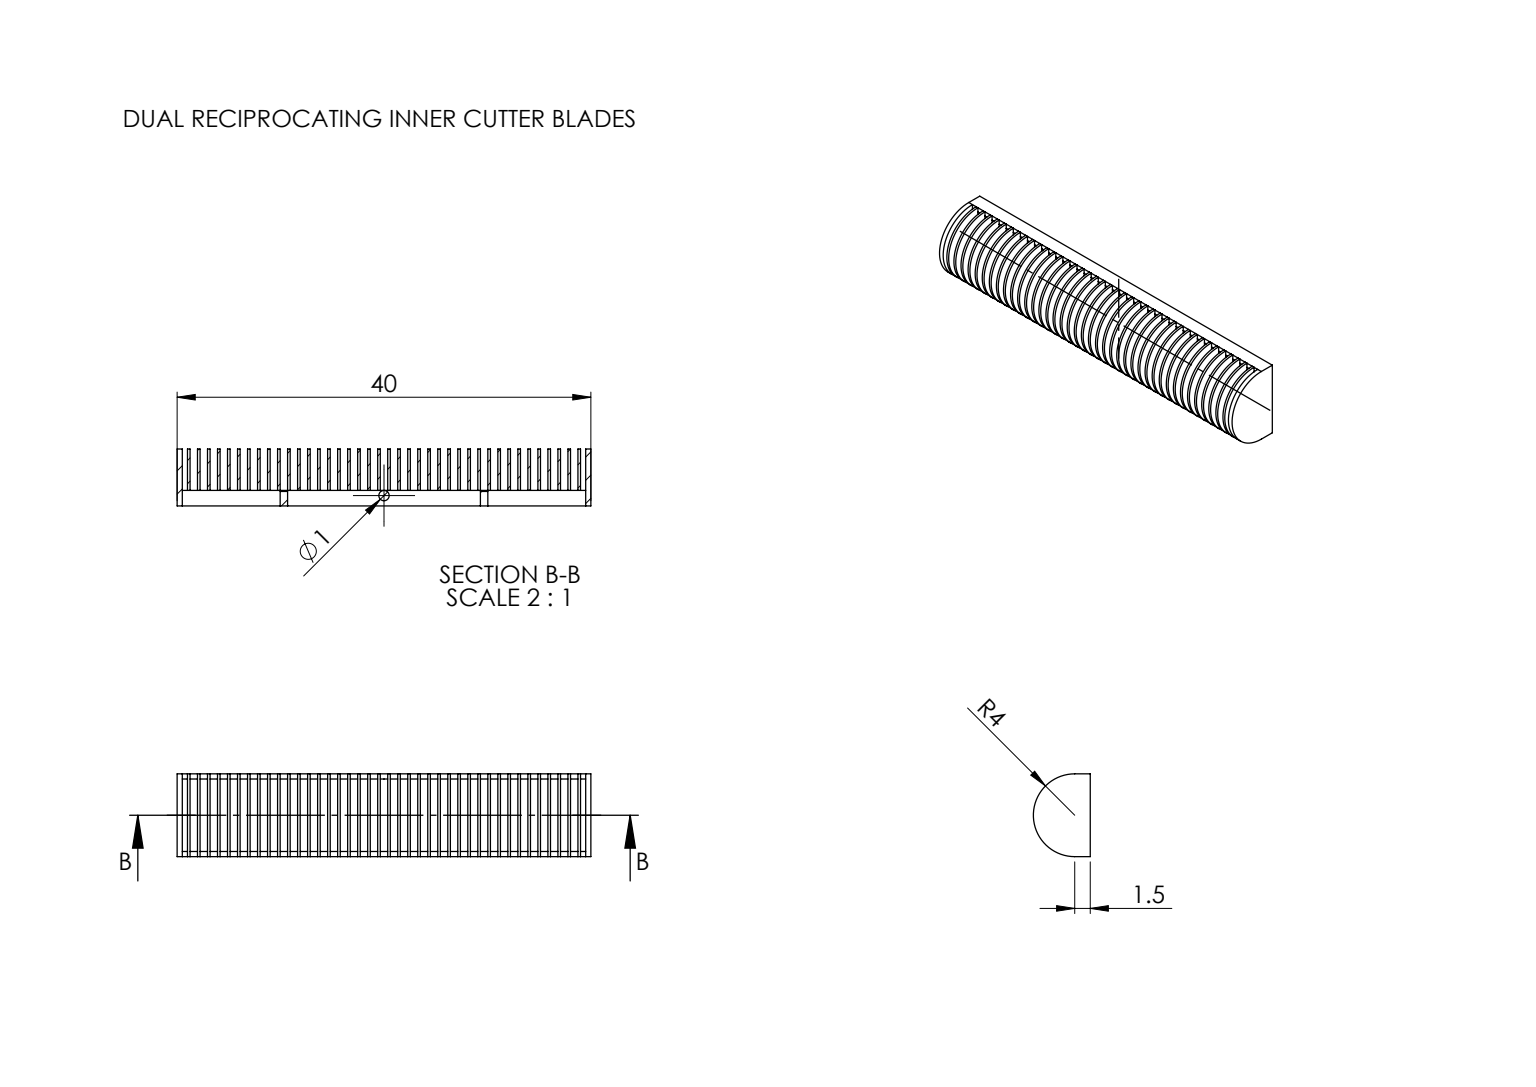
ISO-10303-21;
HEADER;
FILE_DESCRIPTION (('STEP AP214'),
    '1' );
FILE_NAME ('Dual Reciprocating Inner Cutter Blades.step',
    '2026-10-05T05:16:24',
    ( '' ),
    ( '' ),
    'SwSTEP 2.0',
    'SolidWorks 2026',
    '' );
FILE_SCHEMA (( 'AUTOMOTIVE_DESIGN' ));
ENDSEC;

DATA;
#43=ORIENTED_EDGE ( 'NONE', *, *, #10350, .F. ) ;
#63=CARTESIAN_POINT ( 'NONE',  ( -10.28846153846153832, -7.500000000000000000, 29.75000000000000355 ) ) ;
#66=ORIENTED_EDGE ( 'NONE', *, *, #42296, .F. ) ;
#80=EDGE_CURVE ( 'NONE', #19996, #25471, #12251, .T. ) ;
#85=CARTESIAN_POINT ( 'NONE',  ( -6.416666666666667851, -7.500000000000000000, 33.75000000000000000 ) ) ;
#89=ORIENTED_EDGE ( 'NONE', *, *, #31781, .F. ) ;
#103=EDGE_CURVE ( 'NONE', #84442, #3259, #72212, .T. ) ;
#104=VECTOR ( 'NONE', #2101, 1000.000000000000000 ) ;
#130=DIRECTION ( 'NONE',  ( -0.000000000000000000, 1.000000000000000000, -0.000000000000000000 ) ) ;
#140=CIRCLE ( 'NONE', #14540, 4.000000000000000000 ) ;
#156=CARTESIAN_POINT ( 'NONE',  ( 0.000000000000000000, -4.000000000000000000, 29.65000000000000213 ) ) ;
#169=ORIENTED_EDGE ( 'NONE', *, *, #57936, .F. ) ;
#181=ADVANCED_FACE ( 'NONE', ( #62640 ), #1839, .F. ) ;
#187=DIRECTION ( 'NONE',  ( -1.000000000000000000, -0.000000000000000000, -0.000000000000000000 ) ) ;
#201=EDGE_CURVE ( 'NONE', #75095, #37056, #56777, .T. ) ;
#227=DIRECTION ( 'NONE',  ( 1.000000000000000000, 0.000000000000000000, 0.000000000000000000 ) ) ;
#231=ORIENTED_EDGE ( 'NONE', *, *, #20585, .T. ) ;
#235=VERTEX_POINT ( 'NONE', #52679 ) ;
#282=EDGE_CURVE ( 'NONE', #18719, #16151, #10625, .T. ) ;
#284=CARTESIAN_POINT ( 'NONE',  ( -19.50000000000000000, -3.499999999999999556, 29.75000000000000355 ) ) ;
#286=CARTESIAN_POINT ( 'NONE',  ( 20.00000000000000000, -4.000000000000000000, 29.75000000000000355 ) ) ;
#293=DIRECTION ( 'NONE',  ( 0.000000000000000000, 0.000000000000000000, -1.000000000000000000 ) ) ;
#298=VECTOR ( 'NONE', #58906, 1000.000000000000000 ) ;
#299=ORIENTED_EDGE ( 'NONE', *, *, #31219, .F. ) ;
#325=VECTOR ( 'NONE', #40257, 1000.000000000000000 ) ;
#332=VECTOR ( 'NONE', #25563, 1000.000000000000000 ) ;
#345=VERTEX_POINT ( 'NONE', #74747 ) ;
#351=DIRECTION ( 'NONE',  ( -1.000000000000000000, -0.000000000000000000, -0.000000000000000000 ) ) ;
#357=FACE_OUTER_BOUND ( 'NONE', #7317, .T. ) ;
#362=CARTESIAN_POINT ( 'NONE',  ( 5.198717948717946236, -4.000000000000000000, 29.75000000000000355 ) ) ;
#377=ADVANCED_FACE ( 'NONE', ( #29653 ), #76057, .T. ) ;
#393=EDGE_CURVE ( 'NONE', #23382, #20924, #8053, .T. ) ;
#417=DIRECTION ( 'NONE',  ( 1.000000000000000000, 0.000000000000000000, 0.000000000000000000 ) ) ;
#418=CARTESIAN_POINT ( 'NONE',  ( -16.81410256410256565, -11.50000000000000000, 29.75000000000000355 ) ) ;
#426=COLOUR_RGB ( '', 0.72549020, 0.75294118, 0.79215686) ;
#427=VERTEX_POINT ( 'NONE', #8497 ) ;
#455=LINE ( 'NONE', #48625, #11505 ) ;
#469=CARTESIAN_POINT ( 'NONE',  ( 8.102564102564102200, -11.00000000000000000, 29.75000000000000355 ) ) ;
#496=VERTEX_POINT ( 'NONE', #69311 ) ;
#498=FACE_OUTER_BOUND ( 'NONE', #59189, .T. ) ;
#499=EDGE_LOOP ( 'NONE', ( #8065, #69891, #54153, #58268 ) ) ;
#505=ADVANCED_FACE ( 'NONE', ( #65191 ), #59330, .F. ) ;
#525=AXIS2_PLACEMENT_3D ( 'NONE', #7311, #6858, #76199 ) ;
#528=CARTESIAN_POINT ( 'NONE',  ( -3.262820512820514107, -7.500000000000000000, 29.75000000000000355 ) ) ;
#532=ORIENTED_EDGE ( 'NONE', *, *, #45439, .F. ) ;
#537=LINE ( 'NONE', #63557, #72302 ) ;
#544=CIRCLE ( 'NONE', #45150, 4.000000000000000000 ) ;
#548=DIRECTION ( 'NONE',  ( -0.000000000000000000, 1.000000000000000000, -0.000000000000000000 ) ) ;
#550=VECTOR ( 'NONE', #21356, 1000.000000000000000 ) ;
#573=CARTESIAN_POINT ( 'NONE',  ( 20.00000000000000000, -4.000000000000000000, 29.75000000000000355 ) ) ;
#598=DIRECTION ( 'NONE',  ( 0.000000000000000000, -0.000000000000000000, 1.000000000000000000 ) ) ;
#619=ORIENTED_EDGE ( 'NONE', *, *, #51470, .F. ) ;
#634=DIRECTION ( 'NONE',  ( 1.000000000000000000, 0.000000000000000000, 0.000000000000000000 ) ) ;
#641=CARTESIAN_POINT ( 'NONE',  ( 20.00000000000000000, -4.000000000000000000, 29.75000000000000355 ) ) ;
#681=ORIENTED_EDGE ( 'NONE', *, *, #24672, .T. ) ;
#686=DIRECTION ( 'NONE',  ( -0.000000000000000000, 1.000000000000000000, -0.000000000000000000 ) ) ;
#691=PLANE ( 'NONE',  #60122 ) ;
#695=VECTOR ( 'NONE', #44680, 1000.000000000000000 ) ;
#706=CARTESIAN_POINT ( 'NONE',  ( 3.512820512820510555, -3.499999999999999556, 29.75000000000000355 ) ) ;
#723=DIRECTION ( 'NONE',  ( 1.000000000000000000, 0.000000000000000000, 0.000000000000000000 ) ) ;
#756=LINE ( 'NONE', #28222, #84616 ) ;
#774=ORIENTED_EDGE ( 'NONE', *, *, #775, .F. ) ;
#775=EDGE_CURVE ( 'NONE', #46484, #84195, #71288, .T. ) ;
#780=ORIENTED_EDGE ( 'NONE', *, *, #80659, .F. ) ;
#792=CARTESIAN_POINT ( 'NONE',  ( -18.75000000000000000, -4.000000000000000000, 29.75000000000000355 ) ) ;
#811=DIRECTION ( 'NONE',  ( 1.000000000000000000, 0.000000000000000000, 0.000000000000000000 ) ) ;
#823=EDGE_CURVE ( 'NONE', #22055, #5633, #71733, .T. ) ;
#832=CARTESIAN_POINT ( 'NONE',  ( 16.81410256410256565, -3.499999999999999556, 29.75000000000000355 ) ) ;
#838=CARTESIAN_POINT ( 'NONE',  ( -17.78205128205128105, -3.499999999999999556, 29.75000000000000355 ) ) ;
#851=CARTESIAN_POINT ( 'NONE',  ( 20.00000000000000000, -3.499999999999999556, 29.75000000000000355 ) ) ;
#856=VERTEX_POINT ( 'NONE', #42182 ) ;
#857=LINE ( 'NONE', #49041, #17570 ) ;
#859=LINE ( 'NONE', #33327, #83953 ) ;
#860=LINE ( 'NONE', #69327, #48492 ) ;
#866=EDGE_CURVE ( 'NONE', #87922, #72293, #29882, .T. ) ;
#882=VECTOR ( 'NONE', #7598, 1000.000000000000000 ) ;
#885=ORIENTED_EDGE ( 'NONE', *, *, #13025, .T. ) ;
#909=CARTESIAN_POINT ( 'NONE',  ( -5.198717948717948012, -7.500000000000000000, 33.75000000000000000 ) ) ;
#923=ADVANCED_BREP_SHAPE_REPRESENTATION ( '', ( #28293, #83448 ), #70522 ) ;
#938=DIRECTION ( 'NONE',  ( 0.000000000000000000, 0.000000000000000000, -1.000000000000000000 ) ) ;
#940=CYLINDRICAL_SURFACE ( 'NONE', #5295, 4.000000000000000000 ) ;
#949=VERTEX_POINT ( 'NONE', #24881 ) ;
#955=VERTEX_POINT ( 'NONE', #59557 ) ;
#959=AXIS2_PLACEMENT_3D ( 'NONE', #1082, #49271, #73543 ) ;
#965=VECTOR ( 'NONE', #65719, 1000.000000000000000 ) ;
#972=DIRECTION ( 'NONE',  ( -0.000000000000000000, 1.000000000000000000, -0.000000000000000000 ) ) ;
#981=CARTESIAN_POINT ( 'NONE',  ( -10.03846153846153832, -4.000000000000000000, 29.25000000000000000 ) ) ;
#985=ORIENTED_EDGE ( 'NONE', *, *, #59724, .T. ) ;
#987=EDGE_LOOP ( 'NONE', ( #37352, #22515, #57564, #42926 ) ) ;
#992=VECTOR ( 'NONE', #4402, 1000.000000000000000 ) ;
#993=FACE_OUTER_BOUND ( 'NONE', #69056, .T. ) ;
#1006=CARTESIAN_POINT ( 'NONE',  ( -4.480769230769229061, -4.000000000000000000, 29.75000000000000355 ) ) ;
#1012=VERTEX_POINT ( 'NONE', #48701 ) ;
#1029=ORIENTED_EDGE ( 'NONE', *, *, #8831, .T. ) ;
#1031=ADVANCED_FACE ( 'NONE', ( #5959 ), #53690, .T. ) ;
#1036=DIRECTION ( 'NONE',  ( 0.000000000000000000, 0.000000000000000000, -1.000000000000000000 ) ) ;
#1051=VECTOR ( 'NONE', #75352, 1000.000000000000000 ) ;
#1057=EDGE_LOOP ( 'NONE', ( #1568, #37917, #18646, #65919 ) ) ;
#1082=CARTESIAN_POINT ( 'NONE',  ( -16.81410256410256565, -7.500000000000000000, 29.75000000000000355 ) ) ;
#1092=ORIENTED_EDGE ( 'NONE', *, *, #823, .F. ) ;
#1103=EDGE_CURVE ( 'NONE', #81224, #48029, #68558, .T. ) ;
#1133=DIRECTION ( 'NONE',  ( 0.000000000000000000, 0.000000000000000000, 1.000000000000000000 ) ) ;
#1148=VECTOR ( 'NONE', #38524, 1000.000000000000000 ) ;
#1206=ORIENTED_EDGE ( 'NONE', *, *, #30331, .F. ) ;
#1231=DIRECTION ( 'NONE',  ( 0.000000000000000000, 0.000000000000000000, -1.000000000000000000 ) ) ;
#1250=CARTESIAN_POINT ( 'NONE',  ( 20.00000000000000000, -4.000000000000000000, 29.75000000000000355 ) ) ;
#1268=CARTESIAN_POINT ( 'NONE',  ( 6.416666666666664298, -11.50000000000000000, 29.75000000000000355 ) ) ;
#1284=ORIENTED_EDGE ( 'NONE', *, *, #40773, .F. ) ;
#1327=AXIS2_PLACEMENT_3D ( 'NONE', #67691, #28352, #40223 ) ;
#1331=AXIS2_PLACEMENT_3D ( 'NONE', #28757, #51198, #49466 ) ;
#1333=VERTEX_POINT ( 'NONE', #30644 ) ;
#1374=FACE_OUTER_BOUND ( 'NONE', #33214, .T. ) ;
#1386=PLANE ( 'NONE',  #17654 ) ;
#1393=AXIS2_PLACEMENT_3D ( 'NONE', #18730, #59256, #59702 ) ;
#1395=DIRECTION ( 'NONE',  ( 1.000000000000000000, 0.000000000000000000, 0.000000000000000000 ) ) ;
#1397=DIRECTION ( 'NONE',  ( -1.000000000000000000, -0.000000000000000000, 0.000000000000000000 ) ) ;
#1401=VECTOR ( 'NONE', #24481, 1000.000000000000000 ) ;
#1405=AXIS2_PLACEMENT_3D ( 'NONE', #11950, #31322, #53361 ) ;
#1406=ORIENTED_EDGE ( 'NONE', *, *, #78616, .F. ) ;
#1415=CARTESIAN_POINT ( 'NONE',  ( -0.6089743589743593644, -3.499999999999999556, 29.75000000000000355 ) ) ;
#1428=ORIENTED_EDGE ( 'NONE', *, *, #57736, .F. ) ;
#1434=EDGE_CURVE ( 'NONE', #50542, #83291, #88729, .T. ) ;
#1450=AXIS2_PLACEMENT_3D ( 'NONE', #52880, #24518, #79482 ) ;
#1456=ORIENTED_EDGE ( 'NONE', *, *, #88867, .T. ) ;
#1473=ORIENTED_EDGE ( 'NONE', *, *, #63442, .F. ) ;
#1490=CARTESIAN_POINT ( 'NONE',  ( -18.03205128205128105, -3.499999999999999556, 29.75000000000000355 ) ) ;
#1493=VERTEX_POINT ( 'NONE', #21123 ) ;
#1495=DIRECTION ( 'NONE',  ( -1.000000000000000000, -0.000000000000000000, -0.000000000000000000 ) ) ;
#1501=ADVANCED_FACE ( 'NONE', ( #63440 ), #77841, .F. ) ;
#1503=VECTOR ( 'NONE', #30513, 1000.000000000000000 ) ;
#1506=FACE_OUTER_BOUND ( 'NONE', #62728, .T. ) ;
#1517=EDGE_CURVE ( 'NONE', #55049, #67618, #860, .T. ) ;
#1526=ORIENTED_EDGE ( 'NONE', *, *, #34553, .F. ) ;
#1553=EDGE_CURVE ( 'NONE', #78266, #17849, #49497, .T. ) ;
#1559=ORIENTED_EDGE ( 'NONE', *, *, #71272, .T. ) ;
#1565=DIRECTION ( 'NONE',  ( 0.000000000000000000, 0.000000000000000000, -1.000000000000000000 ) ) ;
#1568=ORIENTED_EDGE ( 'NONE', *, *, #54155, .F. ) ;
#1572=EDGE_CURVE ( 'NONE', #20924, #27696, #5306, .T. ) ;
#1576=VECTOR ( 'NONE', #71122, 1000.000000000000000 ) ;
#1582=DIRECTION ( 'NONE',  ( -1.000000000000000000, -0.000000000000000000, -0.000000000000000000 ) ) ;
#1583=DIRECTION ( 'NONE',  ( 0.000000000000000000, 0.000000000000000000, -1.000000000000000000 ) ) ;
#1584=DIRECTION ( 'NONE',  ( -0.000000000000000000, 0.000000000000000000, 1.000000000000000000 ) ) ;
#1587=VECTOR ( 'NONE', #24500, 1000.000000000000000 ) ;
#1614=EDGE_CURVE ( 'NONE', #32479, #19139, #52139, .T. ) ;
#1627=VECTOR ( 'NONE', #61858, 1000.000000000000000 ) ;
#1652=VERTEX_POINT ( 'NONE', #78732 ) ;
#1654=ORIENTED_EDGE ( 'NONE', *, *, #27147, .T. ) ;
#1664=ORIENTED_EDGE ( 'NONE', *, *, #70919, .F. ) ;
#1669=DIRECTION ( 'NONE',  ( 1.000000000000000000, 0.000000000000000000, 0.000000000000000000 ) ) ;
#1679=EDGE_CURVE ( 'NONE', #34673, #24943, #58899, .T. ) ;
#1682=CARTESIAN_POINT ( 'NONE',  ( -2.294871794871794712, -11.00000000000000000, 29.75000000000000355 ) ) ;
#1708=ORIENTED_EDGE ( 'NONE', *, *, #14428, .T. ) ;
#1731=CARTESIAN_POINT ( 'NONE',  ( 14.16025641025641235, -3.499999999999999556, 29.75000000000000355 ) ) ;
#1733=DIRECTION ( 'NONE',  ( 0.000000000000000000, 0.000000000000000000, -1.000000000000000000 ) ) ;
#1734=FACE_OUTER_BOUND ( 'NONE', #71110, .T. ) ;
#1747=ORIENTED_EDGE ( 'NONE', *, *, #24136, .F. ) ;
#1752=PLANE ( 'NONE',  #35748 ) ;
#1759=CARTESIAN_POINT ( 'NONE',  ( 18.75000000000000000, -4.000000000000000000, 29.75000000000000355 ) ) ;
#1774=PLANE ( 'NONE',  #72639 ) ;
#1775=ORIENTED_EDGE ( 'NONE', *, *, #3712, .T. ) ;
#1813=DIRECTION ( 'NONE',  ( -0.000000000000000000, 1.000000000000000000, -0.000000000000000000 ) ) ;
#1829=EDGE_CURVE ( 'NONE', #64127, #48416, #12500, .T. ) ;
#1832=DIRECTION ( 'NONE',  ( -1.000000000000000000, -0.000000000000000000, -0.000000000000000000 ) ) ;
#1839=PLANE ( 'NONE',  #51896 ) ;
#1856=LINE ( 'NONE', #63987, #27063 ) ;
#1861=DIRECTION ( 'NONE',  ( -0.000000000000000000, 1.000000000000000000, -0.000000000000000000 ) ) ;
#1863=VECTOR ( 'NONE', #23258, 1000.000000000000000 ) ;
#1865=CARTESIAN_POINT ( 'NONE',  ( -13.91025641025641058, -11.50000000000000000, 29.75000000000000355 ) ) ;
#1877=ADVANCED_FACE ( 'NONE', ( #25410 ), #51976, .F. ) ;
#1878=VERTEX_POINT ( 'NONE', #66841 ) ;
#1892=DIRECTION ( 'NONE',  ( -1.000000000000000000, 0.000000000000000000, -0.000000000000000000 ) ) ;
#1898=CARTESIAN_POINT ( 'NONE',  ( -3.262820512820514107, -7.500000000000000000, 33.75000000000000000 ) ) ;
#1908=ADVANCED_FACE ( 'NONE', ( #60074 ), #86239, .F. ) ;
#1926=VECTOR ( 'NONE', #72975, 1000.000000000000000 ) ;
#1944=DIRECTION ( 'NONE',  ( -1.000000000000000000, 0.000000000000000000, -0.000000000000000000 ) ) ;
#1957=CARTESIAN_POINT ( 'NONE',  ( 7.384615384615385025, -3.499999999999999556, 29.75000000000000355 ) ) ;
#1964=CIRCLE ( 'NONE', #52285, 4.000000000000000000 ) ;
#1970=EDGE_CURVE ( 'NONE', #30104, #87793, #20865, .T. ) ;
#1972=EDGE_LOOP ( 'NONE', ( #51803, #60788, #41402, #7362 ) ) ;
#1980=EDGE_CURVE ( 'NONE', #55785, #38648, #82590, .T. ) ;
#1992=ORIENTED_EDGE ( 'NONE', *, *, #87731, .T. ) ;
#2027=CARTESIAN_POINT ( 'NONE',  ( -5.198717948717948012, -7.500000000000000000, 33.75000000000000000 ) ) ;
#2070=CARTESIAN_POINT ( 'NONE',  ( -19.50000000000000000, -3.499999999999999556, 29.75000000000000355 ) ) ;
#2085=VERTEX_POINT ( 'NONE', #74740 ) ;
#2092=CARTESIAN_POINT ( 'NONE',  ( -19.00000000000000000, -7.500000000000000000, 29.75000000000000355 ) ) ;
#2095=ORIENTED_EDGE ( 'NONE', *, *, #39042, .F. ) ;
#2101=DIRECTION ( 'NONE',  ( -1.000000000000000000, -0.000000000000000000, 0.000000000000000000 ) ) ;
#2116=CARTESIAN_POINT ( 'NONE',  ( 0.3589743589743582541, -7.500000000000000000, 29.75000000000000355 ) ) ;
#2121=CARTESIAN_POINT ( 'NONE',  ( 20.00000000000000000, -4.000000000000000000, 29.75000000000000355 ) ) ;
#2125=ORIENTED_EDGE ( 'NONE', *, *, #16712, .F. ) ;
#2144=FACE_OUTER_BOUND ( 'NONE', #19220, .T. ) ;
#2160=ORIENTED_EDGE ( 'NONE', *, *, #26803, .T. ) ;
#2174=VECTOR ( 'NONE', #49018, 1000.000000000000000 ) ;
#2177=ORIENTED_EDGE ( 'NONE', *, *, #59364, .T. ) ;
#2183=ORIENTED_EDGE ( 'NONE', *, *, #14015, .F. ) ;
#2191=ADVANCED_FACE ( 'NONE', ( #48569 ), #76050, .F. ) ;
#2194=ORIENTED_EDGE ( 'NONE', *, *, #21005, .T. ) ;
#2199=AXIS2_PLACEMENT_3D ( 'NONE', #14959, #44167, #77095 ) ;
#2212=CARTESIAN_POINT ( 'NONE',  ( -18.75000000000000000, -11.50000000000000000, 29.75000000000000355 ) ) ;
#2225=LINE ( 'NONE', #55849, #67827 ) ;
#2235=CARTESIAN_POINT ( 'NONE',  ( 20.00000000000000000, -4.000000000000000000, 29.75000000000000355 ) ) ;
#2237=EDGE_LOOP ( 'NONE', ( #84036, #26205, #82453, #32891, #73664 ) ) ;
#2248=CARTESIAN_POINT ( 'NONE',  ( 1.326923076923075762, -11.00000000000000000, 29.75000000000000355 ) ) ;
#2256=AXIS2_PLACEMENT_3D ( 'NONE', #9773, #56636, #71466 ) ;
#2258=FACE_OUTER_BOUND ( 'NONE', #13603, .T. ) ;
#2269=CIRCLE ( 'NONE', #6595, 4.000000000000000000 ) ;
#2279=ORIENTED_EDGE ( 'NONE', *, *, #42735, .T. ) ;
#2287=EDGE_CURVE ( 'NONE', #23070, #235, #14045, .T. ) ;
#2291=VECTOR ( 'NONE', #33549, 1000.000000000000000 ) ;
#2293=LINE ( 'NONE', #22141, #25357 ) ;
#2307=ORIENTED_EDGE ( 'NONE', *, *, #76762, .T. ) ;
#2311=DIRECTION ( 'NONE',  ( -0.000000000000000000, 1.000000000000000000, -0.000000000000000000 ) ) ;
#2319=ADVANCED_FACE ( 'NONE', ( #77380 ), #23751, .F. ) ;
#2322=ORIENTED_EDGE ( 'NONE', *, *, #44361, .F. ) ;
#2351=EDGE_LOOP ( 'NONE', ( #79932, #72056, #42009, #57754 ) ) ;
#2360=EDGE_CURVE ( 'NONE', #29827, #86419, #51204, .T. ) ;
#2362=CYLINDRICAL_SURFACE ( 'NONE', #36184, 4.000000000000000000 ) ;
#2382=CIRCLE ( 'NONE', #15324, 4.000000000000000000 ) ;
#2392=VERTEX_POINT ( 'NONE', #78711 ) ;
#2421=VECTOR ( 'NONE', #3040, 1000.000000000000000 ) ;
#2425=EDGE_CURVE ( 'NONE', #48052, #5633, #24651, .T. ) ;
#2432=ORIENTED_EDGE ( 'NONE', *, *, #24288, .T. ) ;
#2434=ORIENTED_EDGE ( 'NONE', *, *, #22837, .T. ) ;
#2437=VECTOR ( 'NONE', #87966, 1000.000000000000000 ) ;
#2441=ORIENTED_EDGE ( 'NONE', *, *, #7391, .T. ) ;
#2448=EDGE_CURVE ( 'NONE', #6548, #11602, #73751, .T. ) ;
#2467=DIRECTION ( 'NONE',  ( 1.000000000000000000, 0.000000000000000000, 0.000000000000000000 ) ) ;
#2502=EDGE_CURVE ( 'NONE', #24740, #74652, #52560, .T. ) ;
#2512=CARTESIAN_POINT ( 'NONE',  ( -13.91025641025641058, -3.499999999999999556, 29.75000000000000355 ) ) ;
#2513=AXIS2_PLACEMENT_3D ( 'NONE', #838, #35064, #62095 ) ;
#2519=ORIENTED_EDGE ( 'NONE', *, *, #20527, .F. ) ;
#2528=DIRECTION ( 'NONE',  ( 0.000000000000000000, 0.000000000000000000, 1.000000000000000000 ) ) ;
#2530=ORIENTED_EDGE ( 'NONE', *, *, #33972, .F. ) ;
#2538=CARTESIAN_POINT ( 'NONE',  ( -19.50000000000000000, -11.50000000000000000, 29.75000000000000355 ) ) ;
#2571=LINE ( 'NONE', #30063, #7312 ) ;
#2576=ADVANCED_FACE ( 'NONE', ( #36202 ), #69525, .F. ) ;
#2579=CARTESIAN_POINT ( 'NONE',  ( 12.94230769230769340, -3.499999999999999556, 29.75000000000000355 ) ) ;
#2608=EDGE_CURVE ( 'NONE', #80662, #81634, #61100, .T. ) ;
#2616=CIRCLE ( 'NONE', #27123, 4.000000000000000000 ) ;
#2620=ADVANCED_FACE ( 'NONE', ( #9587 ), #58213, .F. ) ;
#2623=FACE_OUTER_BOUND ( 'NONE', #72608, .T. ) ;
#2631=EDGE_CURVE ( 'NONE', #35283, #64127, #30743, .T. ) ;
#2662=AXIS2_PLACEMENT_3D ( 'NONE', #67394, #47108, #27293 ) ;
#2667=ORIENTED_EDGE ( 'NONE', *, *, #61590, .F. ) ;
#2668=DIRECTION ( 'NONE',  ( 0.000000000000000000, 1.000000000000000000, 0.000000000000000000 ) ) ;
#2672=LINE ( 'NONE', #2235, #40622 ) ;
#2678=ORIENTED_EDGE ( 'NONE', *, *, #36115, .T. ) ;
#2680=EDGE_CURVE ( 'NONE', #74021, #13621, #37497, .T. ) ;
#2716=EDGE_CURVE ( 'NONE', #53841, #77088, #5511, .T. ) ;
#2724=ORIENTED_EDGE ( 'NONE', *, *, #51536, .T. ) ;
#2725=VECTOR ( 'NONE', #47467, 1000.000000000000000 ) ;
#2742=ORIENTED_EDGE ( 'NONE', *, *, #79560, .T. ) ;
#2763=DIRECTION ( 'NONE',  ( -1.000000000000000000, -0.000000000000000000, -0.000000000000000000 ) ) ;
#2781=VECTOR ( 'NONE', #43857, 1000.000000000000000 ) ;
#2792=VECTOR ( 'NONE', #5260, 1000.000000000000000 ) ;
#2796=AXIS2_PLACEMENT_3D ( 'NONE', #85379, #21900, #44364 ) ;
#2827=VECTOR ( 'NONE', #8252, 1000.000000000000000 ) ;
#2828=ORIENTED_EDGE ( 'NONE', *, *, #53808, .F. ) ;
#2843=VERTEX_POINT ( 'NONE', #20356 ) ;
#2852=VECTOR ( 'NONE', #1832, 1000.000000000000000 ) ;
#2853=CIRCLE ( 'NONE', #11558, 4.000000000000000000 ) ;
#2855=ORIENTED_EDGE ( 'NONE', *, *, #6324, .T. ) ;
#2867=EDGE_CURVE ( 'NONE', #38648, #58158, #59998, .T. ) ;
#2869=CARTESIAN_POINT ( 'NONE',  ( 17.78205128205128105, -3.499999999999999556, 29.75000000000000355 ) ) ;
#2890=EDGE_CURVE ( 'NONE', #10355, #2843, #41066, .T. ) ;
#2904=EDGE_CURVE ( 'NONE', #35531, #86970, #68527, .T. ) ;
#2908=DIRECTION ( 'NONE',  ( 0.000000000000000000, 0.000000000000000000, -1.000000000000000000 ) ) ;
#2913=VECTOR ( 'NONE', #79043, 1000.000000000000000 ) ;
#2915=ADVANCED_FACE ( 'NONE', ( #46489 ), #73967, .F. ) ;
#2928=AXIS2_PLACEMENT_3D ( 'NONE', #34029, #20950, #48421 ) ;
#2966=VECTOR ( 'NONE', #38248, 1000.000000000000000 ) ;
#2972=AXIS2_PLACEMENT_3D ( 'NONE', #41805, #26956, #54413 ) ;
#2979=VECTOR ( 'NONE', #40702, 1000.000000000000000 ) ;
#3004=CARTESIAN_POINT ( 'NONE',  ( 5.448717948717947124, -7.500000000000000000, 29.75000000000000355 ) ) ;
#3029=CARTESIAN_POINT ( 'NONE',  ( 18.03205128205128105, -11.00000000000000000, 29.75000000000000355 ) ) ;
#3040=DIRECTION ( 'NONE',  ( -1.000000000000000000, -0.000000000000000000, -0.000000000000000000 ) ) ;
#3044=VECTOR ( 'NONE', #84328, 1000.000000000000000 ) ;
#3048=DIRECTION ( 'NONE',  ( 1.000000000000000000, 0.000000000000000000, 0.000000000000000000 ) ) ;
#3060=CARTESIAN_POINT ( 'NONE',  ( -19.50000000000000000, -3.499999999999999556, 29.75000000000000355 ) ) ;
#3074=ORIENTED_EDGE ( 'NONE', *, *, #10327, .F. ) ;
#3077=AXIS2_PLACEMENT_3D ( 'NONE', #88927, #42055, #49246 ) ;
#3084=EDGE_CURVE ( 'NONE', #22055, #74851, #83095, .T. ) ;
#3089=CARTESIAN_POINT ( 'NONE',  ( -10.03846153846153832, -3.499999999999999556, 29.75000000000000355 ) ) ;
#3091=ORIENTED_EDGE ( 'NONE', *, *, #14653, .T. ) ;
#3093=CARTESIAN_POINT ( 'NONE',  ( -8.102564102564102200, -7.500000000000000000, 29.75000000000000355 ) ) ;
#3095=CARTESIAN_POINT ( 'NONE',  ( 16.09615384615384670, -3.499999999999999556, 29.75000000000000355 ) ) ;
#3099=VECTOR ( 'NONE', #55182, 1000.000000000000000 ) ;
#3102=LINE ( 'NONE', #10760, #1576 ) ;
#3118=CARTESIAN_POINT ( 'NONE',  ( -11.97435897435897267, -7.500000000000000000, 29.75000000000000355 ) ) ;
#3122=DIRECTION ( 'NONE',  ( 0.000000000000000000, 0.000000000000000000, -1.000000000000000000 ) ) ;
#3128=ORIENTED_EDGE ( 'NONE', *, *, #73177, .F. ) ;
#3154=EDGE_CURVE ( 'NONE', #43102, #76951, #87849, .T. ) ;
#3185=CIRCLE ( 'NONE', #19071, 4.000000000000000000 ) ;
#3188=LINE ( 'NONE', #65770, #78107 ) ;
#3195=ADVANCED_FACE ( 'NONE', ( #14824 ), #68425, .F. ) ;
#3208=VECTOR ( 'NONE', #88293, 1000.000000000000000 ) ;
#3212=CARTESIAN_POINT ( 'NONE',  ( -11.25641025641025550, -3.499999999999999556, 29.75000000000000355 ) ) ;
#3215=CARTESIAN_POINT ( 'NONE',  ( -19.50000000000000000, -3.499999999999999556, 29.75000000000000355 ) ) ;
#3235=ADVANCED_FACE ( 'NONE', ( #56246 ), #62541, .F. ) ;
#3251=ORIENTED_EDGE ( 'NONE', *, *, #79029, .T. ) ;
#3259=VERTEX_POINT ( 'NONE', #7619 ) ;
#3262=VERTEX_POINT ( 'NONE', #418 ) ;
#3275=DIRECTION ( 'NONE',  ( 0.000000000000000000, 0.000000000000000000, -1.000000000000000000 ) ) ;
#3292=VERTEX_POINT ( 'NONE', #27887 ) ;
#3294=ORIENTED_EDGE ( 'NONE', *, *, #55497, .F. ) ;
#3296=CIRCLE ( 'NONE', #66576, 4.000000000000000000 ) ;
#3302=EDGE_CURVE ( 'NONE', #5633, #496, #34222, .T. ) ;
#3303=FACE_OUTER_BOUND ( 'NONE', #83869, .T. ) ;
#3310=EDGE_LOOP ( 'NONE', ( #83643, #82972, #52409, #33244, #73566 ) ) ;
#3332=EDGE_CURVE ( 'NONE', #37853, #58001, #85933, .T. ) ;
#3340=DIRECTION ( 'NONE',  ( 0.000000000000000000, 0.000000000000000000, 1.000000000000000000 ) ) ;
#3356=CARTESIAN_POINT ( 'NONE',  ( 9.070512820512819374, -3.499999999999999556, 29.75000000000000355 ) ) ;
#3398=EDGE_CURVE ( 'NONE', #3876, #58816, #16576, .T. ) ;
#3414=VECTOR ( 'NONE', #68678, 1000.000000000000000 ) ;
#3438=ORIENTED_EDGE ( 'NONE', *, *, #30030, .T. ) ;
#3448=EDGE_CURVE ( 'NONE', #76927, #73366, #25114, .T. ) ;
#3488=AXIS2_PLACEMENT_3D ( 'NONE', #63887, #16156, #15722 ) ;
#3489=VECTOR ( 'NONE', #65292, 1000.000000000000000 ) ;
#3492=ORIENTED_EDGE ( 'NONE', *, *, #69496, .F. ) ;
#3497=CARTESIAN_POINT ( 'NONE',  ( -3.262820512820514107, -7.500000000000000000, 29.75000000000000355 ) ) ;
#3519=ORIENTED_EDGE ( 'NONE', *, *, #19505, .T. ) ;
#3529=VERTEX_POINT ( 'NONE', #52133 ) ;
#3563=DIRECTION ( 'NONE',  ( 0.000000000000000000, 0.000000000000000000, -1.000000000000000000 ) ) ;
#3593=DIRECTION ( 'NONE',  ( 0.000000000000000000, 0.000000000000000000, 1.000000000000000000 ) ) ;
#3624=VECTOR ( 'NONE', #69672, 1000.000000000000000 ) ;
#3628=CARTESIAN_POINT ( 'NONE',  ( 11.97435897435897623, -11.50000000000000000, 29.75000000000000355 ) ) ;
#3629=CARTESIAN_POINT ( 'NONE',  ( 20.00000000000000000, -4.000000000000000000, 29.75000000000000355 ) ) ;
#3633=VERTEX_POINT ( 'NONE', #7952 ) ;
#3634=CARTESIAN_POINT ( 'NONE',  ( -19.50000000000000000, -7.500000000000000000, 33.75000000000000000 ) ) ;
#3638=ORIENTED_EDGE ( 'NONE', *, *, #21291, .T. ) ;
#3647=EDGE_LOOP ( 'NONE', ( #62792, #87525, #25905, #75128, #60301 ) ) ;
#3664=CARTESIAN_POINT ( 'NONE',  ( -1.326923076923076872, -3.499999999999999556, 29.75000000000000355 ) ) ;
#3692=DIRECTION ( 'NONE',  ( 0.000000000000000000, 0.000000000000000000, -1.000000000000000000 ) ) ;
#3698=ORIENTED_EDGE ( 'NONE', *, *, #27739, .F. ) ;
#3701=CARTESIAN_POINT ( 'NONE',  ( 8.102564102564102200, -7.500000000000000000, 29.75000000000000355 ) ) ;
#3712=EDGE_CURVE ( 'NONE', #48041, #62888, #16477, .T. ) ;
#3724=ORIENTED_EDGE ( 'NONE', *, *, #22949, .T. ) ;
#3750=LINE ( 'NONE', #73105, #68099 ) ;
#3756=VERTEX_POINT ( 'NONE', #79520 ) ;
#3770=EDGE_CURVE ( 'NONE', #2392, #2085, #58787, .T. ) ;
#3773=DIRECTION ( 'NONE',  ( -0.000000000000000000, 1.000000000000000000, -0.000000000000000000 ) ) ;
#3778=DIRECTION ( 'NONE',  ( 1.000000000000000000, 0.000000000000000000, 0.000000000000000000 ) ) ;
#3789=CARTESIAN_POINT ( 'NONE',  ( 0.000000000000000000, -11.00000000000000000, 29.75000000000000355 ) ) ;
#3798=DIRECTION ( 'NONE',  ( 0.000000000000000000, 0.000000000000000000, -1.000000000000000000 ) ) ;
#3805=VECTOR ( 'NONE', #55218, 1000.000000000000000 ) ;
#3819=VECTOR ( 'NONE', #9595, 1000.000000000000000 ) ;
#3826=CARTESIAN_POINT ( 'NONE',  ( -3.512820512820513663, -3.499999999999999556, 29.75000000000000355 ) ) ;
#3834=EDGE_CURVE ( 'NONE', #29630, #74179, #48822, .T. ) ;
#3839=LINE ( 'NONE', #12384, #43124 ) ;
#3853=LINE ( 'NONE', #67347, #86829 ) ;
#3856=VERTEX_POINT ( 'NONE', #13713 ) ;
#3871=EDGE_LOOP ( 'NONE', ( #60480, #5811, #3957, #27026 ) ) ;
#3876=VERTEX_POINT ( 'NONE', #42087 ) ;
#3885=CARTESIAN_POINT ( 'NONE',  ( -13.19230769230769162, -11.50000000000000000, 29.75000000000000355 ) ) ;
#3886=PLANE ( 'NONE',  #83698 ) ;
#3887=ORIENTED_EDGE ( 'NONE', *, *, #79981, .F. ) ;
#3894=DIRECTION ( 'NONE',  ( 1.000000000000000000, 0.000000000000000000, 0.000000000000000000 ) ) ;
#3898=DIRECTION ( 'NONE',  ( -1.000000000000000000, -0.000000000000000000, -0.000000000000000000 ) ) ;
#3925=ORIENTED_EDGE ( 'NONE', *, *, #49061, .T. ) ;
#3939=VECTOR ( 'NONE', #25329, 1000.000000000000000 ) ;
#3944=DIRECTION ( 'NONE',  ( -1.000000000000000000, -0.000000000000000000, -0.000000000000000000 ) ) ;
#3945=EDGE_CURVE ( 'NONE', #34461, #49704, #58502, .T. ) ;
#3953=FACE_OUTER_BOUND ( 'NONE', #65208, .T. ) ;
#3956=FACE_OUTER_BOUND ( 'NONE', #54120, .T. ) ;
#3957=ORIENTED_EDGE ( 'NONE', *, *, #5157, .T. ) ;
#3972=DIRECTION ( 'NONE',  ( 0.000000000000000000, 0.000000000000000000, -1.000000000000000000 ) ) ;
#3988=CARTESIAN_POINT ( 'NONE',  ( 2.294871794871793380, -7.500000000000000000, 29.75000000000000355 ) ) ;
#3992=ORIENTED_EDGE ( 'NONE', *, *, #52615, .T. ) ;
#3993=ORIENTED_EDGE ( 'NONE', *, *, #44371, .F. ) ;
#3998=CARTESIAN_POINT ( 'NONE',  ( -5.198717948717948012, -7.500000000000000000, 29.75000000000000355 ) ) ;
#4011=EDGE_CURVE ( 'NONE', #64127, #17254, #64104, .T. ) ;
#4022=CIRCLE ( 'NONE', #22682, 4.000000000000000000 ) ;
#4034=FACE_OUTER_BOUND ( 'NONE', #28136, .T. ) ;
#4036=DIRECTION ( 'NONE',  ( -1.000000000000000000, -0.000000000000000000, -0.000000000000000000 ) ) ;
#4042=ORIENTED_EDGE ( 'NONE', *, *, #13960, .T. ) ;
#4049=EDGE_LOOP ( 'NONE', ( #71534, #10954, #36982, #59686 ) ) ;
#4074=ORIENTED_EDGE ( 'NONE', *, *, #75691, .T. ) ;
#4084=VECTOR ( 'NONE', #85447, 1000.000000000000000 ) ;
#4101=ORIENTED_EDGE ( 'NONE', *, *, #50813, .F. ) ;
#4103=EDGE_CURVE ( 'NONE', #9873, #48052, #5861, .T. ) ;
#4107=LINE ( 'NONE', #51381, #45120 ) ;
#4132=ORIENTED_EDGE ( 'NONE', *, *, #13927, .T. ) ;
#4157=DIRECTION ( 'NONE',  ( -0.000000000000000000, 1.000000000000000000, -0.000000000000000000 ) ) ;
#4165=VECTOR ( 'NONE', #4349, 1000.000000000000000 ) ;
#4183=LINE ( 'NONE', #79854, #35127 ) ;
#4184=CARTESIAN_POINT ( 'NONE',  ( -11.00641025641025550, -11.00000000000000000, 29.75000000000000355 ) ) ;
#4196=CARTESIAN_POINT ( 'NONE',  ( -2.294871794871794712, -7.500000000000000000, 29.75000000000000355 ) ) ;
#4213=LINE ( 'NONE', #71778, #7812 ) ;
#4216=ORIENTED_EDGE ( 'NONE', *, *, #61033, .F. ) ;
#4230=ORIENTED_EDGE ( 'NONE', *, *, #52347, .T. ) ;
#4240=EDGE_LOOP ( 'NONE', ( #29342, #74023, #19363, #82436 ) ) ;
#4260=VECTOR ( 'NONE', #42806, 1000.000000000000000 ) ;
#4285=CARTESIAN_POINT ( 'NONE',  ( 0.000000000000000000, -11.00000000000000000, 29.75000000000000355 ) ) ;
#4291=LINE ( 'NONE', #65088, #73741 ) ;
#4294=ADVANCED_FACE ( 'NONE', ( #3953 ), #71088, .F. ) ;
#4307=PLANE ( 'NONE',  #4987 ) ;
#4331=AXIS2_PLACEMENT_3D ( 'NONE', #67044, #88667, #26947 ) ;
#4346=VERTEX_POINT ( 'NONE', #32334 ) ;
#4349=DIRECTION ( 'NONE',  ( -1.000000000000000000, -0.000000000000000000, -0.000000000000000000 ) ) ;
#4357=DIRECTION ( 'NONE',  ( -1.000000000000000000, -0.000000000000000000, 0.000000000000000000 ) ) ;
#4363=CARTESIAN_POINT ( 'NONE',  ( 0.000000000000000000, -11.00000000000000000, 29.75000000000000355 ) ) ;
#4382=CARTESIAN_POINT ( 'NONE',  ( 0.3589743589743582541, -3.499999999999999556, 29.75000000000000355 ) ) ;
#4402=DIRECTION ( 'NONE',  ( -1.000000000000000000, -0.000000000000000000, 0.000000000000000000 ) ) ;
#4432=DIRECTION ( 'NONE',  ( 1.000000000000000000, 0.000000000000000000, 0.000000000000000000 ) ) ;
#4456=PLANE ( 'NONE',  #9739 ) ;
#4458=EDGE_CURVE ( 'NONE', #63745, #58726, #7071, .T. ) ;
#4476=CARTESIAN_POINT ( 'NONE',  ( 19.50000000000000000, -3.499999999999999556, 28.25000000000000000 ) ) ;
#4488=DIRECTION ( 'NONE',  ( 1.000000000000000000, 0.000000000000000000, 0.000000000000000000 ) ) ;
#4495=ORIENTED_EDGE ( 'NONE', *, *, #45969, .T. ) ;
#4517=AXIS2_PLACEMENT_3D ( 'NONE', #59989, #80272, #32967 ) ;
#4526=EDGE_CURVE ( 'NONE', #64401, #65515, #8403, .T. ) ;
#4528=ORIENTED_EDGE ( 'NONE', *, *, #82243, .F. ) ;
#4533=VECTOR ( 'NONE', #81786, 1000.000000000000000 ) ;
#4540=VECTOR ( 'NONE', #9373, 1000.000000000000000 ) ;
#4541=ORIENTED_EDGE ( 'NONE', *, *, #79517, .T. ) ;
#4543=VERTEX_POINT ( 'NONE', #82299 ) ;
#4551=EDGE_CURVE ( 'NONE', #87881, #31043, #62441, .T. ) ;
#4561=ORIENTED_EDGE ( 'NONE', *, *, #201, .F. ) ;
#4566=FACE_OUTER_BOUND ( 'NONE', #29098, .T. ) ;
#4568=ORIENTED_EDGE ( 'NONE', *, *, #76269, .T. ) ;
#4576=VERTEX_POINT ( 'NONE', #84953 ) ;
#4603=FACE_OUTER_BOUND ( 'NONE', #4716, .T. ) ;
#4607=VECTOR ( 'NONE', #22252, 1000.000000000000000 ) ;
#4641=AXIS2_PLACEMENT_3D ( 'NONE', #83628, #62870, #29558 ) ;
#4647=DIRECTION ( 'NONE',  ( 1.000000000000000000, 0.000000000000000000, 0.000000000000000000 ) ) ;
#4652=ORIENTED_EDGE ( 'NONE', *, *, #30004, .F. ) ;
#4663=AXIS2_PLACEMENT_3D ( 'NONE', #31170, #84818, #58196 ) ;
#4665=DIRECTION ( 'NONE',  ( 1.000000000000000000, 0.000000000000000000, 0.000000000000000000 ) ) ;
#4674=ORIENTED_EDGE ( 'NONE', *, *, #55465, .T. ) ;
#4690=VERTEX_POINT ( 'NONE', #66897 ) ;
#4693=ADVANCED_FACE ( 'NONE', ( #18268 ), #12836, .F. ) ;
#4707=DIRECTION ( 'NONE',  ( 1.000000000000000000, 0.000000000000000000, 0.000000000000000000 ) ) ;
#4716=EDGE_LOOP ( 'NONE', ( #63443, #14466, #29500, #67780 ) ) ;
#4717=DIRECTION ( 'NONE',  ( -1.000000000000000000, 0.000000000000000000, -0.000000000000000000 ) ) ;
#4735=EDGE_CURVE ( 'NONE', #88166, #19996, #32622, .T. ) ;
#4740=AXIS2_PLACEMENT_3D ( 'NONE', #57764, #43803, #31628 ) ;
#4749=CARTESIAN_POINT ( 'NONE',  ( -0.3589743589743593088, -7.500000000000000000, 33.75000000000000000 ) ) ;
#4763=ADVANCED_FACE ( 'NONE', ( #15060 ), #42533, .F. ) ;
#4764=ORIENTED_EDGE ( 'NONE', *, *, #40650, .T. ) ;
#4789=( GEOMETRIC_REPRESENTATION_CONTEXT ( 3 ) GLOBAL_UNCERTAINTY_ASSIGNED_CONTEXT ( ( #48799 ) ) GLOBAL_UNIT_ASSIGNED_CONTEXT ( ( #88673, #50737, #78670 ) ) REPRESENTATION_CONTEXT ( 'NONE', 'WORKASPACE' ) );
#4790=ADVANCED_FACE ( 'NONE', ( #6966 ), #69112, .F. ) ;
#4838=FACE_OUTER_BOUND ( 'NONE', #34839, .T. ) ;
#4853=EDGE_CURVE ( 'NONE', #5644, #53642, #69989, .T. ) ;
#4866=ORIENTED_EDGE ( 'NONE', *, *, #51633, .F. ) ;
#4873=EDGE_LOOP ( 'NONE', ( #21431, #65058, #63052, #41099 ) ) ;
#4889=ORIENTED_EDGE ( 'NONE', *, *, #36115, .F. ) ;
#4891=CARTESIAN_POINT ( 'NONE',  ( 14.16025641025641235, -11.50000000000000000, 29.75000000000000355 ) ) ;
#4924=CARTESIAN_POINT ( 'NONE',  ( -19.50000000000000000, -7.500000000000000000, 29.75000000000000355 ) ) ;
#4932=CARTESIAN_POINT ( 'NONE',  ( -19.50000000000000000, -3.499999999999999556, 29.75000000000000355 ) ) ;
#4936=DIRECTION ( 'NONE',  ( -0.000000000000000000, 1.000000000000000000, -0.000000000000000000 ) ) ;
#4958=CYLINDRICAL_SURFACE ( 'NONE', #44058, 4.000000000000000000 ) ;
#4959=EDGE_CURVE ( 'NONE', #88786, #21236, #50603, .T. ) ;
#4960=VERTEX_POINT ( 'NONE', #85290 ) ;
#4977=LINE ( 'NONE', #45947, #71069 ) ;
#4984=VERTEX_POINT ( 'NONE', #73998 ) ;
#4987=AXIS2_PLACEMENT_3D ( 'NONE', #31788, #79533, #38092 ) ;
#5005=DIRECTION ( 'NONE',  ( -1.000000000000000000, -0.000000000000000000, -0.000000000000000000 ) ) ;
#5015=LINE ( 'NONE', #75251, #25653 ) ;
#5016=CARTESIAN_POINT ( 'NONE',  ( 4.480769230769229061, -7.500000000000000000, 33.75000000000000000 ) ) ;
#5018=LINE ( 'NONE', #32481, #8385 ) ;
#5023=ORIENTED_EDGE ( 'NONE', *, *, #80249, .T. ) ;
#5025=CARTESIAN_POINT ( 'NONE',  ( 0.000000000000000000, -11.00000000000000000, 29.75000000000000355 ) ) ;
#5036=CARTESIAN_POINT ( 'NONE',  ( -11.97435897435897267, -3.499999999999999556, 29.75000000000000355 ) ) ;
#5055=ADVANCED_FACE ( 'NONE', ( #46072 ), #86638, .T. ) ;
#5058=DIRECTION ( 'NONE',  ( -1.000000000000000000, -0.000000000000000000, -0.000000000000000000 ) ) ;
#5068=VERTEX_POINT ( 'NONE', #11857 ) ;
#5075=CARTESIAN_POINT ( 'NONE',  ( 19.00000000000000000, -7.500000000000000000, 33.75000000000000000 ) ) ;
#5076=AXIS2_PLACEMENT_3D ( 'NONE', #22433, #43585, #29209 ) ;
#5082=LINE ( 'NONE', #73098, #30014 ) ;
#5087=DIRECTION ( 'NONE',  ( 0.000000000000000000, 0.000000000000000000, -1.000000000000000000 ) ) ;
#5091=ADVANCED_FACE ( 'NONE', ( #2258 ), #37827, .F. ) ;
#5124=ORIENTED_EDGE ( 'NONE', *, *, #84379, .F. ) ;
#5128=ORIENTED_EDGE ( 'NONE', *, *, #26771, .T. ) ;
#5134=LINE ( 'NONE', #33500, #19821 ) ;
#5139=VECTOR ( 'NONE', #74516, 1000.000000000000000 ) ;
#5152=CARTESIAN_POINT ( 'NONE',  ( 0.6089743589743582541, -3.499999999999999556, 29.75000000000000355 ) ) ;
#5154=VERTEX_POINT ( 'NONE', #15800 ) ;
#5155=DIRECTION ( 'NONE',  ( 0.000000000000000000, 0.000000000000000000, -1.000000000000000000 ) ) ;
#5157=EDGE_CURVE ( 'NONE', #24285, #64772, #13965, .T. ) ;
#5184=ADVANCED_FACE ( 'NONE', ( #85139 ), #50448, .F. ) ;
#5185=CIRCLE ( 'NONE', #64636, 4.000000000000000000 ) ;
#5203=DIRECTION ( 'NONE',  ( -0.000000000000000000, 1.000000000000000000, -0.000000000000000000 ) ) ;
#5226=DIRECTION ( 'NONE',  ( -0.000000000000000000, 1.000000000000000000, -0.000000000000000000 ) ) ;
#5228=DIRECTION ( 'NONE',  ( 1.000000000000000000, 0.000000000000000000, 0.000000000000000000 ) ) ;
#5245=DIRECTION ( 'NONE',  ( -1.000000000000000000, 0.000000000000000000, -0.000000000000000000 ) ) ;
#5254=DIRECTION ( 'NONE',  ( -0.000000000000000000, 0.000000000000000000, 1.000000000000000000 ) ) ;
#5260=DIRECTION ( 'NONE',  ( -1.000000000000000000, -0.000000000000000000, -0.000000000000000000 ) ) ;
#5261=FACE_OUTER_BOUND ( 'NONE', #1972, .T. ) ;
#5271=DIRECTION ( 'NONE',  ( 0.000000000000000000, 0.000000000000000000, 1.000000000000000000 ) ) ;
#5294=CARTESIAN_POINT ( 'NONE',  ( 1.326923076923076206, -11.50000000000000000, 29.75000000000000355 ) ) ;
#5295=AXIS2_PLACEMENT_3D ( 'NONE', #28407, #24190, #22101 ) ;
#5298=VERTEX_POINT ( 'NONE', #20714 ) ;
#5302=ORIENTED_EDGE ( 'NONE', *, *, #41534, .T. ) ;
#5306=CIRCLE ( 'NONE', #35530, 4.000000000000000000 ) ;
#5330=FACE_OUTER_BOUND ( 'NONE', #68814, .T. ) ;
#5348=ORIENTED_EDGE ( 'NONE', *, *, #54458, .T. ) ;
#5353=CARTESIAN_POINT ( 'NONE',  ( 20.00000000000000000, -4.000000000000000000, 29.75000000000000355 ) ) ;
#5355=AXIS2_PLACEMENT_3D ( 'NONE', #78495, #22233, #16796 ) ;
#5356=CARTESIAN_POINT ( 'NONE',  ( -2.544871794871794268, -3.499999999999999556, 29.75000000000000355 ) ) ;
#5362=CARTESIAN_POINT ( 'NONE',  ( -8.102564102564102200, -7.500000000000000000, 29.75000000000000355 ) ) ;
#5370=VECTOR ( 'NONE', #81390, 1000.000000000000000 ) ;
#5376=EDGE_CURVE ( 'NONE', #23382, #4960, #58809, .T. ) ;
#5384=EDGE_CURVE ( 'NONE', #38268, #62375, #61914, .T. ) ;
#5385=EDGE_CURVE ( 'NONE', #82638, #50277, #85920, .T. ) ;
#5419=CARTESIAN_POINT ( 'NONE',  ( 0.6089743589743582541, -11.00000000000000000, 29.75000000000000355 ) ) ;
#5423=EDGE_CURVE ( 'NONE', #13394, #88674, #27691, .T. ) ;
#5425=CIRCLE ( 'NONE', #47060, 4.000000000000000000 ) ;
#5461=VECTOR ( 'NONE', #79594, 1000.000000000000000 ) ;
#5468=DIRECTION ( 'NONE',  ( -1.000000000000000000, -0.000000000000000000, 0.000000000000000000 ) ) ;
#5474=DIRECTION ( 'NONE',  ( 0.000000000000000000, 0.000000000000000000, -1.000000000000000000 ) ) ;
#5476=ORIENTED_EDGE ( 'NONE', *, *, #60288, .F. ) ;
#5484=CARTESIAN_POINT ( 'NONE',  ( 6.416666666666664298, -3.499999999999999556, 29.75000000000000355 ) ) ;
#5490=EDGE_LOOP ( 'NONE', ( #68024, #52183, #40695, #29887, #49586 ) ) ;
#5491=CARTESIAN_POINT ( 'NONE',  ( 20.00000000000000000, -4.000000000000000000, 29.75000000000000355 ) ) ;
#5494=AXIS2_PLACEMENT_3D ( 'NONE', #62378, #63274, #16425 ) ;
#5501=VERTEX_POINT ( 'NONE', #42546 ) ;
#5504=DIRECTION ( 'NONE',  ( -1.000000000000000000, -0.000000000000000000, -0.000000000000000000 ) ) ;
#5511=LINE ( 'NONE', #52791, #60013 ) ;
#5521=DIRECTION ( 'NONE',  ( 0.000000000000000000, 0.000000000000000000, -1.000000000000000000 ) ) ;
#5522=FILL_AREA_STYLE ('',( #67224 ) ) ;
#5532=AXIS2_PLACEMENT_3D ( 'NONE', #3664, #37452, #37909 ) ;
#5554=PLANE ( 'NONE',  #79245 ) ;
#5559=ORIENTED_EDGE ( 'NONE', *, *, #55685, .F. ) ;
#5565=VERTEX_POINT ( 'NONE', #69565 ) ;
#5578=ORIENTED_EDGE ( 'NONE', *, *, #84632, .F. ) ;
#5582=ORIENTED_EDGE ( 'NONE', *, *, #86968, .T. ) ;
#5588=DIRECTION ( 'NONE',  ( -0.000000000000000000, 1.000000000000000000, -0.000000000000000000 ) ) ;
#5602=ORIENTED_EDGE ( 'NONE', *, *, #20892, .T. ) ;
#5619=VECTOR ( 'NONE', #37011, 1000.000000000000000 ) ;
#5630=ORIENTED_EDGE ( 'NONE', *, *, #51166, .F. ) ;
#5631=LINE ( 'NONE', #25460, #9828 ) ;
#5633=VERTEX_POINT ( 'NONE', #65469 ) ;
#5644=VERTEX_POINT ( 'NONE', #44740 ) ;
#5649=LINE ( 'NONE', #12849, #3414 ) ;
#5656=ORIENTED_EDGE ( 'NONE', *, *, #11400, .T. ) ;
#5667=DIRECTION ( 'NONE',  ( 1.000000000000000000, 0.000000000000000000, 0.000000000000000000 ) ) ;
#5668=CARTESIAN_POINT ( 'NONE',  ( -19.50000000000000000, -3.499999999999999556, 29.75000000000000355 ) ) ;
#5682=EDGE_CURVE ( 'NONE', #13118, #48938, #51040, .T. ) ;
#5685=DIRECTION ( 'NONE',  ( -1.000000000000000000, -0.000000000000000000, -0.000000000000000000 ) ) ;
#5687=CARTESIAN_POINT ( 'NONE',  ( -7.134615384615385025, -7.500000000000000000, 33.75000000000000000 ) ) ;
#5694=ORIENTED_EDGE ( 'NONE', *, *, #18098, .T. ) ;
#5696=VECTOR ( 'NONE', #83649, 1000.000000000000000 ) ;
#5702=DIRECTION ( 'NONE',  ( -1.000000000000000000, 0.000000000000000000, -0.000000000000000000 ) ) ;
#5714=VECTOR ( 'NONE', #63324, 1000.000000000000000 ) ;
#5719=DIRECTION ( 'NONE',  ( 1.000000000000000000, 0.000000000000000000, 0.000000000000000000 ) ) ;
#5729=FACE_OUTER_BOUND ( 'NONE', #80632, .T. ) ;
#5739=ORIENTED_EDGE ( 'NONE', *, *, #57543, .F. ) ;
#5743=ADVANCED_FACE ( 'NONE', ( #53280 ), #68572, .F. ) ;
#5747=FACE_OUTER_BOUND ( 'NONE', #42025, .T. ) ;
#5749=DIRECTION ( 'NONE',  ( -1.000000000000000000, -0.000000000000000000, -0.000000000000000000 ) ) ;
#5753=VECTOR ( 'NONE', #41479, 1000.000000000000000 ) ;
#5761=VECTOR ( 'NONE', #25421, 1000.000000000000000 ) ;
#5764=CARTESIAN_POINT ( 'NONE',  ( 13.19230769230769340, -4.000000000000000000, 29.75000000000000355 ) ) ;
#5774=DIRECTION ( 'NONE',  ( -1.000000000000000000, -0.000000000000000000, 0.000000000000000000 ) ) ;
#5791=ORIENTED_EDGE ( 'NONE', *, *, #1572, .T. ) ;
#5804=DIRECTION ( 'NONE',  ( -1.000000000000000000, -0.000000000000000000, -0.000000000000000000 ) ) ;
#5809=VERTEX_POINT ( 'NONE', #76667 ) ;
#5811=ORIENTED_EDGE ( 'NONE', *, *, #30990, .T. ) ;
#5816=DIRECTION ( 'NONE',  ( -1.000000000000000000, -0.000000000000000000, 0.000000000000000000 ) ) ;
#5826=CARTESIAN_POINT ( 'NONE',  ( 12.94230769230769340, -4.000000000000000000, 29.75000000000000355 ) ) ;
#5834=AXIS2_PLACEMENT_3D ( 'NONE', #56873, #84368, #72487 ) ;
#5861=LINE ( 'NONE', #25683, #8194 ) ;
#5864=LINE ( 'NONE', #38758, #24848 ) ;
#5870=EDGE_CURVE ( 'NONE', #40595, #7366, #10870, .T. ) ;
#5892=VECTOR ( 'NONE', #53076, 1000.000000000000000 ) ;
#5893=DIRECTION ( 'NONE',  ( 1.000000000000000000, 0.000000000000000000, 0.000000000000000000 ) ) ;
#5894=CARTESIAN_POINT ( 'NONE',  ( 0.000000000000000000, -11.00000000000000000, 29.75000000000000355 ) ) ;
#5895=CYLINDRICAL_SURFACE ( 'NONE', #36611, 4.000000000000000000 ) ;
#5900=VECTOR ( 'NONE', #55086, 1000.000000000000000 ) ;
#5910=FACE_OUTER_BOUND ( 'NONE', #87078, .T. ) ;
#5920=LINE ( 'NONE', #88358, #39585 ) ;
#5941=EDGE_CURVE ( 'NONE', #50855, #66461, #31123, .T. ) ;
#5958=AXIS2_PLACEMENT_3D ( 'NONE', #65402, #51413, #65837 ) ;
#5959=FACE_OUTER_BOUND ( 'NONE', #2351, .T. ) ;
#5961=VERTEX_POINT ( 'NONE', #72560 ) ;
#5964=ORIENTED_EDGE ( 'NONE', *, *, #13142, .T. ) ;
#5979=ORIENTED_EDGE ( 'NONE', *, *, #25373, .F. ) ;
#5989=ORIENTED_EDGE ( 'NONE', *, *, #22457, .T. ) ;
#5990=VERTEX_POINT ( 'NONE', #18959 ) ;
#5998=VECTOR ( 'NONE', #76844, 1000.000000000000000 ) ;
#6024=VECTOR ( 'NONE', #83112, 1000.000000000000000 ) ;
#6027=LINE ( 'NONE', #61835, #57855 ) ;
#6036=AXIS2_PLACEMENT_3D ( 'NONE', #16575, #79619, #58435 ) ;
#6039=EDGE_LOOP ( 'NONE', ( #23897, #26384, #32819, #20124, #6320 ) ) ;
#6058=CARTESIAN_POINT ( 'NONE',  ( -7.384615384615385025, -3.499999999999999556, 29.75000000000000355 ) ) ;
#6062=LINE ( 'NONE', #88065, #81908 ) ;
#6064=ADVANCED_FACE ( 'NONE', ( #45974 ), #47307, .T. ) ;
#6067=LINE ( 'NONE', #68207, #37670 ) ;
#6101=CARTESIAN_POINT ( 'NONE',  ( -17.06410256410256565, -7.500000000000000000, 33.75000000000000000 ) ) ;
#6112=PLANE ( 'NONE',  #43188 ) ;
#6115=VERTEX_POINT ( 'NONE', #8550 ) ;
#6121=CARTESIAN_POINT ( 'NONE',  ( 6.416666666666664298, -7.500000000000000000, 33.75000000000000000 ) ) ;
#6134=CARTESIAN_POINT ( 'NONE',  ( -10.03846153846153832, -1.926643599941765039, 29.65000000000000213 ) ) ;
#6135=LINE ( 'NONE', #66044, #12959 ) ;
#6147=ORIENTED_EDGE ( 'NONE', *, *, #52746, .T. ) ;
#6148=CARTESIAN_POINT ( 'NONE',  ( 11.97435897435897267, -3.499999999999999556, 29.75000000000000355 ) ) ;
#6169=ADVANCED_FACE ( 'NONE', ( #43213 ), #36026, .T. ) ;
#6197=CARTESIAN_POINT ( 'NONE',  ( -19.50000000000000000, -4.000000000000000000, 28.25000000000000000 ) ) ;
#6215=DIRECTION ( 'NONE',  ( 1.000000000000000000, 0.000000000000000000, 0.000000000000000000 ) ) ;
#6216=CARTESIAN_POINT ( 'NONE',  ( 0.000000000000000000, -11.00000000000000000, 29.75000000000000355 ) ) ;
#6226=ORIENTED_EDGE ( 'NONE', *, *, #64141, .F. ) ;
#6237=CARTESIAN_POINT ( 'NONE',  ( 7.384615384615385025, -11.50000000000000000, 29.75000000000000355 ) ) ;
#6242=ORIENTED_EDGE ( 'NONE', *, *, #72877, .F. ) ;
#6244=VECTOR ( 'NONE', #37854, 1000.000000000000000 ) ;
#6261=ORIENTED_EDGE ( 'NONE', *, *, #30593, .T. ) ;
#6269=CARTESIAN_POINT ( 'NONE',  ( 16.81410256410256565, -4.000000000000000000, 29.75000000000000355 ) ) ;
#6283=AXIS2_PLACEMENT_3D ( 'NONE', #19019, #46491, #86154 ) ;
#6284=VECTOR ( 'NONE', #36456, 1000.000000000000000 ) ;
#6319=ORIENTED_EDGE ( 'NONE', *, *, #18918, .F. ) ;
#6320=ORIENTED_EDGE ( 'NONE', *, *, #17694, .F. ) ;
#6322=VERTEX_POINT ( 'NONE', #33697 ) ;
#6324=EDGE_CURVE ( 'NONE', #79249, #2843, #60269, .T. ) ;
#6345=DIRECTION ( 'NONE',  ( -1.000000000000000000, -0.000000000000000000, -0.000000000000000000 ) ) ;
#6349=CARTESIAN_POINT ( 'NONE',  ( -9.070512820512819374, -7.500000000000000000, 29.75000000000000355 ) ) ;
#6359=CARTESIAN_POINT ( 'NONE',  ( -12.22435897435897267, -11.50000000000000000, 29.75000000000000355 ) ) ;
#6369=ORIENTED_EDGE ( 'NONE', *, *, #27784, .F. ) ;
#6376=CARTESIAN_POINT ( 'NONE',  ( 20.00000000000000000, -4.000000000000000000, 29.75000000000000355 ) ) ;
#6379=VECTOR ( 'NONE', #1813, 1000.000000000000000 ) ;
#6384=CARTESIAN_POINT ( 'NONE',  ( 17.06410256410256565, -7.500000000000000000, 29.75000000000000355 ) ) ;
#6390=DIRECTION ( 'NONE',  ( 0.000000000000000000, 0.000000000000000000, 1.000000000000000000 ) ) ;
#6396=ORIENTED_EDGE ( 'NONE', *, *, #28478, .F. ) ;
#6402=DIRECTION ( 'NONE',  ( -0.000000000000000000, 1.000000000000000000, -0.000000000000000000 ) ) ;
#6412=DIRECTION ( 'NONE',  ( 0.000000000000000000, 0.000000000000000000, -1.000000000000000000 ) ) ;
#6420=EDGE_CURVE ( 'NONE', #80799, #72564, #49855, .T. ) ;
#6425=DIRECTION ( 'NONE',  ( -1.000000000000000000, -0.000000000000000000, -0.000000000000000000 ) ) ;
#6433=ADVANCED_FACE ( 'NONE', ( #43109 ), #82334, .T. ) ;
#6464=CARTESIAN_POINT ( 'NONE',  ( -6.166666666666667851, -11.50000000000000000, 29.75000000000000355 ) ) ;
#6467=DIRECTION ( 'NONE',  ( 1.000000000000000000, 0.000000000000000000, 0.000000000000000000 ) ) ;
#6481=CARTESIAN_POINT ( 'NONE',  ( 0.3589743589743582541, -3.499999999999999556, 29.75000000000000355 ) ) ;
#6486=PLANE ( 'NONE',  #23167 ) ;
#6487=CARTESIAN_POINT ( 'NONE',  ( -5.198717948717948012, -7.500000000000000000, 29.75000000000000355 ) ) ;
#6496=VERTEX_POINT ( 'NONE', #792 ) ;
#6497=CARTESIAN_POINT ( 'NONE',  ( 14.16025641025641235, -7.500000000000000000, 29.75000000000000355 ) ) ;
#6501=DIRECTION ( 'NONE',  ( 0.000000000000000000, 0.000000000000000000, -1.000000000000000000 ) ) ;
#6529=EDGE_CURVE ( 'NONE', #52479, #73448, #71629, .T. ) ;
#6531=DIRECTION ( 'NONE',  ( 0.000000000000000000, 0.000000000000000000, -1.000000000000000000 ) ) ;
#6540=ORIENTED_EDGE ( 'NONE', *, *, #53299, .F. ) ;
#6546=DIRECTION ( 'NONE',  ( -0.000000000000000000, 1.000000000000000000, -0.000000000000000000 ) ) ;
#6547=CARTESIAN_POINT ( 'NONE',  ( 1.576923076923075762, -11.00000000000000000, 29.75000000000000355 ) ) ;
#6548=VERTEX_POINT ( 'NONE', #10212 ) ;
#6562=CARTESIAN_POINT ( 'NONE',  ( 14.87820512820512953, -3.499999999999999556, 29.75000000000000355 ) ) ;
#6565=EDGE_CURVE ( 'NONE', #37401, #85779, #78661, .T. ) ;
#6566=FACE_OUTER_BOUND ( 'NONE', #15968, .T. ) ;
#6580=EDGE_CURVE ( 'NONE', #54838, #3756, #72342, .T. ) ;
#6595=AXIS2_PLACEMENT_3D ( 'NONE', #54505, #33360, #41893 ) ;
#6602=LINE ( 'NONE', #12909, #78993 ) ;
#6611=CARTESIAN_POINT ( 'NONE',  ( 14.16025641025641235, -3.499999999999999556, 29.75000000000000355 ) ) ;
#6628=VERTEX_POINT ( 'NONE', #52070 ) ;
#6637=VECTOR ( 'NONE', #33943, 1000.000000000000000 ) ;
#6645=CARTESIAN_POINT ( 'NONE',  ( 10.03846153846153832, -1.926643599941765039, 29.65000000000000213 ) ) ;
#6647=ORIENTED_EDGE ( 'NONE', *, *, #51633, .T. ) ;
#6668=ORIENTED_EDGE ( 'NONE', *, *, #86809, .F. ) ;
#6700=DIRECTION ( 'NONE',  ( -1.000000000000000000, -0.000000000000000000, -0.000000000000000000 ) ) ;
#6707=ORIENTED_EDGE ( 'NONE', *, *, #44492, .T. ) ;
#6732=EDGE_LOOP ( 'NONE', ( #22007, #12714, #55571, #82893, #84727, #32780, #29589, #11892, #20486, #69305, #45069, #41570, #8770, #19516, #76424, #88197, #86066, #77163, #13618, #60068, #66458, #56708, #17357, #40141, #77014, #86223, #6974, #14962, #58072, #65817, #48595, #69662, #76166, #49047, #7948, #45831, #8960, #29724, #48770, #78647, #11151, #80574, #43607, #4541, #80061, #17587, #65323, #24272, #34896, #23065, #26972, #74702, #84230, #24839, #30342, #61277, #20497, #29129, #47612, #44170, #50715, #77781, #14043, #14906, #39795, #47545, #49913, #87314, #87688, #88531, #22922, #85957, #1526, #18470, #10522, #19414, #23812, #10562, #89167, #28977, #73570, #4132, #86573, #37817, #8363, #6647 ) ) ;
#6764=CARTESIAN_POINT ( 'NONE',  ( 12.22435897435897267, -7.500000000000000000, 29.75000000000000355 ) ) ;
#6771=AXIS2_PLACEMENT_3D ( 'NONE', #16870, #44319, #3798 ) ;
#6773=EDGE_CURVE ( 'NONE', #48865, #4543, #11996, .T. ) ;
#6774=EDGE_LOOP ( 'NONE', ( #17258, #68046, #58584, #42297, #2432 ) ) ;
#6783=DIRECTION ( 'NONE',  ( -0.000000000000000000, 1.000000000000000000, -0.000000000000000000 ) ) ;
#6784=CARTESIAN_POINT ( 'NONE',  ( 14.16025641025641235, -11.50000000000000000, 29.75000000000000355 ) ) ;
#6787=DIRECTION ( 'NONE',  ( 1.000000000000000000, 0.000000000000000000, 0.000000000000000000 ) ) ;
#6789=ORIENTED_EDGE ( 'NONE', *, *, #30004, .T. ) ;
#6792=VECTOR ( 'NONE', #55177, 1000.000000000000000 ) ;
#6794=ORIENTED_EDGE ( 'NONE', *, *, #62694, .T. ) ;
#6812=CARTESIAN_POINT ( 'NONE',  ( -11.00641025641025550, -3.499999999999999556, 29.75000000000000355 ) ) ;
#6815=PLANE ( 'NONE',  #64702 ) ;
#6817=EDGE_CURVE ( 'NONE', #60898, #30751, #77567, .T. ) ;
#6836=ORIENTED_EDGE ( 'NONE', *, *, #71965, .F. ) ;
#6849=ORIENTED_EDGE ( 'NONE', *, *, #59724, .F. ) ;
#6858=DIRECTION ( 'NONE',  ( 1.000000000000000000, 0.000000000000000000, 0.000000000000000000 ) ) ;
#6860=EDGE_CURVE ( 'NONE', #61382, #66664, #9543, .T. ) ;
#6877=ORIENTED_EDGE ( 'NONE', *, *, #35665, .T. ) ;
#6902=LINE ( 'NONE', #66836, #8310 ) ;
#6908=DIRECTION ( 'NONE',  ( 0.000000000000000000, 0.000000000000000000, -1.000000000000000000 ) ) ;
#6911=CARTESIAN_POINT ( 'NONE',  ( 16.81410256410256565, -3.499999999999999556, 29.75000000000000355 ) ) ;
#6912=DIRECTION ( 'NONE',  ( -1.000000000000000000, -0.000000000000000000, -0.000000000000000000 ) ) ;
#6914=CARTESIAN_POINT ( 'NONE',  ( 18.75000000000000000, -7.500000000000000000, 33.75000000000000000 ) ) ;
#6916=CARTESIAN_POINT ( 'NONE',  ( 10.03846153846153832, -1.926643599941765039, 29.65000000000000213 ) ) ;
#6918=ADVANCED_FACE ( 'NONE', ( #30270 ), #57738, .T. ) ;
#6924=EDGE_CURVE ( 'NONE', #20735, #50090, #31595, .T. ) ;
#6925=AXIS2_PLACEMENT_3D ( 'NONE', #59193, #4707, #79478 ) ;
#6937=CARTESIAN_POINT ( 'NONE',  ( 16.09615384615384670, -7.500000000000000000, 33.75000000000000000 ) ) ;
#6939=ADVANCED_FACE ( 'NONE', ( #86561 ), #59062, .F. ) ;
#6944=EDGE_CURVE ( 'NONE', #4960, #30751, #85658, .T. ) ;
#6957=CARTESIAN_POINT ( 'NONE',  ( -10.03846153846153832, -7.500000000000000000, 29.75000000000000355 ) ) ;
#6958=CARTESIAN_POINT ( 'NONE',  ( 20.00000000000000000, -4.000000000000000000, 29.75000000000000355 ) ) ;
#6963=VECTOR ( 'NONE', #16964, 1000.000000000000000 ) ;
#6966=FACE_OUTER_BOUND ( 'NONE', #25400, .T. ) ;
#6969=DIRECTION ( 'NONE',  ( -1.000000000000000000, -0.000000000000000000, -0.000000000000000000 ) ) ;
#6970=VERTEX_POINT ( 'NONE', #11778 ) ;
#6974=ORIENTED_EDGE ( 'NONE', *, *, #88867, .F. ) ;
#6983=ORIENTED_EDGE ( 'NONE', *, *, #23229, .T. ) ;
#6985=EDGE_LOOP ( 'NONE', ( #87739, #6986, #36817, #66625 ) ) ;
#6986=ORIENTED_EDGE ( 'NONE', *, *, #52585, .F. ) ;
#6990=EDGE_CURVE ( 'NONE', #1652, #27448, #5018, .T. ) ;
#6998=CARTESIAN_POINT ( 'NONE',  ( 10.03846153846153832, -3.499999999999999556, 29.75000000000000355 ) ) ;
#7010=LINE ( 'NONE', #12441, #31149 ) ;
#7020=CIRCLE ( 'NONE', #47273, 4.000000000000000000 ) ;
#7026=ORIENTED_EDGE ( 'NONE', *, *, #15358, .F. ) ;
#7035=FACE_OUTER_BOUND ( 'NONE', #25856, .T. ) ;
#7036=DIRECTION ( 'NONE',  ( 1.000000000000000000, 0.000000000000000000, 0.000000000000000000 ) ) ;
#7037=CARTESIAN_POINT ( 'NONE',  ( 19.00000000000000000, -7.500000000000000000, 29.75000000000000355 ) ) ;
#7054=EDGE_LOOP ( 'NONE', ( #33026, #20969, #20577, #49044 ) ) ;
#7067=ORIENTED_EDGE ( 'NONE', *, *, #36613, .F. ) ;
#7071=LINE ( 'NONE', #89070, #77224 ) ;
#7072=PLANE ( 'NONE',  #81771 ) ;
#7074=DIRECTION ( 'NONE',  ( -0.000000000000000000, 1.000000000000000000, -0.000000000000000000 ) ) ;
#7093=DIRECTION ( 'NONE',  ( -0.000000000000000000, 1.000000000000000000, -0.000000000000000000 ) ) ;
#7105=EDGE_CURVE ( 'NONE', #35739, #24943, #82901, .T. ) ;
#7112=VECTOR ( 'NONE', #45288, 1000.000000000000000 ) ;
#7117=CARTESIAN_POINT ( 'NONE',  ( -15.84615384615384670, -3.499999999999999556, 29.75000000000000355 ) ) ;
#7122=VECTOR ( 'NONE', #46272, 1000.000000000000000 ) ;
#7126=ORIENTED_EDGE ( 'NONE', *, *, #1679, .T. ) ;
#7139=VERTEX_POINT ( 'NONE', #16202 ) ;
#7147=DIRECTION ( 'NONE',  ( 0.000000000000000000, -0.000000000000000000, 1.000000000000000000 ) ) ;
#7154=LINE ( 'NONE', #80613, #57776 ) ;
#7168=ORIENTED_EDGE ( 'NONE', *, *, #86757, .T. ) ;
#7177=AXIS2_PLACEMENT_3D ( 'NONE', #70355, #36135, #63587 ) ;
#7190=FACE_OUTER_BOUND ( 'NONE', #50073, .T. ) ;
#7193=VECTOR ( 'NONE', #16509, 1000.000000000000000 ) ;
#7207=ORIENTED_EDGE ( 'NONE', *, *, #80705, .T. ) ;
#7214=ORIENTED_EDGE ( 'NONE', *, *, #52463, .T. ) ;
#7217=VECTOR ( 'NONE', #57206, 1000.000000000000000 ) ;
#7226=FACE_OUTER_BOUND ( 'NONE', #77540, .T. ) ;
#7231=DIRECTION ( 'NONE',  ( -0.000000000000000000, 1.000000000000000000, -0.000000000000000000 ) ) ;
#7235=LINE ( 'NONE', #14885, #30321 ) ;
#7244=CIRCLE ( 'NONE', #57574, 4.000000000000000000 ) ;
#7253=VECTOR ( 'NONE', #38968, 1000.000000000000000 ) ;
#7263=DIRECTION ( 'NONE',  ( 0.000000000000000000, 0.000000000000000000, -1.000000000000000000 ) ) ;
#7269=ORIENTED_EDGE ( 'NONE', *, *, #54079, .F. ) ;
#7285=AXIS2_PLACEMENT_3D ( 'NONE', #284, #32733, #25978 ) ;
#7287=LINE ( 'NONE', #13158, #2437 ) ;
#7311=CARTESIAN_POINT ( 'NONE',  ( -7.134615384615385025, -7.500000000000000000, 29.75000000000000355 ) ) ;
#7312=VECTOR ( 'NONE', #71477, 1000.000000000000000 ) ;
#7317=EDGE_LOOP ( 'NONE', ( #51929, #19614, #55066, #88928 ) ) ;
#7318=EDGE_CURVE ( 'NONE', #64772, #24285, #29985, .T. ) ;
#7336=LINE ( 'NONE', #82108, #69095 ) ;
#7345=CARTESIAN_POINT ( 'NONE',  ( -15.84615384615384670, -3.499999999999999556, 29.75000000000000355 ) ) ;
#7348=VECTOR ( 'NONE', #75930, 1000.000000000000000 ) ;
#7351=ORIENTED_EDGE ( 'NONE', *, *, #10327, .T. ) ;
#7353=CARTESIAN_POINT ( 'NONE',  ( 20.00000000000000000, -4.000000000000000000, 29.75000000000000355 ) ) ;
#7358=CARTESIAN_POINT ( 'NONE',  ( 13.91025641025641235, -7.500000000000000000, 29.75000000000000355 ) ) ;
#7362=ORIENTED_EDGE ( 'NONE', *, *, #45497, .T. ) ;
#7366=VERTEX_POINT ( 'NONE', #72023 ) ;
#7367=CARTESIAN_POINT ( 'NONE',  ( -6.166666666666667851, -3.499999999999999556, 29.75000000000000355 ) ) ;
#7379=ORIENTED_EDGE ( 'NONE', *, *, #13473, .F. ) ;
#7381=ORIENTED_EDGE ( 'NONE', *, *, #62694, .F. ) ;
#7388=LINE ( 'NONE', #13692, #55380 ) ;
#7390=AXIS2_PLACEMENT_3D ( 'NONE', #57083, #16540, #50754 ) ;
#7391=EDGE_CURVE ( 'NONE', #83716, #50957, #37799, .T. ) ;
#7400=EDGE_CURVE ( 'NONE', #67446, #54682, #11330, .T. ) ;
#7405=LINE ( 'NONE', #40751, #88621 ) ;
#7408=CARTESIAN_POINT ( 'NONE',  ( -8.102564102564102200, -3.499999999999999556, 29.75000000000000355 ) ) ;
#7446=VERTEX_POINT ( 'NONE', #60736 ) ;
#7465=DIRECTION ( 'NONE',  ( 1.000000000000000000, 0.000000000000000000, 0.000000000000000000 ) ) ;
#7479=EDGE_CURVE ( 'NONE', #62888, #53841, #84714, .T. ) ;
#7481=ORIENTED_EDGE ( 'NONE', *, *, #3154, .T. ) ;
#7487=ORIENTED_EDGE ( 'NONE', *, *, #5385, .F. ) ;
#7526=CARTESIAN_POINT ( 'NONE',  ( -17.06410256410256565, -4.000000000000000000, 29.75000000000000355 ) ) ;
#7527=AXIS2_PLACEMENT_3D ( 'NONE', #33271, #18421, #46333 ) ;
#7532=ORIENTED_EDGE ( 'NONE', *, *, #56827, .T. ) ;
#7534=CIRCLE ( 'NONE', #53563, 4.000000000000000000 ) ;
#7543=DIRECTION ( 'NONE',  ( -1.000000000000000000, -0.000000000000000000, -0.000000000000000000 ) ) ;
#7551=EDGE_CURVE ( 'NONE', #86305, #34265, #49873, .T. ) ;
#7558=CARTESIAN_POINT ( 'NONE',  ( -19.50000000000000000, -3.499999999999999556, 29.75000000000000355 ) ) ;
#7584=EDGE_CURVE ( 'NONE', #21400, #53945, #48537, .T. ) ;
#7586=CARTESIAN_POINT ( 'NONE',  ( 8.102564102564102200, -7.500000000000000000, 29.75000000000000355 ) ) ;
#7589=FACE_OUTER_BOUND ( 'NONE', #54038, .T. ) ;
#7598=DIRECTION ( 'NONE',  ( -1.000000000000000000, -0.000000000000000000, 0.000000000000000000 ) ) ;
#7619=CARTESIAN_POINT ( 'NONE',  ( 14.87820512820512953, -7.500000000000000000, 33.75000000000000000 ) ) ;
#7644=VERTEX_POINT ( 'NONE', #9347 ) ;
#7652=CIRCLE ( 'NONE', #63699, 4.000000000000000000 ) ;
#7666=DIRECTION ( 'NONE',  ( 0.000000000000000000, 0.000000000000000000, 1.000000000000000000 ) ) ;
#7668=DIRECTION ( 'NONE',  ( -1.000000000000000000, -0.000000000000000000, -0.000000000000000000 ) ) ;
#7677=EDGE_CURVE ( 'NONE', #63997, #5154, #37238, .T. ) ;
#7687=CARTESIAN_POINT ( 'NONE',  ( -13.91025641025641058, -3.499999999999999556, 29.75000000000000355 ) ) ;
#7690=ORIENTED_EDGE ( 'NONE', *, *, #64805, .F. ) ;
#7709=ORIENTED_EDGE ( 'NONE', *, *, #17869, .F. ) ;
#7715=EDGE_CURVE ( 'NONE', #81881, #26475, #7020, .T. ) ;
#7753=PLANE ( 'NONE',  #58862 ) ;
#7774=PLANE ( 'NONE',  #14439 ) ;
#7784=DIRECTION ( 'NONE',  ( 0.000000000000000000, 0.000000000000000000, -1.000000000000000000 ) ) ;
#7794=CARTESIAN_POINT ( 'NONE',  ( 0.000000000000000000, -11.00000000000000000, 29.75000000000000355 ) ) ;
#7812=VECTOR ( 'NONE', #44744, 1000.000000000000000 ) ;
#7850=DIRECTION ( 'NONE',  ( 0.000000000000000000, 0.000000000000000000, -1.000000000000000000 ) ) ;
#7873=FACE_OUTER_BOUND ( 'NONE', #28467, .T. ) ;
#7880=VERTEX_POINT ( 'NONE', #20526 ) ;
#7883=CARTESIAN_POINT ( 'NONE',  ( 0.000000000000000000, -11.00000000000000000, 29.75000000000000355 ) ) ;
#7894=DIRECTION ( 'NONE',  ( -1.000000000000000000, -0.000000000000000000, -0.000000000000000000 ) ) ;
#7904=DIRECTION ( 'NONE',  ( -0.000000000000000000, 0.000000000000000000, 1.000000000000000000 ) ) ;
#7921=ORIENTED_EDGE ( 'NONE', *, *, #14548, .T. ) ;
#7932=LINE ( 'NONE', #14689, #79909 ) ;
#7939=DIRECTION ( 'NONE',  ( -1.000000000000000000, -0.000000000000000000, -0.000000000000000000 ) ) ;
#7948=ORIENTED_EDGE ( 'NONE', *, *, #77177, .F. ) ;
#7952=CARTESIAN_POINT ( 'NONE',  ( -12.94230769230769162, -7.500000000000000000, 33.75000000000000000 ) ) ;
#7969=ADVANCED_FACE ( 'NONE', ( #70042 ), #48431, .T. ) ;
#7972=DIRECTION ( 'NONE',  ( -1.000000000000000000, -0.000000000000000000, 0.000000000000000000 ) ) ;
#7973=VERTEX_POINT ( 'NONE', #15551 ) ;
#7995=VERTEX_POINT ( 'NONE', #43901 ) ;
#8005=EDGE_LOOP ( 'NONE', ( #10524, #88073, #64116, #46392 ) ) ;
#8019=CARTESIAN_POINT ( 'NONE',  ( 5.198717948717946236, -7.500000000000000000, 29.75000000000000355 ) ) ;
#8027=PLANE ( 'NONE',  #52136 ) ;
#8036=VECTOR ( 'NONE', #60996, 1000.000000000000000 ) ;
#8053=LINE ( 'NONE', #1731, #26952 ) ;
#8065=ORIENTED_EDGE ( 'NONE', *, *, #33339, .F. ) ;
#8067=DIRECTION ( 'NONE',  ( 1.000000000000000000, 0.000000000000000000, 0.000000000000000000 ) ) ;
#8068=DIRECTION ( 'NONE',  ( -0.000000000000000000, 1.000000000000000000, -0.000000000000000000 ) ) ;
#8078=AXIS2_PLACEMENT_3D ( 'NONE', #21958, #42676, #88668 ) ;
#8096=ORIENTED_EDGE ( 'NONE', *, *, #45232, .F. ) ;
#8124=EDGE_LOOP ( 'NONE', ( #72308, #87766, #31778, #65672 ) ) ;
#8139=CARTESIAN_POINT ( 'NONE',  ( -8.352564102564102200, -7.500000000000000000, 29.75000000000000355 ) ) ;
#8144=EDGE_LOOP ( 'NONE', ( #16860, #78803, #52814, #32722 ) ) ;
#8153=FACE_OUTER_BOUND ( 'NONE', #15511, .T. ) ;
#8183=CARTESIAN_POINT ( 'NONE',  ( -19.50000000000000000, -11.50000000000000000, 29.75000000000000355 ) ) ;
#8193=DIRECTION ( 'NONE',  ( 0.000000000000000000, 0.000000000000000000, 1.000000000000000000 ) ) ;
#8194=VECTOR ( 'NONE', #53595, 1000.000000000000000 ) ;
#8199=CARTESIAN_POINT ( 'NONE',  ( -13.91025641025641058, -3.499999999999999556, 29.75000000000000355 ) ) ;
#8221=DIRECTION ( 'NONE',  ( -1.000000000000000000, -0.000000000000000000, -0.000000000000000000 ) ) ;
#8230=DIRECTION ( 'NONE',  ( -0.000000000000000000, 1.000000000000000000, -0.000000000000000000 ) ) ;
#8252=DIRECTION ( 'NONE',  ( -0.000000000000000000, 1.000000000000000000, -0.000000000000000000 ) ) ;
#8257=LINE ( 'NONE', #82594, #66991 ) ;
#8285=PLANE ( 'NONE',  #5355 ) ;
#8287=VERTEX_POINT ( 'NONE', #62295 ) ;
#8298=VECTOR ( 'NONE', #83941, 1000.000000000000000 ) ;
#8299=ORIENTED_EDGE ( 'NONE', *, *, #49583, .F. ) ;
#8302=DIRECTION ( 'NONE',  ( 0.000000000000000000, 0.000000000000000000, -1.000000000000000000 ) ) ;
#8310=VECTOR ( 'NONE', #53759, 1000.000000000000000 ) ;
#8312=ORIENTED_EDGE ( 'NONE', *, *, #59850, .F. ) ;
#8326=ORIENTED_EDGE ( 'NONE', *, *, #26310, .F. ) ;
#8336=ORIENTED_EDGE ( 'NONE', *, *, #103, .T. ) ;
#8346=DIRECTION ( 'NONE',  ( -1.000000000000000000, -0.000000000000000000, -0.000000000000000000 ) ) ;
#8352=DIRECTION ( 'NONE',  ( -1.000000000000000000, -0.000000000000000000, -0.000000000000000000 ) ) ;
#8357=AXIS2_PLACEMENT_3D ( 'NONE', #11380, #5521, #60895 ) ;
#8363=ORIENTED_EDGE ( 'NONE', *, *, #63023, .F. ) ;
#8367=ORIENTED_EDGE ( 'NONE', *, *, #5384, .F. ) ;
#8385=VECTOR ( 'NONE', #6783, 1000.000000000000000 ) ;
#8390=CARTESIAN_POINT ( 'NONE',  ( 20.00000000000000000, -4.000000000000000000, 29.75000000000000355 ) ) ;
#8393=PLANE ( 'NONE',  #37709 ) ;
#8403=LINE ( 'NONE', #61563, #88766 ) ;
#8411=EDGE_LOOP ( 'NONE', ( #70986, #57155, #45065, #52294, #13962 ) ) ;
#8421=LINE ( 'NONE', #37651, #65263 ) ;
#8434=ORIENTED_EDGE ( 'NONE', *, *, #37084, .F. ) ;
#8457=FACE_OUTER_BOUND ( 'NONE', #24417, .T. ) ;
#8465=LINE ( 'NONE', #40919, #66054 ) ;
#8467=LINE ( 'NONE', #1250, #25708 ) ;
#8486=LINE ( 'NONE', #23310, #31024 ) ;
#8492=CARTESIAN_POINT ( 'NONE',  ( -4.230769230769230838, -11.00000000000000000, 29.75000000000000355 ) ) ;
#8495=EDGE_CURVE ( 'NONE', #15822, #82638, #9546, .T. ) ;
#8497=CARTESIAN_POINT ( 'NONE',  ( -12.22435897435897267, -7.500000000000000000, 33.75000000000000000 ) ) ;
#8502=DIRECTION ( 'NONE',  ( 1.000000000000000000, 0.000000000000000000, 0.000000000000000000 ) ) ;
#8520=EDGE_CURVE ( 'NONE', #55273, #7366, #71687, .T. ) ;
#8541=VERTEX_POINT ( 'NONE', #23938 ) ;
#8543=DIRECTION ( 'NONE',  ( -1.000000000000000000, -0.000000000000000000, -0.000000000000000000 ) ) ;
#8550=CARTESIAN_POINT ( 'NONE',  ( -0.3589743589743593088, -11.00000000000000000, 29.75000000000000355 ) ) ;
#8554=CARTESIAN_POINT ( 'NONE',  ( 14.16025641025641235, -3.499999999999999556, 29.75000000000000355 ) ) ;
#8560=ORIENTED_EDGE ( 'NONE', *, *, #50296, .F. ) ;
#8573=EDGE_CURVE ( 'NONE', #7973, #76696, #18607, .T. ) ;
#8580=CARTESIAN_POINT ( 'NONE',  ( -19.50000000000000000, -3.499999999999999556, 29.75000000000000355 ) ) ;
#8613=CIRCLE ( 'NONE', #74774, 4.000000000000000000 ) ;
#8616=CARTESIAN_POINT ( 'NONE',  ( 0.000000000000000000, -4.000000000000000000, 29.65000000000000213 ) ) ;
#8620=DIRECTION ( 'NONE',  ( -0.000000000000000000, 1.000000000000000000, -0.000000000000000000 ) ) ;
#8633=ADVANCED_FACE ( 'NONE', ( #65813 ), #58615, .T. ) ;
#8635=EDGE_CURVE ( 'NONE', #71093, #62448, #11395, .T. ) ;
#8649=ORIENTED_EDGE ( 'NONE', *, *, #36816, .F. ) ;
#8651=ORIENTED_EDGE ( 'NONE', *, *, #53689, .T. ) ;
#8666=ORIENTED_EDGE ( 'NONE', *, *, #24551, .F. ) ;
#8691=DIRECTION ( 'NONE',  ( 0.000000000000000000, 0.000000000000000000, 1.000000000000000000 ) ) ;
#8706=LINE ( 'NONE', #49242, #73730 ) ;
#8715=ORIENTED_EDGE ( 'NONE', *, *, #40494, .F. ) ;
#8729=ADVANCED_FACE ( 'NONE', ( #5910 ), #61273, .F. ) ;
#8730=VECTOR ( 'NONE', #11999, 1000.000000000000000 ) ;
#8733=VECTOR ( 'NONE', #29711, 1000.000000000000000 ) ;
#8741=CARTESIAN_POINT ( 'NONE',  ( -15.84615384615384670, -7.500000000000000000, 29.75000000000000355 ) ) ;
#8747=EDGE_LOOP ( 'NONE', ( #36110, #40984, #75532, #17105 ) ) ;
#8751=CARTESIAN_POINT ( 'NONE',  ( -14.87820512820512953, -11.50000000000000000, 29.75000000000000355 ) ) ;
#8768=ORIENTED_EDGE ( 'NONE', *, *, #80913, .F. ) ;
#8770=ORIENTED_EDGE ( 'NONE', *, *, #18098, .F. ) ;
#8779=ORIENTED_EDGE ( 'NONE', *, *, #29078, .T. ) ;
#8785=VECTOR ( 'NONE', #73028, 1000.000000000000000 ) ;
#8787=ORIENTED_EDGE ( 'NONE', *, *, #56126, .F. ) ;
#8811=CARTESIAN_POINT ( 'NONE',  ( 2.294871794871793380, -7.500000000000000000, 29.75000000000000355 ) ) ;
#8813=EDGE_CURVE ( 'NONE', #22240, #42959, #9448, .T. ) ;
#8831=EDGE_CURVE ( 'NONE', #53391, #4984, #50850, .T. ) ;
#8835=LINE ( 'NONE', #15588, #61986 ) ;
#8851=VECTOR ( 'NONE', #12312, 1000.000000000000000 ) ;
#8858=ORIENTED_EDGE ( 'NONE', *, *, #27806, .T. ) ;
#8865=DIRECTION ( 'NONE',  ( -1.000000000000000000, -0.000000000000000000, -0.000000000000000000 ) ) ;
#8876=LINE ( 'NONE', #57047, #1863 ) ;
#8894=ORIENTED_EDGE ( 'NONE', *, *, #59168, .T. ) ;
#8935=DIRECTION ( 'NONE',  ( 0.000000000000000000, 0.000000000000000000, -1.000000000000000000 ) ) ;
#8946=EDGE_LOOP ( 'NONE', ( #34097, #5578, #55629, #61111 ) ) ;
#8951=CARTESIAN_POINT ( 'NONE',  ( 5.448717948717947124, -7.500000000000000000, 33.75000000000000000 ) ) ;
#8957=VECTOR ( 'NONE', #27006, 1000.000000000000000 ) ;
#8960=ORIENTED_EDGE ( 'NONE', *, *, #26750, .F. ) ;
#8970=ORIENTED_EDGE ( 'NONE', *, *, #77003, .T. ) ;
#9007=AXIS2_PLACEMENT_3D ( 'NONE', #8811, #84474, #10134 ) ;
#9008=DIRECTION ( 'NONE',  ( 0.000000000000000000, 0.000000000000000000, -1.000000000000000000 ) ) ;
#9015=DIRECTION ( 'NONE',  ( 1.000000000000000000, 0.000000000000000000, 0.000000000000000000 ) ) ;
#9027=LINE ( 'NONE', #36497, #72514 ) ;
#9032=ORIENTED_EDGE ( 'NONE', *, *, #45241, .F. ) ;
#9033=CARTESIAN_POINT ( 'NONE',  ( -2.294871794871794712, -3.499999999999999556, 29.75000000000000355 ) ) ;
#9037=CARTESIAN_POINT ( 'NONE',  ( 20.00000000000000000, -3.499999999999999556, 29.75000000000000355 ) ) ;
#9048=CIRCLE ( 'NONE', #4663, 4.000000000000000000 ) ;
#9049=ADVANCED_FACE ( 'NONE', ( #26074 ), #20207, .F. ) ;
#9050=AXIS2_PLACEMENT_3D ( 'NONE', #75325, #14501, #62676 ) ;
#9054=CARTESIAN_POINT ( 'NONE',  ( 0.000000000000000000, -11.00000000000000000, 29.75000000000000355 ) ) ;
#9059=ORIENTED_EDGE ( 'NONE', *, *, #6924, .T. ) ;
#9062=EDGE_CURVE ( 'NONE', #61963, #18170, #67952, .T. ) ;
#9074=FACE_OUTER_BOUND ( 'NONE', #45275, .T. ) ;
#9080=ORIENTED_EDGE ( 'NONE', *, *, #88924, .T. ) ;
#9084=FACE_OUTER_BOUND ( 'NONE', #84669, .T. ) ;
#9086=CARTESIAN_POINT ( 'NONE',  ( 0.000000000000000000, -3.499999999999999556, 29.25000000000000000 ) ) ;
#9089=PLANE ( 'NONE',  #43867 ) ;
#9096=LINE ( 'NONE', #69457, #50235 ) ;
#9142=AXIS2_PLACEMENT_3D ( 'NONE', #7358, #43353, #1036 ) ;
#9144=DIRECTION ( 'NONE',  ( 1.000000000000000000, 0.000000000000000000, 0.000000000000000000 ) ) ;
#9151=DIRECTION ( 'NONE',  ( -1.000000000000000000, -0.000000000000000000, -0.000000000000000000 ) ) ;
#9164=FACE_OUTER_BOUND ( 'NONE', #78650, .T. ) ;
#9171=CARTESIAN_POINT ( 'NONE',  ( 0.000000000000000000, -11.00000000000000000, 29.75000000000000355 ) ) ;
#9173=VECTOR ( 'NONE', #78196, 1000.000000000000000 ) ;
#9174=ADVANCED_FACE ( 'NONE', ( #28279 ), #58742, .F. ) ;
#9177=CIRCLE ( 'NONE', #20670, 4.000000000000000000 ) ;
#9202=VECTOR ( 'NONE', #21280, 1000.000000000000000 ) ;
#9244=CARTESIAN_POINT ( 'NONE',  ( 19.50000000000000000, -4.000000000000000000, 28.25000000000000000 ) ) ;
#9250=CARTESIAN_POINT ( 'NONE',  ( -7.384615384615385025, -7.500000000000000000, 29.75000000000000355 ) ) ;
#9253=PLANE ( 'NONE',  #47808 ) ;
#9262=DIRECTION ( 'NONE',  ( -0.000000000000000000, 1.000000000000000000, -0.000000000000000000 ) ) ;
#9286=DIRECTION ( 'NONE',  ( -1.000000000000000000, -0.000000000000000000, -0.000000000000000000 ) ) ;
#9291=VECTOR ( 'NONE', #89110, 1000.000000000000000 ) ;
#9292=ORIENTED_EDGE ( 'NONE', *, *, #46342, .T. ) ;
#9295=AXIS2_PLACEMENT_3D ( 'NONE', #48942, #39993, #61567 ) ;
#9303=FACE_OUTER_BOUND ( 'NONE', #22132, .T. ) ;
#9325=EDGE_CURVE ( 'NONE', #61773, #20358, #69497, .T. ) ;
#9332=CARTESIAN_POINT ( 'NONE',  ( 5.448717948717947124, -7.500000000000000000, 33.75000000000000000 ) ) ;
#9333=CARTESIAN_POINT ( 'NONE',  ( -16.09615384615384670, -11.50000000000000000, 29.75000000000000355 ) ) ;
#9347=CARTESIAN_POINT ( 'NONE',  ( -2.544871794871794268, -7.500000000000000000, 33.75000000000000000 ) ) ;
#9349=VECTOR ( 'NONE', #27491, 1000.000000000000000 ) ;
#9355=CARTESIAN_POINT ( 'NONE',  ( 20.00000000000000000, -4.000000000000000000, 29.75000000000000355 ) ) ;
#9373=DIRECTION ( 'NONE',  ( -0.000000000000000000, 1.000000000000000000, -0.000000000000000000 ) ) ;
#9384=EDGE_LOOP ( 'NONE', ( #169, #86856, #59499, #76673 ) ) ;
#9395=EDGE_LOOP ( 'NONE', ( #75224, #42056, #47172, #55235, #42415 ) ) ;
#9400=PLANE ( 'NONE',  #74565 ) ;
#9404=ORIENTED_EDGE ( 'NONE', *, *, #21500, .T. ) ;
#9407=ORIENTED_EDGE ( 'NONE', *, *, #42263, .T. ) ;
#9413=EDGE_LOOP ( 'NONE', ( #37798, #35222, #86346, #41951, #17194 ) ) ;
#9422=PLANE ( 'NONE',  #46519 ) ;
#9429=CARTESIAN_POINT ( 'NONE',  ( -13.91025641025641058, -3.499999999999999556, 29.75000000000000355 ) ) ;
#9430=AXIS2_PLACEMENT_3D ( 'NONE', #14458, #36070, #68952 ) ;
#9431=DIRECTION ( 'NONE',  ( 1.000000000000000000, 0.000000000000000000, 0.000000000000000000 ) ) ;
#9433=VERTEX_POINT ( 'NONE', #10006 ) ;
#9435=ORIENTED_EDGE ( 'NONE', *, *, #24038, .F. ) ;
#9448=LINE ( 'NONE', #42363, #40214 ) ;
#9456=EDGE_LOOP ( 'NONE', ( #8894, #28406, #50049, #88518, #36283 ) ) ;
#9459=CARTESIAN_POINT ( 'NONE',  ( 5.198717948717946236, -3.499999999999999556, 29.75000000000000355 ) ) ;
#9463=EDGE_LOOP ( 'NONE', ( #83758, #87340, #11262, #51150 ) ) ;
#9483=VECTOR ( 'NONE', #20190, 1000.000000000000000 ) ;
#9487=CARTESIAN_POINT ( 'NONE',  ( -5.198717948717946236, -4.000000000000000000, 29.75000000000000355 ) ) ;
#9490=DIRECTION ( 'NONE',  ( 1.000000000000000000, 0.000000000000000000, 0.000000000000000000 ) ) ;
#9513=EDGE_CURVE ( 'NONE', #73448, #24740, #68997, .T. ) ;
#9519=VECTOR ( 'NONE', #81699, 1000.000000000000000 ) ;
#9527=DIRECTION ( 'NONE',  ( 0.000000000000000000, 0.000000000000000000, 1.000000000000000000 ) ) ;
#9529=FACE_OUTER_BOUND ( 'NONE', #29127, .T. ) ;
#9543=LINE ( 'NONE', #63602, #18485 ) ;
#9546=LINE ( 'NONE', #63156, #38725 ) ;
#9550=CARTESIAN_POINT ( 'NONE',  ( 4.480769230769229061, -3.499999999999999556, 29.75000000000000355 ) ) ;
#9560=CARTESIAN_POINT ( 'NONE',  ( -11.97435897435897267, -7.500000000000000000, 33.75000000000000000 ) ) ;
#9573=VECTOR ( 'NONE', #51746, 1000.000000000000000 ) ;
#9587=FACE_OUTER_BOUND ( 'NONE', #10376, .T. ) ;
#9595=DIRECTION ( 'NONE',  ( -1.000000000000000000, -0.000000000000000000, -0.000000000000000000 ) ) ;
#9615=ORIENTED_EDGE ( 'NONE', *, *, #83641, .T. ) ;
#9623=VERTEX_POINT ( 'NONE', #26194 ) ;
#9632=CARTESIAN_POINT ( 'NONE',  ( 3.262820512820510999, -7.500000000000000000, 29.75000000000000355 ) ) ;
#9640=EDGE_LOOP ( 'NONE', ( #52202, #50522, #72406, #78322 ) ) ;
#9641=CARTESIAN_POINT ( 'NONE',  ( 0.000000000000000000, -11.00000000000000000, 29.75000000000000355 ) ) ;
#9643=DIRECTION ( 'NONE',  ( -0.000000000000000000, 1.000000000000000000, -0.000000000000000000 ) ) ;
#9647=ADVANCED_FACE ( 'NONE', ( #87471 ), #80255, .F. ) ;
#9663=ORIENTED_EDGE ( 'NONE', *, *, #41092, .T. ) ;
#9665=LINE ( 'NONE', #23618, #33684 ) ;
#9666=EDGE_LOOP ( 'NONE', ( #89, #41043, #9723, #58789, #79308 ) ) ;
#9684=ORIENTED_EDGE ( 'NONE', *, *, #25027, .F. ) ;
#9694=CARTESIAN_POINT ( 'NONE',  ( 6.416666666666664298, -3.499999999999999556, 29.75000000000000355 ) ) ;
#9708=FACE_OUTER_BOUND ( 'NONE', #67246, .T. ) ;
#9719=CARTESIAN_POINT ( 'NONE',  ( 20.00000000000000000, -4.000000000000000000, 29.75000000000000355 ) ) ;
#9723=ORIENTED_EDGE ( 'NONE', *, *, #42881, .F. ) ;
#9727=AXIS2_PLACEMENT_3D ( 'NONE', #84384, #43385, #42507 ) ;
#9730=ADVANCED_FACE ( 'NONE', ( #75271 ), #40604, .F. ) ;
#9737=DIRECTION ( 'NONE',  ( -1.000000000000000000, 0.000000000000000000, -0.000000000000000000 ) ) ;
#9738=CYLINDRICAL_SURFACE ( 'NONE', #50848, 4.000000000000000000 ) ;
#9739=AXIS2_PLACEMENT_3D ( 'NONE', #80124, #18426, #45886 ) ;
#9764=CARTESIAN_POINT ( 'NONE',  ( -15.12820512820512953, -11.50000000000000000, 29.75000000000000355 ) ) ;
#9773=CARTESIAN_POINT ( 'NONE',  ( -19.00000000000000000, -7.500000000000000000, 29.75000000000000355 ) ) ;
#9790=VECTOR ( 'NONE', #9286, 1000.000000000000000 ) ;
#9795=LINE ( 'NONE', #35168, #32613 ) ;
#9810=EDGE_CURVE ( 'NONE', #27448, #14834, #37363, .T. ) ;
#9819=EDGE_CURVE ( 'NONE', #68727, #71459, #36925, .T. ) ;
#9821=DIRECTION ( 'NONE',  ( 1.000000000000000000, 0.000000000000000000, 0.000000000000000000 ) ) ;
#9826=DIRECTION ( 'NONE',  ( -1.000000000000000000, 0.000000000000000000, -0.000000000000000000 ) ) ;
#9828=VECTOR ( 'NONE', #53370, 1000.000000000000000 ) ;
#9854=ORIENTED_EDGE ( 'NONE', *, *, #36587, .F. ) ;
#9862=CARTESIAN_POINT ( 'NONE',  ( 2.294871794871793380, -7.500000000000000000, 33.75000000000000000 ) ) ;
#9873=VERTEX_POINT ( 'NONE', #71592 ) ;
#9876=AXIS2_PLACEMENT_3D ( 'NONE', #51296, #84699, #85131 ) ;
#9891=VERTEX_POINT ( 'NONE', #85128 ) ;
#9902=EDGE_LOOP ( 'NONE', ( #44486, #12934, #46200, #87148, #46539 ) ) ;
#9912=DIRECTION ( 'NONE',  ( 0.000000000000000000, 0.000000000000000000, -1.000000000000000000 ) ) ;
#9916=CARTESIAN_POINT ( 'NONE',  ( -9.070512820512819374, -4.000000000000000000, 29.75000000000000355 ) ) ;
#9945=VECTOR ( 'NONE', #66875, 1000.000000000000000 ) ;
#9954=DIRECTION ( 'NONE',  ( -1.000000000000000000, -0.000000000000000000, -0.000000000000000000 ) ) ;
#9959=ORIENTED_EDGE ( 'NONE', *, *, #10586, .T. ) ;
#9960=ORIENTED_EDGE ( 'NONE', *, *, #64405, .F. ) ;
#9967=CYLINDRICAL_SURFACE ( 'NONE', #41115, 4.000000000000000000 ) ;
#9969=ORIENTED_EDGE ( 'NONE', *, *, #88741, .F. ) ;
#9975=CARTESIAN_POINT ( 'NONE',  ( 10.03846153846153832, -1.926643599941765039, 29.65000000000000213 ) ) ;
#9986=DIRECTION ( 'NONE',  ( 0.000000000000000000, 0.000000000000000000, 1.000000000000000000 ) ) ;
#9993=AXIS2_PLACEMENT_3D ( 'NONE', #19318, #53983, #19758 ) ;
#10005=VECTOR ( 'NONE', #3773, 1000.000000000000000 ) ;
#10006=CARTESIAN_POINT ( 'NONE',  ( 3.262820512820510999, -11.00000000000000000, 29.75000000000000355 ) ) ;
#10008=AXIS2_PLACEMENT_3D ( 'NONE', #13367, #12927, #82727 ) ;
#10041=CARTESIAN_POINT ( 'NONE',  ( -19.50000000000000000, -3.499999999999999556, 29.75000000000000355 ) ) ;
#10045=CARTESIAN_POINT ( 'NONE',  ( -12.94230769230769340, -4.000000000000000000, 29.75000000000000355 ) ) ;
#10052=EDGE_CURVE ( 'NONE', #78478, #17849, #59425, .T. ) ;
#10061=AXIS2_PLACEMENT_3D ( 'NONE', #79322, #52281, #38332 ) ;
#10064=DIRECTION ( 'NONE',  ( 0.000000000000000000, 0.000000000000000000, 1.000000000000000000 ) ) ;
#10092=DIRECTION ( 'NONE',  ( 0.000000000000000000, 0.000000000000000000, -1.000000000000000000 ) ) ;
#10094=ORIENTED_EDGE ( 'NONE', *, *, #27779, .F. ) ;
#10095=VECTOR ( 'NONE', #54775, 1000.000000000000000 ) ;
#10114=ORIENTED_EDGE ( 'NONE', *, *, #17333, .T. ) ;
#10123=VECTOR ( 'NONE', #7668, 1000.000000000000000 ) ;
#10131=ORIENTED_EDGE ( 'NONE', *, *, #71669, .T. ) ;
#10134=DIRECTION ( 'NONE',  ( 0.000000000000000000, 0.000000000000000000, -1.000000000000000000 ) ) ;
#10135=ADVANCED_FACE ( 'NONE', ( #60756 ), #68843, .F. ) ;
#10147=FACE_OUTER_BOUND ( 'NONE', #88297, .T. ) ;
#10154=CARTESIAN_POINT ( 'NONE',  ( -6.416666666666667851, -3.499999999999999556, 29.75000000000000355 ) ) ;
#10160=DIRECTION ( 'NONE',  ( -1.000000000000000000, 0.000000000000000000, -0.000000000000000000 ) ) ;
#10184=VECTOR ( 'NONE', #42027, 1000.000000000000000 ) ;
#10211=DIRECTION ( 'NONE',  ( 1.000000000000000000, 0.000000000000000000, 0.000000000000000000 ) ) ;
#10212=CARTESIAN_POINT ( 'NONE',  ( 19.00000000000000000, -11.50000000000000000, 29.75000000000000355 ) ) ;
#10215=CARTESIAN_POINT ( 'NONE',  ( -14.87820512820512953, -7.500000000000000000, 33.75000000000000000 ) ) ;
#10217=CARTESIAN_POINT ( 'NONE',  ( 11.25641025641025550, -11.50000000000000000, 29.75000000000000355 ) ) ;
#10252=CARTESIAN_POINT ( 'NONE',  ( -19.50000000000000000, -3.499999999999999556, 29.75000000000000355 ) ) ;
#10268=LINE ( 'NONE', #8616, #50245 ) ;
#10274=VECTOR ( 'NONE', #87686, 1000.000000000000000 ) ;
#10280=EDGE_LOOP ( 'NONE', ( #88879, #83982, #85742, #32925, #69482 ) ) ;
#10293=ORIENTED_EDGE ( 'NONE', *, *, #33937, .F. ) ;
#10303=ORIENTED_EDGE ( 'NONE', *, *, #76518, .T. ) ;
#10308=LINE ( 'NONE', #87325, #10585 ) ;
#10311=EDGE_CURVE ( 'NONE', #22055, #54542, #36393, .T. ) ;
#10312=DIRECTION ( 'NONE',  ( -1.000000000000000000, -0.000000000000000000, 0.000000000000000000 ) ) ;
#10319=LINE ( 'NONE', #51722, #15983 ) ;
#10327=EDGE_CURVE ( 'NONE', #66664, #30312, #50765, .T. ) ;
#10341=EDGE_LOOP ( 'NONE', ( #73695, #18486, #19239, #8336 ) ) ;
#10345=CARTESIAN_POINT ( 'NONE',  ( -19.50000000000000000, -11.50000000000000000, 29.75000000000000355 ) ) ;
#10350=EDGE_CURVE ( 'NONE', #21924, #27341, #52109, .T. ) ;
#10355=VERTEX_POINT ( 'NONE', #32298 ) ;
#10356=DIRECTION ( 'NONE',  ( 0.000000000000000000, 0.000000000000000000, -1.000000000000000000 ) ) ;
#10376=EDGE_LOOP ( 'NONE', ( #23159, #28106, #44586, #21061 ) ) ;
#10388=DIRECTION ( 'NONE',  ( 0.000000000000000000, 0.000000000000000000, -1.000000000000000000 ) ) ;
#10399=VECTOR ( 'NONE', #22780, 1000.000000000000000 ) ;
#10406=ORIENTED_EDGE ( 'NONE', *, *, #52347, .F. ) ;
#10412=CARTESIAN_POINT ( 'NONE',  ( -19.50000000000000000, -11.50000000000000000, 29.75000000000000355 ) ) ;
#10424=ORIENTED_EDGE ( 'NONE', *, *, #51993, .F. ) ;
#10475=ORIENTED_EDGE ( 'NONE', *, *, #8831, .F. ) ;
#10477=DIRECTION ( 'NONE',  ( 0.000000000000000000, 0.000000000000000000, -1.000000000000000000 ) ) ;
#10491=ORIENTED_EDGE ( 'NONE', *, *, #59941, .T. ) ;
#10495=DIRECTION ( 'NONE',  ( -1.000000000000000000, -0.000000000000000000, -0.000000000000000000 ) ) ;
#10501=PLANE ( 'NONE',  #58464 ) ;
#10513=MECHANICAL_DESIGN_GEOMETRIC_PRESENTATION_REPRESENTATION('',(#49347),#4789);
#10522=ORIENTED_EDGE ( 'NONE', *, *, #37549, .F. ) ;
#10524=ORIENTED_EDGE ( 'NONE', *, *, #54773, .F. ) ;
#10526=CARTESIAN_POINT ( 'NONE',  ( 7.384615384615385025, -3.499999999999999556, 29.75000000000000355 ) ) ;
#10553=DIRECTION ( 'NONE',  ( 1.000000000000000000, 0.000000000000000000, 0.000000000000000000 ) ) ;
#10557=DIRECTION ( 'NONE',  ( -0.000000000000000000, 1.000000000000000000, -0.000000000000000000 ) ) ;
#10558=DIRECTION ( 'NONE',  ( -1.000000000000000000, -0.000000000000000000, -0.000000000000000000 ) ) ;
#10562=ORIENTED_EDGE ( 'NONE', *, *, #775, .T. ) ;
#10572=DIRECTION ( 'NONE',  ( 0.000000000000000000, 0.000000000000000000, 1.000000000000000000 ) ) ;
#10573=DIRECTION ( 'NONE',  ( 0.000000000000000000, 0.000000000000000000, -1.000000000000000000 ) ) ;
#10581=EDGE_CURVE ( 'NONE', #88786, #31128, #27312, .T. ) ;
#10582=VECTOR ( 'NONE', #79390, 1000.000000000000000 ) ;
#10585=VECTOR ( 'NONE', #25600, 1000.000000000000000 ) ;
#10586=EDGE_CURVE ( 'NONE', #83291, #32479, #67413, .T. ) ;
#10607=DIRECTION ( 'NONE',  ( -1.000000000000000000, -0.000000000000000000, -0.000000000000000000 ) ) ;
#10612=ADVANCED_FACE ( 'NONE', ( #7035 ), #34512, .F. ) ;
#10623=EDGE_LOOP ( 'NONE', ( #18195, #86501, #4042, #44837 ) ) ;
#10625=CIRCLE ( 'NONE', #82529, 4.000000000000000000 ) ;
#10631=DIRECTION ( 'NONE',  ( -1.000000000000000000, -0.000000000000000000, 0.000000000000000000 ) ) ;
#10635=EDGE_CURVE ( 'NONE', #6496, #36253, #23210, .T. ) ;
#10656=DIRECTION ( 'NONE',  ( 0.000000000000000000, 0.000000000000000000, -1.000000000000000000 ) ) ;
#10664=ORIENTED_EDGE ( 'NONE', *, *, #22912, .F. ) ;
#10668=CARTESIAN_POINT ( 'NONE',  ( 0.000000000000000000, -11.00000000000000000, 29.75000000000000355 ) ) ;
#10675=LINE ( 'NONE', #50312, #41052 ) ;
#10688=CARTESIAN_POINT ( 'NONE',  ( 4.230769230769229061, -11.50000000000000000, 29.75000000000000355 ) ) ;
#10697=VECTOR ( 'NONE', #49299, 1000.000000000000000 ) ;
#10704=VECTOR ( 'NONE', #60762, 1000.000000000000000 ) ;
#10706=DIRECTION ( 'NONE',  ( -0.000000000000000000, 0.000000000000000000, 1.000000000000000000 ) ) ;
#10707=ORIENTED_EDGE ( 'NONE', *, *, #53737, .T. ) ;
#10721=CARTESIAN_POINT ( 'NONE',  ( 20.00000000000000000, -4.000000000000000000, 29.75000000000000355 ) ) ;
#10733=CARTESIAN_POINT ( 'NONE',  ( -17.06410256410256565, -11.00000000000000000, 29.75000000000000355 ) ) ;
#10743=ADVANCED_FACE ( 'NONE', ( #10147 ), #86721, .F. ) ;
#10756=DIRECTION ( 'NONE',  ( 0.000000000000000000, 0.000000000000000000, -1.000000000000000000 ) ) ;
#10760=CARTESIAN_POINT ( 'NONE',  ( 20.00000000000000000, -4.000000000000000000, 29.75000000000000355 ) ) ;
#10762=CARTESIAN_POINT ( 'NONE',  ( -1.326923076923076872, -7.500000000000000000, 29.75000000000000355 ) ) ;
#10776=CARTESIAN_POINT ( 'NONE',  ( 0.000000000000000000, -11.00000000000000000, 29.25000000000000000 ) ) ;
#10797=AXIS2_PLACEMENT_3D ( 'NONE', #70842, #9144, #36604 ) ;
#10802=DIRECTION ( 'NONE',  ( 1.000000000000000000, 0.000000000000000000, 0.000000000000000000 ) ) ;
#10811=CARTESIAN_POINT ( 'NONE',  ( 8.352564102564102200, -7.500000000000000000, 29.75000000000000355 ) ) ;
#10834=CARTESIAN_POINT ( 'NONE',  ( 20.00000000000000000, -4.000000000000000000, 29.75000000000000355 ) ) ;
#10840=AXIS2_PLACEMENT_3D ( 'NONE', #46090, #18175, #39785 ) ;
#10844=EDGE_CURVE ( 'NONE', #21562, #58964, #27542, .T. ) ;
#10858=AXIS2_PLACEMENT_3D ( 'NONE', #34848, #20460, #67761 ) ;
#10870=LINE ( 'NONE', #3212, #71555 ) ;
#10873=CARTESIAN_POINT ( 'NONE',  ( 10.28846153846153832, -11.50000000000000000, 29.75000000000000355 ) ) ;
#10876=ORIENTED_EDGE ( 'NONE', *, *, #68229, .T. ) ;
#10899=LINE ( 'NONE', #57750, #65410 ) ;
#10951=EDGE_CURVE ( 'NONE', #57687, #72142, #86948, .T. ) ;
#10954=ORIENTED_EDGE ( 'NONE', *, *, #43118, .F. ) ;
#10958=DIRECTION ( 'NONE',  ( 0.000000000000000000, 0.000000000000000000, 1.000000000000000000 ) ) ;
#10959=VECTOR ( 'NONE', #60018, 1000.000000000000000 ) ;
#10988=CARTESIAN_POINT ( 'NONE',  ( 0.3589743589743582541, -3.499999999999999556, 29.75000000000000355 ) ) ;
#11004=DIRECTION ( 'NONE',  ( 0.000000000000000000, 0.000000000000000000, -1.000000000000000000 ) ) ;
#11039=DIRECTION ( 'NONE',  ( -1.000000000000000000, -0.000000000000000000, -0.000000000000000000 ) ) ;
#11047=EDGE_LOOP ( 'NONE', ( #69568, #64526, #28938, #58143 ) ) ;
#11056=VECTOR ( 'NONE', #28002, 1000.000000000000000 ) ;
#11065=DIRECTION ( 'NONE',  ( 1.000000000000000000, 0.000000000000000000, 0.000000000000000000 ) ) ;
#11074=ORIENTED_EDGE ( 'NONE', *, *, #5941, .T. ) ;
#11076=LINE ( 'NONE', #73224, #25823 ) ;
#11078=DIRECTION ( 'NONE',  ( -1.000000000000000000, -0.000000000000000000, -0.000000000000000000 ) ) ;
#11091=ORIENTED_EDGE ( 'NONE', *, *, #11555, .T. ) ;
#11100=CARTESIAN_POINT ( 'NONE',  ( 0.6089743589743582541, -7.500000000000000000, 33.75000000000000000 ) ) ;
#11109=LINE ( 'NONE', #46229, #71650 ) ;
#11117=PLANE ( 'NONE',  #82335 ) ;
#11137=LINE ( 'NONE', #37716, #18946 ) ;
#11139=ORIENTED_EDGE ( 'NONE', *, *, #5384, .T. ) ;
#11146=CARTESIAN_POINT ( 'NONE',  ( 4.480769230769229061, -3.499999999999999556, 29.75000000000000355 ) ) ;
#11151=ORIENTED_EDGE ( 'NONE', *, *, #22457, .F. ) ;
#11154=VECTOR ( 'NONE', #19018, 1000.000000000000000 ) ;
#11155=ADVANCED_FACE ( 'NONE', ( #54452, #62100, #75186, #28311 ), #89157, .F. ) ;
#11172=DIRECTION ( 'NONE',  ( -1.000000000000000000, -0.000000000000000000, -0.000000000000000000 ) ) ;
#11175=ORIENTED_EDGE ( 'NONE', *, *, #28655, .T. ) ;
#11178=ORIENTED_EDGE ( 'NONE', *, *, #84873, .T. ) ;
#11205=DIRECTION ( 'NONE',  ( 0.000000000000000000, 0.000000000000000000, -1.000000000000000000 ) ) ;
#11208=AXIS2_PLACEMENT_3D ( 'NONE', #17586, #71620, #45036 ) ;
#11223=DIRECTION ( 'NONE',  ( -1.000000000000000000, 0.000000000000000000, -0.000000000000000000 ) ) ;
#11232=ORIENTED_EDGE ( 'NONE', *, *, #71061, .T. ) ;
#11236=LINE ( 'NONE', #80142, #48836 ) ;
#11262=ORIENTED_EDGE ( 'NONE', *, *, #60230, .T. ) ;
#11292=AXIS2_PLACEMENT_3D ( 'NONE', #46361, #68405, #86936 ) ;
#11303=EDGE_CURVE ( 'NONE', #26164, #73448, #32314, .T. ) ;
#11308=CARTESIAN_POINT ( 'NONE',  ( -4.480769230769230838, -7.500000000000000000, 33.75000000000000000 ) ) ;
#11321=CARTESIAN_POINT ( 'NONE',  ( -19.50000000000000000, -3.499999999999999556, 29.75000000000000355 ) ) ;
#11330=CIRCLE ( 'NONE', #45847, 4.000000000000000000 ) ;
#11334=EDGE_LOOP ( 'NONE', ( #35981, #75989, #32268, #85677, #58131 ) ) ;
#11346=VERTEX_POINT ( 'NONE', #25551 ) ;
#11360=AXIS2_PLACEMENT_3D ( 'NONE', #32553, #4647, #85733 ) ;
#11380=CARTESIAN_POINT ( 'NONE',  ( -19.50000000000000000, -3.499999999999999556, 29.75000000000000355 ) ) ;
#11395=CIRCLE ( 'NONE', #30105, 4.000000000000000000 ) ;
#11400=EDGE_CURVE ( 'NONE', #79802, #12929, #67714, .T. ) ;
#11405=EDGE_CURVE ( 'NONE', #20924, #30751, #33642, .T. ) ;
#11417=VECTOR ( 'NONE', #35791, 1000.000000000000000 ) ;
#11421=DIRECTION ( 'NONE',  ( -1.000000000000000000, 0.000000000000000000, -0.000000000000000000 ) ) ;
#11424=AXIS2_PLACEMENT_3D ( 'NONE', #52103, #59310, #5702 ) ;
#11436=DIRECTION ( 'NONE',  ( 1.000000000000000000, 0.000000000000000000, 0.000000000000000000 ) ) ;
#11465=CARTESIAN_POINT ( 'NONE',  ( 18.03205128205128105, -3.499999999999999556, 29.75000000000000355 ) ) ;
#11471=ORIENTED_EDGE ( 'NONE', *, *, #21667, .T. ) ;
#11489=EDGE_CURVE ( 'NONE', #48658, #5961, #140, .T. ) ;
#11492=VECTOR ( 'NONE', #49536, 1000.000000000000000 ) ;
#11498=VERTEX_POINT ( 'NONE', #83162 ) ;
#11500=PLANE ( 'NONE',  #50301 ) ;
#11505=VECTOR ( 'NONE', #21155, 1000.000000000000000 ) ;
#11506=DIRECTION ( 'NONE',  ( -0.000000000000000000, 1.000000000000000000, -0.000000000000000000 ) ) ;
#11513=DIRECTION ( 'NONE',  ( 1.000000000000000000, 0.000000000000000000, 0.000000000000000000 ) ) ;
#11522=DIRECTION ( 'NONE',  ( -0.000000000000000000, 1.000000000000000000, -0.000000000000000000 ) ) ;
#11525=CARTESIAN_POINT ( 'NONE',  ( 0.000000000000000000, -11.00000000000000000, 29.75000000000000355 ) ) ;
#11554=DIRECTION ( 'NONE',  ( 0.000000000000000000, 0.000000000000000000, -1.000000000000000000 ) ) ;
#11555=EDGE_CURVE ( 'NONE', #77416, #83736, #8835, .T. ) ;
#11558=AXIS2_PLACEMENT_3D ( 'NONE', #84979, #49418, #21942 ) ;
#11561=CARTESIAN_POINT ( 'NONE',  ( 8.352564102564102200, -7.500000000000000000, 33.75000000000000000 ) ) ;
#11578=DIRECTION ( 'NONE',  ( -0.000000000000000000, 1.000000000000000000, -0.000000000000000000 ) ) ;
#11579=FACE_OUTER_BOUND ( 'NONE', #57814, .T. ) ;
#11593=ORIENTED_EDGE ( 'NONE', *, *, #34870, .T. ) ;
#11602=VERTEX_POINT ( 'NONE', #63761 ) ;
#11614=VECTOR ( 'NONE', #12329, 1000.000000000000000 ) ;
#11647=CIRCLE ( 'NONE', #66291, 4.000000000000000000 ) ;
#11658=LINE ( 'NONE', #88226, #23038 ) ;
#11681=CARTESIAN_POINT ( 'NONE',  ( -3.512820512820514995, -4.000000000000000000, 29.75000000000000355 ) ) ;
#11694=AXIS2_PLACEMENT_3D ( 'NONE', #75800, #6467, #61836 ) ;
#11698=PLANE ( 'NONE',  #22298 ) ;
#11702=DIRECTION ( 'NONE',  ( -0.000000000000000000, 1.000000000000000000, -0.000000000000000000 ) ) ;
#11720=VERTEX_POINT ( 'NONE', #13211 ) ;
#11739=EDGE_CURVE ( 'NONE', #83736, #30367, #47877, .T. ) ;
#11744=EDGE_LOOP ( 'NONE', ( #37988, #51134, #20401, #31272, #45517 ) ) ;
#11750=ORIENTED_EDGE ( 'NONE', *, *, #84771, .F. ) ;
#11751=LINE ( 'NONE', #25259, #32480 ) ;
#11759=DIRECTION ( 'NONE',  ( 0.000000000000000000, 0.000000000000000000, -1.000000000000000000 ) ) ;
#11768=EDGE_CURVE ( 'NONE', #59129, #17957, #87943, .T. ) ;
#11778=CARTESIAN_POINT ( 'NONE',  ( -6.166666666666667851, -4.000000000000000000, 29.75000000000000355 ) ) ;
#11786=EDGE_LOOP ( 'NONE', ( #81747, #58600, #21146, #2279, #78024, #81684, #26917, #22752, #44699, #28036, #1092, #54484, #46566, #85352, #75983, #46149, #40359, #76800, #30647, #15158, #85073, #84949, #37862, #86317, #10406, #11139, #40252, #25292, #61926, #2434, #53309, #35326, #58106, #67871, #83489, #18129, #75727, #53301, #36157, #50719, #79728, #63123, #17530, #86073, #41626, #30701, #30650, #78169, #21478, #1992, #30205, #57152, #32586, #42760, #45603, #38976, #44053, #77305, #59553, #75258, #47396, #45939, #35971, #33373, #3993, #80361, #53610, #46528, #26508, #35802, #12841, #35703, #15423, #60400, #39197, #74072, #73796, #86199, #3492, #35711, #69423, #45285, #59915, #61486, #74999, #50583 ) ) ;
#11794=DIRECTION ( 'NONE',  ( -1.000000000000000000, -0.000000000000000000, -0.000000000000000000 ) ) ;
#11807=ADVANCED_FACE ( 'NONE', ( #40248 ), #67712, .F. ) ;
#11820=CARTESIAN_POINT ( 'NONE',  ( 0.000000000000000000, -11.00000000000000000, 29.75000000000000355 ) ) ;
#11821=LINE ( 'NONE', #17685, #38956 ) ;
#11822=VECTOR ( 'NONE', #48917, 1000.000000000000000 ) ;
#11835=DIRECTION ( 'NONE',  ( 1.000000000000000000, 0.000000000000000000, 0.000000000000000000 ) ) ;
#11837=DIRECTION ( 'NONE',  ( 0.000000000000000000, 0.000000000000000000, -1.000000000000000000 ) ) ;
#11843=DIRECTION ( 'NONE',  ( -1.000000000000000000, -0.000000000000000000, -0.000000000000000000 ) ) ;
#11845=AXIS2_PLACEMENT_3D ( 'NONE', #51062, #7894, #1133 ) ;
#11856=ADVANCED_FACE ( 'NONE', ( #25527 ), #39500, .T. ) ;
#11857=CARTESIAN_POINT ( 'NONE',  ( 3.512820512820510555, -3.499999999999999556, 29.75000000000000355 ) ) ;
#11880=VERTEX_POINT ( 'NONE', #12892 ) ;
#11892=ORIENTED_EDGE ( 'NONE', *, *, #20072, .T. ) ;
#11920=DIRECTION ( 'NONE',  ( 0.000000000000000000, 0.000000000000000000, -1.000000000000000000 ) ) ;
#11928=EDGE_CURVE ( 'NONE', #43735, #71459, #84035, .T. ) ;
#11944=LINE ( 'NONE', #66880, #79535 ) ;
#11950=CARTESIAN_POINT ( 'NONE',  ( -19.50000000000000000, -3.499999999999999556, 29.75000000000000355 ) ) ;
#11960=ORIENTED_EDGE ( 'NONE', *, *, #56342, .F. ) ;
#11976=DIRECTION ( 'NONE',  ( 1.000000000000000000, 0.000000000000000000, 0.000000000000000000 ) ) ;
#11985=ORIENTED_EDGE ( 'NONE', *, *, #11405, .T. ) ;
#11987=DIRECTION ( 'NONE',  ( 0.000000000000000000, 0.000000000000000000, -1.000000000000000000 ) ) ;
#11996=LINE ( 'NONE', #45766, #47195 ) ;
#11999=DIRECTION ( 'NONE',  ( 1.000000000000000000, 0.000000000000000000, 0.000000000000000000 ) ) ;
#12001=VECTOR ( 'NONE', #6546, 1000.000000000000000 ) ;
#12002=LINE ( 'NONE', #46661, #62075 ) ;
#12026=DIRECTION ( 'NONE',  ( 0.000000000000000000, 0.000000000000000000, -1.000000000000000000 ) ) ;
#12036=VECTOR ( 'NONE', #17871, 1000.000000000000000 ) ;
#12047=ADVANCED_FACE ( 'NONE', ( #33524 ), #72716, .F. ) ;
#12049=CARTESIAN_POINT ( 'NONE',  ( -19.50000000000000000, -3.499999999999999556, 29.75000000000000355 ) ) ;
#12054=FACE_OUTER_BOUND ( 'NONE', #72107, .T. ) ;
#12071=EDGE_LOOP ( 'NONE', ( #19629, #61689, #89120, #56208, #13405 ) ) ;
#12080=ORIENTED_EDGE ( 'NONE', *, *, #48877, .F. ) ;
#12089=ORIENTED_EDGE ( 'NONE', *, *, #79684, .T. ) ;
#12090=ADVANCED_FACE ( 'NONE', ( #38954 ), #32623, .F. ) ;
#12112=ORIENTED_EDGE ( 'NONE', *, *, #40665, .T. ) ;
#12117=FACE_OUTER_BOUND ( 'NONE', #57303, .T. ) ;
#12121=FACE_OUTER_BOUND ( 'NONE', #27381, .T. ) ;
#12157=CARTESIAN_POINT ( 'NONE',  ( -15.12820512820512953, -7.500000000000000000, 29.75000000000000355 ) ) ;
#12158=ORIENTED_EDGE ( 'NONE', *, *, #19215, .T. ) ;
#12160=FACE_OUTER_BOUND ( 'NONE', #64616, .T. ) ;
#12161=ORIENTED_EDGE ( 'NONE', *, *, #17333, .F. ) ;
#12162=VECTOR ( 'NONE', #53311, 1000.000000000000000 ) ;
#12168=ORIENTED_EDGE ( 'NONE', *, *, #3302, .T. ) ;
#12176=CARTESIAN_POINT ( 'NONE',  ( -19.50000000000000000, -3.499999999999999556, 29.75000000000000355 ) ) ;
#12183=ADVANCED_FACE ( 'NONE', ( #68627 ), #20878, .F. ) ;
#12188=VECTOR ( 'NONE', #46473, 1000.000000000000000 ) ;
#12190=LINE ( 'NONE', #85624, #29554 ) ;
#12195=ORIENTED_EDGE ( 'NONE', *, *, #72553, .T. ) ;
#12204=DIRECTION ( 'NONE',  ( -1.000000000000000000, -0.000000000000000000, -0.000000000000000000 ) ) ;
#12208=LINE ( 'NONE', #82889, #14571 ) ;
#12230=VERTEX_POINT ( 'NONE', #33953 ) ;
#12233=DIRECTION ( 'NONE',  ( -0.000000000000000000, 1.000000000000000000, -0.000000000000000000 ) ) ;
#12249=DIRECTION ( 'NONE',  ( -1.000000000000000000, 0.000000000000000000, -0.000000000000000000 ) ) ;
#12251=LINE ( 'NONE', #67204, #69275 ) ;
#12256=ADVANCED_FACE ( 'NONE', ( #1506 ), #48793, .T. ) ;
#12258=CARTESIAN_POINT ( 'NONE',  ( -19.50000000000000000, -3.499999999999999556, 29.75000000000000355 ) ) ;
#12265=CARTESIAN_POINT ( 'NONE',  ( -9.320512820512821150, -4.000000000000000000, 29.65000000000000213 ) ) ;
#12277=VECTOR ( 'NONE', #5774, 1000.000000000000000 ) ;
#12281=EDGE_CURVE ( 'NONE', #61882, #11602, #54656, .T. ) ;
#12284=FACE_OUTER_BOUND ( 'NONE', #27778, .T. ) ;
#12298=VECTOR ( 'NONE', #59644, 1000.000000000000000 ) ;
#12312=DIRECTION ( 'NONE',  ( -1.000000000000000000, 0.000000000000000000, -0.000000000000000000 ) ) ;
#12313=ORIENTED_EDGE ( 'NONE', *, *, #7677, .F. ) ;
#12320=CARTESIAN_POINT ( 'NONE',  ( 11.25641025641025550, -7.500000000000000000, 33.75000000000000000 ) ) ;
#12329=DIRECTION ( 'NONE',  ( -0.000000000000000000, 1.000000000000000000, -0.000000000000000000 ) ) ;
#12332=VECTOR ( 'NONE', #58522, 1000.000000000000000 ) ;
#12340=ORIENTED_EDGE ( 'NONE', *, *, #78372, .F. ) ;
#12348=CARTESIAN_POINT ( 'NONE',  ( 20.00000000000000000, -4.000000000000000000, 29.75000000000000355 ) ) ;
#12361=CARTESIAN_POINT ( 'NONE',  ( -19.50000000000000000, -3.499999999999999556, 29.75000000000000355 ) ) ;
#12369=LINE ( 'NONE', #6058, #27235 ) ;
#12380=CARTESIAN_POINT ( 'NONE',  ( 0.000000000000000000, -11.00000000000000000, 28.75000000000000000 ) ) ;
#12384=CARTESIAN_POINT ( 'NONE',  ( -2.294871794871794712, -3.499999999999999556, 29.75000000000000355 ) ) ;
#12389=CARTESIAN_POINT ( 'NONE',  ( 9.320512820512821150, -7.500000000000000000, 29.75000000000000355 ) ) ;
#12397=VECTOR ( 'NONE', #25543, 1000.000000000000000 ) ;
#12401=ORIENTED_EDGE ( 'NONE', *, *, #27038, .F. ) ;
#12405=EDGE_CURVE ( 'NONE', #80094, #22635, #30423, .T. ) ;
#12410=LINE ( 'NONE', #11525, #55174 ) ;
#12440=DIRECTION ( 'NONE',  ( -0.000000000000000000, 1.000000000000000000, -0.000000000000000000 ) ) ;
#12441=CARTESIAN_POINT ( 'NONE',  ( 9.320512820512821150, -3.499999999999999556, 29.75000000000000355 ) ) ;
#12447=DIRECTION ( 'NONE',  ( 0.000000000000000000, 0.000000000000000000, -1.000000000000000000 ) ) ;
#12463=VERTEX_POINT ( 'NONE', #66300 ) ;
#12469=ADVANCED_FACE ( 'NONE', ( #4603 ), #45136, .T. ) ;
#12488=DIRECTION ( 'NONE',  ( 0.000000000000000000, 0.000000000000000000, -1.000000000000000000 ) ) ;
#12499=CARTESIAN_POINT ( 'NONE',  ( -9.070512820512819374, -7.500000000000000000, 33.75000000000000000 ) ) ;
#12500=LINE ( 'NONE', #47607, #21112 ) ;
#12516=CARTESIAN_POINT ( 'NONE',  ( 11.00641025641025550, -3.499999999999999556, 29.75000000000000355 ) ) ;
#12520=LINE ( 'NONE', #6216, #81312 ) ;
#12531=CARTESIAN_POINT ( 'NONE',  ( 20.00000000000000000, -4.000000000000000000, 29.75000000000000355 ) ) ;
#12551=VERTEX_POINT ( 'NONE', #20777 ) ;
#12557=LINE ( 'NONE', #5356, #12650 ) ;
#12567=ORIENTED_EDGE ( 'NONE', *, *, #37856, .F. ) ;
#12570=CARTESIAN_POINT ( 'NONE',  ( -9.070512820512819374, -7.500000000000000000, 29.75000000000000355 ) ) ;
#12585=DIRECTION ( 'NONE',  ( -0.000000000000000000, 1.000000000000000000, -0.000000000000000000 ) ) ;
#12586=EDGE_CURVE ( 'NONE', #44505, #54542, #55449, .T. ) ;
#12595=VECTOR ( 'NONE', #25604, 1000.000000000000000 ) ;
#12620=CARTESIAN_POINT ( 'NONE',  ( -1.326923076923076872, -7.500000000000000000, 33.75000000000000000 ) ) ;
#12630=PLANE ( 'NONE',  #77521 ) ;
#12632=VECTOR ( 'NONE', #43172, 1000.000000000000000 ) ;
#12637=ORIENTED_EDGE ( 'NONE', *, *, #59833, .F. ) ;
#12646=LINE ( 'NONE', #21164, #24085 ) ;
#12648=DIRECTION ( 'NONE',  ( -0.000000000000000000, 0.000000000000000000, 1.000000000000000000 ) ) ;
#12650=VECTOR ( 'NONE', #38246, 1000.000000000000000 ) ;
#12651=DIRECTION ( 'NONE',  ( -0.000000000000000000, 1.000000000000000000, -0.000000000000000000 ) ) ;
#12670=ORIENTED_EDGE ( 'NONE', *, *, #28655, .F. ) ;
#12675=ORIENTED_EDGE ( 'NONE', *, *, #52809, .F. ) ;
#12676=DIRECTION ( 'NONE',  ( 0.000000000000000000, 0.000000000000000000, -1.000000000000000000 ) ) ;
#12684=ORIENTED_EDGE ( 'NONE', *, *, #60417, .F. ) ;
#12686=FACE_OUTER_BOUND ( 'NONE', #3871, .T. ) ;
#12699=VECTOR ( 'NONE', #58234, 1000.000000000000000 ) ;
#12704=CARTESIAN_POINT ( 'NONE',  ( -9.320512820512821150, -4.000000000000000000, 29.25000000000000000 ) ) ;
#12706=EDGE_LOOP ( 'NONE', ( #32954, #14510, #35927, #85228 ) ) ;
#12712=ORIENTED_EDGE ( 'NONE', *, *, #44209, .F. ) ;
#12714=ORIENTED_EDGE ( 'NONE', *, *, #12768, .F. ) ;
#12734=CYLINDRICAL_SURFACE ( 'NONE', #9050, 4.000000000000000000 ) ;
#12745=DIRECTION ( 'NONE',  ( -0.000000000000000000, 0.000000000000000000, 1.000000000000000000 ) ) ;
#12746=LINE ( 'NONE', #46094, #83955 ) ;
#12749=ORIENTED_EDGE ( 'NONE', *, *, #60356, .T. ) ;
#12755=LINE ( 'NONE', #54173, #46291 ) ;
#12758=DIRECTION ( 'NONE',  ( -1.000000000000000000, -0.000000000000000000, -0.000000000000000000 ) ) ;
#12768=EDGE_CURVE ( 'NONE', #80730, #82878, #25214, .T. ) ;
#12771=DIRECTION ( 'NONE',  ( 0.000000000000000000, -1.000000000000000000, 0.000000000000000000 ) ) ;
#12794=AXIS2_PLACEMENT_3D ( 'NONE', #3998, #65258, #64808 ) ;
#12809=DIRECTION ( 'NONE',  ( -0.000000000000000000, 1.000000000000000000, -0.000000000000000000 ) ) ;
#12819=ORIENTED_EDGE ( 'NONE', *, *, #81031, .T. ) ;
#12824=DIRECTION ( 'NONE',  ( 1.000000000000000000, 0.000000000000000000, 0.000000000000000000 ) ) ;
#12827=LINE ( 'NONE', #4749, #86665 ) ;
#12833=ORIENTED_EDGE ( 'NONE', *, *, #82525, .T. ) ;
#12835=CIRCLE ( 'NONE', #9993, 4.000000000000000000 ) ;
#12836=PLANE ( 'NONE',  #51485 ) ;
#12841=ORIENTED_EDGE ( 'NONE', *, *, #79709, .F. ) ;
#12849=CARTESIAN_POINT ( 'NONE',  ( 20.00000000000000000, -4.000000000000000000, 29.75000000000000355 ) ) ;
#12869=ADVANCED_FACE ( 'NONE', ( #83611 ), #15141, .T. ) ;
#12871=ORIENTED_EDGE ( 'NONE', *, *, #36613, .T. ) ;
#12892=CARTESIAN_POINT ( 'NONE',  ( 8.102564102564102200, -4.000000000000000000, 29.75000000000000355 ) ) ;
#12905=AXIS2_PLACEMENT_3D ( 'NONE', #25639, #53545, #20217 ) ;
#12909=CARTESIAN_POINT ( 'NONE',  ( 0.000000000000000000, -11.00000000000000000, 29.75000000000000355 ) ) ;
#12927=DIRECTION ( 'NONE',  ( 1.000000000000000000, 0.000000000000000000, 0.000000000000000000 ) ) ;
#12929=VERTEX_POINT ( 'NONE', #41726 ) ;
#12931=EDGE_CURVE ( 'NONE', #5154, #46042, #49365, .T. ) ;
#12934=ORIENTED_EDGE ( 'NONE', *, *, #44903, .T. ) ;
#12937=DIRECTION ( 'NONE',  ( -1.000000000000000000, -0.000000000000000000, 0.000000000000000000 ) ) ;
#12939=ORIENTED_EDGE ( 'NONE', *, *, #73718, .T. ) ;
#12949=ORIENTED_EDGE ( 'NONE', *, *, #4551, .F. ) ;
#12956=CARTESIAN_POINT ( 'NONE',  ( 15.12820512820512953, -3.499999999999999556, 29.75000000000000355 ) ) ;
#12959=VECTOR ( 'NONE', #4357, 1000.000000000000000 ) ;
#12967=AXIS2_PLACEMENT_3D ( 'NONE', #30029, #37665, #76891 ) ;
#12969=ORIENTED_EDGE ( 'NONE', *, *, #63442, .T. ) ;
#12979=CARTESIAN_POINT ( 'NONE',  ( -14.87820512820512953, -7.500000000000000000, 29.75000000000000355 ) ) ;
#12990=DIRECTION ( 'NONE',  ( -0.000000000000000000, 0.000000000000000000, 1.000000000000000000 ) ) ;
#13025=EDGE_CURVE ( 'NONE', #32479, #80662, #65078, .T. ) ;
#13044=PLANE ( 'NONE',  #66457 ) ;
#13060=LINE ( 'NONE', #88737, #54840 ) ;
#13066=CARTESIAN_POINT ( 'NONE',  ( -8.352564102564102200, -7.500000000000000000, 33.75000000000000000 ) ) ;
#13067=ORIENTED_EDGE ( 'NONE', *, *, #20037, .F. ) ;
#13094=DIRECTION ( 'NONE',  ( -1.000000000000000000, -0.000000000000000000, -0.000000000000000000 ) ) ;
#13100=DIRECTION ( 'NONE',  ( -0.000000000000000000, 1.000000000000000000, -0.000000000000000000 ) ) ;
#13118=VERTEX_POINT ( 'NONE', #39419 ) ;
#13132=VECTOR ( 'NONE', #82955, 1000.000000000000000 ) ;
#13142=EDGE_CURVE ( 'NONE', #19996, #17369, #6067, .T. ) ;
#13158=CARTESIAN_POINT ( 'NONE',  ( 20.00000000000000000, -4.000000000000000000, 29.75000000000000355 ) ) ;
#13160=VERTEX_POINT ( 'NONE', #27215 ) ;
#13167=VECTOR ( 'NONE', #12585, 1000.000000000000000 ) ;
#13174=VERTEX_POINT ( 'NONE', #75406 ) ;
#13180=CARTESIAN_POINT ( 'NONE',  ( -7.384615384615385025, -4.000000000000000000, 29.75000000000000355 ) ) ;
#13193=DIRECTION ( 'NONE',  ( 1.000000000000000000, 0.000000000000000000, 0.000000000000000000 ) ) ;
#13202=EDGE_LOOP ( 'NONE', ( #5124, #37956, #67610, #59324, #4652 ) ) ;
#13211=CARTESIAN_POINT ( 'NONE',  ( 20.00000000000000000, -3.499999999999999556, 28.25000000000000000 ) ) ;
#13221=ORIENTED_EDGE ( 'NONE', *, *, #10311, .F. ) ;
#13224=CARTESIAN_POINT ( 'NONE',  ( -19.50000000000000000, -3.499999999999999556, 29.75000000000000355 ) ) ;
#13234=ORIENTED_EDGE ( 'NONE', *, *, #2287, .F. ) ;
#13235=LINE ( 'NONE', #81698, #24142 ) ;
#13246=DIRECTION ( 'NONE',  ( 0.000000000000000000, 0.000000000000000000, -1.000000000000000000 ) ) ;
#13248=ORIENTED_EDGE ( 'NONE', *, *, #37353, .F. ) ;
#13258=LINE ( 'NONE', #81726, #8036 ) ;
#13259=VECTOR ( 'NONE', #78017, 1000.000000000000000 ) ;
#13262=DIRECTION ( 'NONE',  ( -1.000000000000000000, -0.000000000000000000, -0.000000000000000000 ) ) ;
#13272=DIRECTION ( 'NONE',  ( 0.000000000000000000, 0.000000000000000000, -1.000000000000000000 ) ) ;
#13274=EDGE_LOOP ( 'NONE', ( #71321, #36383, #30231, #80298 ) ) ;
#13278=AXIS2_PLACEMENT_3D ( 'NONE', #44543, #3122, #24280 ) ;
#13285=AXIS2_PLACEMENT_3D ( 'NONE', #73659, #75417, #13711 ) ;
#13287=ORIENTED_EDGE ( 'NONE', *, *, #25012, .T. ) ;
#13316=EDGE_CURVE ( 'NONE', #53642, #45062, #57803, .T. ) ;
#13318=EDGE_LOOP ( 'NONE', ( #68055, #11750, #35082, #44569 ) ) ;
#13328=DIRECTION ( 'NONE',  ( 1.000000000000000000, 0.000000000000000000, 0.000000000000000000 ) ) ;
#13340=ORIENTED_EDGE ( 'NONE', *, *, #38918, .F. ) ;
#13358=EDGE_CURVE ( 'NONE', #75410, #63745, #29443, .T. ) ;
#13367=CARTESIAN_POINT ( 'NONE',  ( 13.19230769230769340, -7.500000000000000000, 29.75000000000000355 ) ) ;
#13374=AXIS2_PLACEMENT_3D ( 'NONE', #62320, #634, #61437 ) ;
#13381=ORIENTED_EDGE ( 'NONE', *, *, #51107, .T. ) ;
#13382=EDGE_CURVE ( 'NONE', #17730, #34333, #85265, .T. ) ;
#13385=EDGE_CURVE ( 'NONE', #38776, #33822, #36634, .T. ) ;
#13394=VERTEX_POINT ( 'NONE', #1957 ) ;
#13398=AXIS2_PLACEMENT_3D ( 'NONE', #23250, #79545, #25034 ) ;
#13405=ORIENTED_EDGE ( 'NONE', *, *, #32911, .T. ) ;
#13407=CARTESIAN_POINT ( 'NONE',  ( 3.262820512820510999, -7.500000000000000000, 33.75000000000000000 ) ) ;
#13411=CARTESIAN_POINT ( 'NONE',  ( -2.294871794871794712, -7.500000000000000000, 29.75000000000000355 ) ) ;
#13426=ORIENTED_EDGE ( 'NONE', *, *, #17456, .T. ) ;
#13430=ORIENTED_EDGE ( 'NONE', *, *, #23135, .T. ) ;
#13442=LINE ( 'NONE', #47673, #49649 ) ;
#13446=EDGE_LOOP ( 'NONE', ( #86883, #59901, #76602, #31099 ) ) ;
#13473=EDGE_CURVE ( 'NONE', #66098, #34205, #33330, .T. ) ;
#13483=FACE_OUTER_BOUND ( 'NONE', #9413, .T. ) ;
#13515=DIRECTION ( 'NONE',  ( -1.000000000000000000, -0.000000000000000000, -0.000000000000000000 ) ) ;
#13523=CARTESIAN_POINT ( 'NONE',  ( 5.448717948717947124, -3.499999999999999556, 29.75000000000000355 ) ) ;
#13527=EDGE_CURVE ( 'NONE', #42531, #60579, #26663, .T. ) ;
#13532=CARTESIAN_POINT ( 'NONE',  ( -10.03846153846153832, -11.00000000000000000, 29.65000000000000213 ) ) ;
#13538=CARTESIAN_POINT ( 'NONE',  ( 9.320512820512821150, -7.500000000000000000, 33.75000000000000000 ) ) ;
#13542=DIRECTION ( 'NONE',  ( 0.000000000000000000, 0.000000000000000000, -1.000000000000000000 ) ) ;
#13549=EDGE_LOOP ( 'NONE', ( #32447, #55705, #63906, #42308 ) ) ;
#13563=LINE ( 'NONE', #41044, #24217 ) ;
#13567=CYLINDRICAL_SURFACE ( 'NONE', #48265, 0.5000000000000004441 ) ;
#13575=ORIENTED_EDGE ( 'NONE', *, *, #43956, .F. ) ;
#13599=CIRCLE ( 'NONE', #68243, 4.000000000000000000 ) ;
#13601=DIRECTION ( 'NONE',  ( -1.000000000000000000, 0.000000000000000000, -0.000000000000000000 ) ) ;
#13602=PLANE ( 'NONE',  #46970 ) ;
#13603=EDGE_LOOP ( 'NONE', ( #73712, #25816, #33241, #63253 ) ) ;
#13615=DIRECTION ( 'NONE',  ( 0.000000000000000000, 0.000000000000000000, 1.000000000000000000 ) ) ;
#13617=DIRECTION ( 'NONE',  ( -0.000000000000000000, 1.000000000000000000, -0.000000000000000000 ) ) ;
#13618=ORIENTED_EDGE ( 'NONE', *, *, #41041, .F. ) ;
#13621=VERTEX_POINT ( 'NONE', #9487 ) ;
#13633=EDGE_LOOP ( 'NONE', ( #65998, #29434, #46146, #13287 ) ) ;
#13634=EDGE_CURVE ( 'NONE', #51834, #30410, #85155, .T. ) ;
#13635=VERTEX_POINT ( 'NONE', #50030 ) ;
#13641=DIRECTION ( 'NONE',  ( 1.000000000000000000, 0.000000000000000000, 0.000000000000000000 ) ) ;
#13647=CARTESIAN_POINT ( 'NONE',  ( 18.75000000000000000, -7.500000000000000000, 29.75000000000000355 ) ) ;
#13657=LINE ( 'NONE', #41137, #46362 ) ;
#13660=VECTOR ( 'NONE', #26036, 1000.000000000000000 ) ;
#13667=EDGE_CURVE ( 'NONE', #22635, #51776, #84285, .T. ) ;
#13685=ORIENTED_EDGE ( 'NONE', *, *, #18414, .F. ) ;
#13692=CARTESIAN_POINT ( 'NONE',  ( 0.000000000000000000, -11.00000000000000000, 29.75000000000000355 ) ) ;
#13694=VECTOR ( 'NONE', #6700, 1000.000000000000000 ) ;
#13705=ORIENTED_EDGE ( 'NONE', *, *, #48185, .F. ) ;
#13711=DIRECTION ( 'NONE',  ( 1.000000000000000000, 0.000000000000000000, 0.000000000000000000 ) ) ;
#13713=CARTESIAN_POINT ( 'NONE',  ( 15.84615384615384670, -7.500000000000000000, 33.75000000000000000 ) ) ;
#13715=EDGE_CURVE ( 'NONE', #74633, #39901, #65315, .T. ) ;
#13727=FACE_OUTER_BOUND ( 'NONE', #54515, .T. ) ;
#13736=DIRECTION ( 'NONE',  ( -1.000000000000000000, 0.000000000000000000, -0.000000000000000000 ) ) ;
#13759=LINE ( 'NONE', #54295, #81614 ) ;
#13788=ORIENTED_EDGE ( 'NONE', *, *, #16391, .F. ) ;
#13803=ORIENTED_EDGE ( 'NONE', *, *, #27140, .F. ) ;
#13810=CARTESIAN_POINT ( 'NONE',  ( 15.84615384615384670, -11.00000000000000000, 29.75000000000000355 ) ) ;
#13827=DIRECTION ( 'NONE',  ( -1.000000000000000000, -0.000000000000000000, -0.000000000000000000 ) ) ;
#13838=DIRECTION ( 'NONE',  ( -1.000000000000000000, 0.000000000000000000, -0.000000000000000000 ) ) ;
#13841=CARTESIAN_POINT ( 'NONE',  ( -4.230769230769230838, -11.50000000000000000, 29.75000000000000355 ) ) ;
#13843=ORIENTED_EDGE ( 'NONE', *, *, #11489, .T. ) ;
#13868=FILL_AREA_STYLE_COLOUR ( '', #426 ) ;
#13901=LINE ( 'NONE', #88265, #13694 ) ;
#13927=EDGE_CURVE ( 'NONE', #61963, #53841, #75198, .T. ) ;
#13929=VERTEX_POINT ( 'NONE', #68427 ) ;
#13941=CARTESIAN_POINT ( 'NONE',  ( 16.09615384615384670, -7.500000000000000000, 29.75000000000000355 ) ) ;
#13946=CARTESIAN_POINT ( 'NONE',  ( -4.480769230769230838, -11.00000000000000000, 29.75000000000000355 ) ) ;
#13947=ORIENTED_EDGE ( 'NONE', *, *, #45451, .F. ) ;
#13953=EDGE_LOOP ( 'NONE', ( #74141, #45424, #51358, #23711 ) ) ;
#13957=CARTESIAN_POINT ( 'NONE',  ( 14.16025641025641235, -7.500000000000000000, 33.75000000000000000 ) ) ;
#13958=ORIENTED_EDGE ( 'NONE', *, *, #60991, .T. ) ;
#13960=EDGE_CURVE ( 'NONE', #43735, #3876, #83282, .T. ) ;
#13962=ORIENTED_EDGE ( 'NONE', *, *, #50612, .T. ) ;
#13965=CIRCLE ( 'NONE', #26970, 0.5000000000000004441 ) ;
#13973=VECTOR ( 'NONE', #65644, 1000.000000000000000 ) ;
#13978=EDGE_CURVE ( 'NONE', #13635, #44538, #857, .T. ) ;
#13979=CARTESIAN_POINT ( 'NONE',  ( 11.97435897435897267, -3.499999999999999556, 29.75000000000000355 ) ) ;
#13996=DIRECTION ( 'NONE',  ( -1.000000000000000000, -0.000000000000000000, -0.000000000000000000 ) ) ;
#14003=DIRECTION ( 'NONE',  ( -1.000000000000000000, 0.000000000000000000, -0.000000000000000000 ) ) ;
#14005=DIRECTION ( 'NONE',  ( 1.000000000000000000, 0.000000000000000000, 0.000000000000000000 ) ) ;
#14009=PLANE ( 'NONE',  #9430 ) ;
#14015=EDGE_CURVE ( 'NONE', #51615, #78324, #30538, .T. ) ;
#14022=CARTESIAN_POINT ( 'NONE',  ( 8.352564102564102200, -3.499999999999999556, 29.75000000000000355 ) ) ;
#14041=FACE_OUTER_BOUND ( 'NONE', #70911, .T. ) ;
#14043=ORIENTED_EDGE ( 'NONE', *, *, #26033, .F. ) ;
#14045=CIRCLE ( 'NONE', #15473, 4.000000000000000000 ) ;
#14056=AXIS2_PLACEMENT_3D ( 'NONE', #86224, #11436, #24048 ) ;
#14063=ORIENTED_EDGE ( 'NONE', *, *, #34417, .F. ) ;
#14074=EDGE_CURVE ( 'NONE', #4690, #42018, #7534, .T. ) ;
#14091=ORIENTED_EDGE ( 'NONE', *, *, #17401, .T. ) ;
#14099=AXIS2_PLACEMENT_3D ( 'NONE', #2116, #31366, #64690 ) ;
#14104=LINE ( 'NONE', #14547, #57645 ) ;
#14110=EDGE_CURVE ( 'NONE', #58603, #49729, #11647, .T. ) ;
#14129=VECTOR ( 'NONE', #72259, 1000.000000000000000 ) ;
#14132=VERTEX_POINT ( 'NONE', #5294 ) ;
#14138=VECTOR ( 'NONE', #44163, 1000.000000000000000 ) ;
#14174=VERTEX_POINT ( 'NONE', #58897 ) ;
#14178=PLANE ( 'NONE',  #53775 ) ;
#14182=LINE ( 'NONE', #75884, #62434 ) ;
#14209=EDGE_CURVE ( 'NONE', #73790, #26695, #31433, .T. ) ;
#14254=AXIS2_PLACEMENT_3D ( 'NONE', #27796, #48058, #13838 ) ;
#14271=CARTESIAN_POINT ( 'NONE',  ( 14.87820512820512953, -3.499999999999999556, 29.75000000000000355 ) ) ;
#14280=ORIENTED_EDGE ( 'NONE', *, *, #67022, .T. ) ;
#14292=ORIENTED_EDGE ( 'NONE', *, *, #66998, .F. ) ;
#14301=DIRECTION ( 'NONE',  ( 0.000000000000000000, 0.000000000000000000, 1.000000000000000000 ) ) ;
#14302=ORIENTED_EDGE ( 'NONE', *, *, #12281, .F. ) ;
#14317=VECTOR ( 'NONE', #82505, 1000.000000000000000 ) ;
#14319=CARTESIAN_POINT ( 'NONE',  ( 16.81410256410256565, -7.500000000000000000, 33.75000000000000000 ) ) ;
#14335=ORIENTED_EDGE ( 'NONE', *, *, #64595, .T. ) ;
#14373=ORIENTED_EDGE ( 'NONE', *, *, #59451, .F. ) ;
#14378=ORIENTED_EDGE ( 'NONE', *, *, #86712, .F. ) ;
#14395=LINE ( 'NONE', #25809, #85529 ) ;
#14397=ORIENTED_EDGE ( 'NONE', *, *, #51107, .F. ) ;
#14402=ORIENTED_EDGE ( 'NONE', *, *, #88083, .F. ) ;
#14428=EDGE_CURVE ( 'NONE', #17730, #34055, #49813, .T. ) ;
#14438=ADVANCED_FACE ( 'NONE', ( #63329 ), #77290, .T. ) ;
#14439=AXIS2_PLACEMENT_3D ( 'NONE', #62698, #76678, #28949 ) ;
#14447=DIRECTION ( 'NONE',  ( 1.000000000000000000, 0.000000000000000000, 0.000000000000000000 ) ) ;
#14458=CARTESIAN_POINT ( 'NONE',  ( -7.134615384615385025, -7.500000000000000000, 29.75000000000000355 ) ) ;
#14466=ORIENTED_EDGE ( 'NONE', *, *, #8495, .T. ) ;
#14470=DIRECTION ( 'NONE',  ( -0.000000000000000000, 1.000000000000000000, -0.000000000000000000 ) ) ;
#14481=EDGE_LOOP ( 'NONE', ( #13248, #43194, #49056, #48719 ) ) ;
#14492=DIRECTION ( 'NONE',  ( 1.000000000000000000, 0.000000000000000000, 0.000000000000000000 ) ) ;
#14501=DIRECTION ( 'NONE',  ( -1.000000000000000000, -0.000000000000000000, -0.000000000000000000 ) ) ;
#14509=LINE ( 'NONE', #69455, #57708 ) ;
#14510=ORIENTED_EDGE ( 'NONE', *, *, #29458, .T. ) ;
#14540=AXIS2_PLACEMENT_3D ( 'NONE', #39967, #20996, #75955 ) ;
#14546=CARTESIAN_POINT ( 'NONE',  ( 15.12820512820512953, -11.50000000000000000, 29.75000000000000355 ) ) ;
#14547=CARTESIAN_POINT ( 'NONE',  ( 0.000000000000000000, -11.00000000000000000, 29.75000000000000355 ) ) ;
#14548=EDGE_CURVE ( 'NONE', #955, #88209, #74875, .T. ) ;
#14571=VECTOR ( 'NONE', #13094, 1000.000000000000000 ) ;
#14628=DIRECTION ( 'NONE',  ( 0.000000000000000000, 0.000000000000000000, 1.000000000000000000 ) ) ;
#14637=CARTESIAN_POINT ( 'NONE',  ( -10.03846153846153832, -7.500000000000000000, 29.75000000000000355 ) ) ;
#14642=EDGE_LOOP ( 'NONE', ( #18236, #31004, #48621, #74126 ) ) ;
#14653=EDGE_CURVE ( 'NONE', #78266, #64241, #48267, .T. ) ;
#14657=ORIENTED_EDGE ( 'NONE', *, *, #51565, .F. ) ;
#14689=CARTESIAN_POINT ( 'NONE',  ( -19.50000000000000000, -3.499999999999999556, 29.75000000000000355 ) ) ;
#14695=LINE ( 'NONE', #76846, #14799 ) ;
#14723=LINE ( 'NONE', #41310, #56580 ) ;
#14724=CARTESIAN_POINT ( 'NONE',  ( 14.87820512820512953, -4.000000000000000000, 29.75000000000000355 ) ) ;
#14727=EDGE_CURVE ( 'NONE', #45168, #54472, #35657, .T. ) ;
#14759=DIRECTION ( 'NONE',  ( -1.000000000000000000, 0.000000000000000000, -0.000000000000000000 ) ) ;
#14762=AXIS2_PLACEMENT_3D ( 'NONE', #25358, #36759, #78630 ) ;
#14767=PLANE ( 'NONE',  #29169 ) ;
#14772=FACE_OUTER_BOUND ( 'NONE', #79976, .T. ) ;
#14782=DIRECTION ( 'NONE',  ( -0.000000000000000000, 1.000000000000000000, -0.000000000000000000 ) ) ;
#14790=CARTESIAN_POINT ( 'NONE',  ( -0.3589743589743593088, -7.500000000000000000, 29.75000000000000355 ) ) ;
#14799=VECTOR ( 'NONE', #78164, 1000.000000000000000 ) ;
#14804=CIRCLE ( 'NONE', #56511, 4.000000000000000000 ) ;
#14818=ORIENTED_EDGE ( 'NONE', *, *, #44361, .T. ) ;
#14824=FACE_OUTER_BOUND ( 'NONE', #80704, .T. ) ;
#14826=DIRECTION ( 'NONE',  ( -1.000000000000000000, -0.000000000000000000, -0.000000000000000000 ) ) ;
#14828=EDGE_CURVE ( 'NONE', #64401, #74021, #58564, .T. ) ;
#14834=VERTEX_POINT ( 'NONE', #78397 ) ;
#14850=EDGE_CURVE ( 'NONE', #82495, #71093, #43727, .T. ) ;
#14859=ORIENTED_EDGE ( 'NONE', *, *, #54658, .T. ) ;
#14862=ORIENTED_EDGE ( 'NONE', *, *, #65778, .F. ) ;
#14869=DIRECTION ( 'NONE',  ( 0.000000000000000000, 0.000000000000000000, -1.000000000000000000 ) ) ;
#14872=LINE ( 'NONE', #42346, #10123 ) ;
#14885=CARTESIAN_POINT ( 'NONE',  ( -19.50000000000000000, -3.499999999999999556, 29.75000000000000355 ) ) ;
#14906=ORIENTED_EDGE ( 'NONE', *, *, #47763, .T. ) ;
#14924=ORIENTED_EDGE ( 'NONE', *, *, #23135, .F. ) ;
#14927=LINE ( 'NONE', #68972, #70395 ) ;
#14935=EDGE_LOOP ( 'NONE', ( #81151, #74893, #53573, #21298 ) ) ;
#14945=DIRECTION ( 'NONE',  ( -1.000000000000000000, 0.000000000000000000, -0.000000000000000000 ) ) ;
#14949=ORIENTED_EDGE ( 'NONE', *, *, #39053, .T. ) ;
#14959=CARTESIAN_POINT ( 'NONE',  ( 18.03205128205128105, -7.500000000000000000, 29.75000000000000355 ) ) ;
#14962=ORIENTED_EDGE ( 'NONE', *, *, #45241, .T. ) ;
#14964=DIRECTION ( 'NONE',  ( -0.000000000000000000, 1.000000000000000000, -0.000000000000000000 ) ) ;
#14967=FACE_OUTER_BOUND ( 'NONE', #11744, .T. ) ;
#14996=DIRECTION ( 'NONE',  ( -1.000000000000000000, -0.000000000000000000, -0.000000000000000000 ) ) ;
#14999=ORIENTED_EDGE ( 'NONE', *, *, #56784, .T. ) ;
#15008=CARTESIAN_POINT ( 'NONE',  ( 10.03846153846153832, -7.500000000000000000, 29.75000000000000355 ) ) ;
#15028=EDGE_CURVE ( 'NONE', #6548, #6628, #46399, .T. ) ;
#15052=AXIS2_PLACEMENT_3D ( 'NONE', #80938, #59757, #87253 ) ;
#15060=FACE_OUTER_BOUND ( 'NONE', #85986, .T. ) ;
#15081=VERTEX_POINT ( 'NONE', #55808 ) ;
#15086=PLANE ( 'NONE',  #25902 ) ;
#15098=CARTESIAN_POINT ( 'NONE',  ( 20.00000000000000000, -4.000000000000000000, 28.25000000000000000 ) ) ;
#15113=DIRECTION ( 'NONE',  ( 0.000000000000000000, 0.000000000000000000, -1.000000000000000000 ) ) ;
#15116=DIRECTION ( 'NONE',  ( 0.000000000000000000, 0.000000000000000000, -1.000000000000000000 ) ) ;
#15130=DIRECTION ( 'NONE',  ( -1.000000000000000000, -0.000000000000000000, -0.000000000000000000 ) ) ;
#15133=EDGE_CURVE ( 'NONE', #25570, #3292, #13060, .T. ) ;
#15140=VECTOR ( 'NONE', #55419, 1000.000000000000000 ) ;
#15141=PLANE ( 'NONE',  #76525 ) ;
#15157=ORIENTED_EDGE ( 'NONE', *, *, #40029, .T. ) ;
#15158=ORIENTED_EDGE ( 'NONE', *, *, #25373, .T. ) ;
#15169=ORIENTED_EDGE ( 'NONE', *, *, #79709, .T. ) ;
#15173=ORIENTED_EDGE ( 'NONE', *, *, #85750, .F. ) ;
#15186=DIRECTION ( 'NONE',  ( 0.000000000000000000, 0.000000000000000000, 1.000000000000000000 ) ) ;
#15190=CARTESIAN_POINT ( 'NONE',  ( 4.480769230769229061, -3.499999999999999556, 29.75000000000000355 ) ) ;
#15208=LINE ( 'NONE', #76010, #41967 ) ;
#15211=AXIS2_PLACEMENT_3D ( 'NONE', #54846, #81003, #19293 ) ;
#15217=LINE ( 'NONE', #70148, #37510 ) ;
#15235=DIRECTION ( 'NONE',  ( 0.000000000000000000, 0.000000000000000000, -1.000000000000000000 ) ) ;
#15246=LINE ( 'NONE', #21093, #85751 ) ;
#15249=ORIENTED_EDGE ( 'NONE', *, *, #80652, .T. ) ;
#15256=CARTESIAN_POINT ( 'NONE',  ( -1.326923076923076872, -7.500000000000000000, 29.75000000000000355 ) ) ;
#15267=DIRECTION ( 'NONE',  ( 0.000000000000000000, 0.000000000000000000, -1.000000000000000000 ) ) ;
#15271=EDGE_CURVE ( 'NONE', #14174, #38958, #54916, .T. ) ;
#15288=VERTEX_POINT ( 'NONE', #57384 ) ;
#15298=EDGE_LOOP ( 'NONE', ( #72685, #86643, #75432, #58886, #49251 ) ) ;
#15301=ORIENTED_EDGE ( 'NONE', *, *, #19197, .T. ) ;
#15306=DIRECTION ( 'NONE',  ( 1.000000000000000000, 0.000000000000000000, 0.000000000000000000 ) ) ;
#15313=ADVANCED_FACE ( 'NONE', ( #28142 ), #55612, .T. ) ;
#15324=AXIS2_PLACEMENT_3D ( 'NONE', #6497, #61424, #55556 ) ;
#15336=FACE_OUTER_BOUND ( 'NONE', #56504, .T. ) ;
#15341=DIRECTION ( 'NONE',  ( 0.000000000000000000, 0.000000000000000000, -1.000000000000000000 ) ) ;
#15342=CARTESIAN_POINT ( 'NONE',  ( 12.22435897435897267, -3.499999999999999556, 29.75000000000000355 ) ) ;
#15358=EDGE_CURVE ( 'NONE', #88209, #81743, #87110, .T. ) ;
#15367=ORIENTED_EDGE ( 'NONE', *, *, #6860, .F. ) ;
#15369=CIRCLE ( 'NONE', #65671, 4.000000000000000000 ) ;
#15380=ORIENTED_EDGE ( 'NONE', *, *, #12931, .F. ) ;
#15391=PLANE ( 'NONE',  #65588 ) ;
#15423=ORIENTED_EDGE ( 'NONE', *, *, #11405, .F. ) ;
#15434=CIRCLE ( 'NONE', #45577, 4.000000000000000000 ) ;
#15438=VERTEX_POINT ( 'NONE', #12320 ) ;
#15446=DIRECTION ( 'NONE',  ( -1.000000000000000000, -0.000000000000000000, -0.000000000000000000 ) ) ;
#15460=EDGE_CURVE ( 'NONE', #78324, #63745, #12755, .T. ) ;
#15473=AXIS2_PLACEMENT_3D ( 'NONE', #28764, #55773, #40945 ) ;
#15491=DIRECTION ( 'NONE',  ( 0.000000000000000000, 0.000000000000000000, -1.000000000000000000 ) ) ;
#15493=ORIENTED_EDGE ( 'NONE', *, *, #47371, .F. ) ;
#15494=DIRECTION ( 'NONE',  ( -0.000000000000000000, 1.000000000000000000, -0.000000000000000000 ) ) ;
#15498=ORIENTED_EDGE ( 'NONE', *, *, #17958, .T. ) ;
#15501=VERTEX_POINT ( 'NONE', #60051 ) ;
#15511=EDGE_LOOP ( 'NONE', ( #84473, #6540, #51977, #21323, #16006 ) ) ;
#15518=LINE ( 'NONE', #76322, #10697 ) ;
#15519=AXIS2_PLACEMENT_3D ( 'NONE', #42739, #34646, #20683 ) ;
#15531=ORIENTED_EDGE ( 'NONE', *, *, #66560, .T. ) ;
#15543=DIRECTION ( 'NONE',  ( 1.000000000000000000, 0.000000000000000000, 0.000000000000000000 ) ) ;
#15546=ORIENTED_EDGE ( 'NONE', *, *, #21182, .T. ) ;
#15549=CARTESIAN_POINT ( 'NONE',  ( -19.50000000000000000, -3.499999999999999556, 29.75000000000000355 ) ) ;
#15550=DIRECTION ( 'NONE',  ( 0.000000000000000000, -0.000000000000000000, 1.000000000000000000 ) ) ;
#15551=CARTESIAN_POINT ( 'NONE',  ( 15.12820512820512953, -7.500000000000000000, 33.75000000000000000 ) ) ;
#15554=CARTESIAN_POINT ( 'NONE',  ( 5.198717948717946236, -3.499999999999999556, 29.75000000000000355 ) ) ;
#15568=ORIENTED_EDGE ( 'NONE', *, *, #63439, .T. ) ;
#15588=CARTESIAN_POINT ( 'NONE',  ( 20.00000000000000000, -4.000000000000000000, 28.25000000000000000 ) ) ;
#15589=ORIENTED_EDGE ( 'NONE', *, *, #34738, .T. ) ;
#15614=EDGE_LOOP ( 'NONE', ( #63496, #38183, #28176, #27077 ) ) ;
#15621=DIRECTION ( 'NONE',  ( 0.000000000000000000, 0.000000000000000000, 1.000000000000000000 ) ) ;
#15630=LINE ( 'NONE', #15190, #21995 ) ;
#15636=DIRECTION ( 'NONE',  ( -0.000000000000000000, 1.000000000000000000, -0.000000000000000000 ) ) ;
#15641=DIRECTION ( 'NONE',  ( 0.000000000000000000, 0.000000000000000000, 1.000000000000000000 ) ) ;
#15646=EDGE_CURVE ( 'NONE', #27448, #34293, #48752, .T. ) ;
#15653=ORIENTED_EDGE ( 'NONE', *, *, #54841, .F. ) ;
#15655=LINE ( 'NONE', #83682, #51581 ) ;
#15674=EDGE_CURVE ( 'NONE', #16624, #40595, #57729, .T. ) ;
#15680=CARTESIAN_POINT ( 'NONE',  ( -5.448717948717948012, -7.500000000000000000, 29.75000000000000355 ) ) ;
#15685=DIRECTION ( 'NONE',  ( -0.000000000000000000, 1.000000000000000000, -0.000000000000000000 ) ) ;
#15692=DIRECTION ( 'NONE',  ( 1.000000000000000000, 0.000000000000000000, 0.000000000000000000 ) ) ;
#15696=DIRECTION ( 'NONE',  ( 0.000000000000000000, 0.000000000000000000, 1.000000000000000000 ) ) ;
#15702=DIRECTION ( 'NONE',  ( 0.000000000000000000, 0.000000000000000000, -1.000000000000000000 ) ) ;
#15711=EDGE_CURVE ( 'NONE', #72244, #45222, #72571, .T. ) ;
#15714=VERTEX_POINT ( 'NONE', #23490 ) ;
#15722=DIRECTION ( 'NONE',  ( 0.000000000000000000, 0.000000000000000000, -1.000000000000000000 ) ) ;
#15739=EDGE_LOOP ( 'NONE', ( #84316, #30961, #67274, #16814 ) ) ;
#15799=DIRECTION ( 'NONE',  ( 1.000000000000000000, 0.000000000000000000, 0.000000000000000000 ) ) ;
#15800=CARTESIAN_POINT ( 'NONE',  ( -9.320512820512821150, -4.000000000000000000, 29.75000000000000355 ) ) ;
#15821=PLANE ( 'NONE',  #52263 ) ;
#15822=VERTEX_POINT ( 'NONE', #87446 ) ;
#15824=EDGE_CURVE ( 'NONE', #7139, #77956, #54068, .T. ) ;
#15825=ORIENTED_EDGE ( 'NONE', *, *, #45812, .F. ) ;
#15828=ORIENTED_EDGE ( 'NONE', *, *, #62605, .T. ) ;
#15877=DIRECTION ( 'NONE',  ( 1.000000000000000000, 0.000000000000000000, 0.000000000000000000 ) ) ;
#15885=ADVANCED_FACE ( 'NONE', ( #48646 ), #68919, .F. ) ;
#15896=ORIENTED_EDGE ( 'NONE', *, *, #41010, .T. ) ;
#15898=DIRECTION ( 'NONE',  ( 0.000000000000000000, 0.000000000000000000, -1.000000000000000000 ) ) ;
#15902=LINE ( 'NONE', #78032, #25635 ) ;
#15907=EDGE_CURVE ( 'NONE', #81743, #5154, #2225, .T. ) ;
#15932=LINE ( 'NONE', #69539, #59842 ) ;
#15955=VERTEX_POINT ( 'NONE', #64364 ) ;
#15968=EDGE_LOOP ( 'NONE', ( #4528, #58804, #26338, #7351 ) ) ;
#15983=VECTOR ( 'NONE', #65250, 1000.000000000000000 ) ;
#15991=AXIS2_PLACEMENT_3D ( 'NONE', #81244, #27172, #33927 ) ;
#15993=CARTESIAN_POINT ( 'NONE',  ( 6.416666666666664298, -7.500000000000000000, 29.75000000000000355 ) ) ;
#16003=DIRECTION ( 'NONE',  ( 0.000000000000000000, 0.000000000000000000, -1.000000000000000000 ) ) ;
#16006=ORIENTED_EDGE ( 'NONE', *, *, #52712, .F. ) ;
#16017=CARTESIAN_POINT ( 'NONE',  ( 20.00000000000000000, -4.000000000000000000, 29.75000000000000355 ) ) ;
#16019=CARTESIAN_POINT ( 'NONE',  ( -19.50000000000000000, -3.499999999999999556, 29.75000000000000355 ) ) ;
#16062=FACE_OUTER_BOUND ( 'NONE', #42556, .T. ) ;
#16072=ORIENTED_EDGE ( 'NONE', *, *, #26942, .F. ) ;
#16073=VECTOR ( 'NONE', #18583, 1000.000000000000000 ) ;
#16075=PLANE ( 'NONE',  #64053 ) ;
#16090=CARTESIAN_POINT ( 'NONE',  ( -5.448717948717948012, -11.50000000000000000, 29.75000000000000355 ) ) ;
#16100=FACE_OUTER_BOUND ( 'NONE', #58359, .T. ) ;
#16115=AXIS2_PLACEMENT_3D ( 'NONE', #64521, #36635, #64089 ) ;
#16126=CARTESIAN_POINT ( 'NONE',  ( 3.262820512820510999, -3.499999999999999556, 29.75000000000000355 ) ) ;
#16146=DIRECTION ( 'NONE',  ( 1.000000000000000000, 0.000000000000000000, 0.000000000000000000 ) ) ;
#16151=VERTEX_POINT ( 'NONE', #67943 ) ;
#16155=EDGE_CURVE ( 'NONE', #78547, #44728, #87341, .T. ) ;
#16156=DIRECTION ( 'NONE',  ( 1.000000000000000000, 0.000000000000000000, 0.000000000000000000 ) ) ;
#16158=ADVANCED_FACE ( 'NONE', ( #73816 ), #80118, .T. ) ;
#16163=ADVANCED_FACE ( 'NONE', ( #12117 ), #61164, .F. ) ;
#16172=ORIENTED_EDGE ( 'NONE', *, *, #8520, .T. ) ;
#16202=CARTESIAN_POINT ( 'NONE',  ( 9.320512820512821150, -7.500000000000000000, 33.75000000000000000 ) ) ;
#16220=EDGE_CURVE ( 'NONE', #30874, #58158, #30378, .T. ) ;
#16246=ADVANCED_FACE ( 'NONE', ( #84892 ), #29066, .T. ) ;
#16250=EDGE_LOOP ( 'NONE', ( #78204, #1775, #48519, #50498 ) ) ;
#16261=ORIENTED_EDGE ( 'NONE', *, *, #38599, .F. ) ;
#16270=ORIENTED_EDGE ( 'NONE', *, *, #26498, .T. ) ;
#16278=CYLINDRICAL_SURFACE ( 'NONE', #2199, 4.000000000000000000 ) ;
#16289=ORIENTED_EDGE ( 'NONE', *, *, #30331, .T. ) ;
#16293=FACE_OUTER_BOUND ( 'NONE', #56155, .T. ) ;
#16294=EDGE_CURVE ( 'NONE', #74652, #24285, #66832, .T. ) ;
#16296=CARTESIAN_POINT ( 'NONE',  ( 20.00000000000000000, -4.000000000000000000, 29.75000000000000355 ) ) ;
#16298=ORIENTED_EDGE ( 'NONE', *, *, #81831, .F. ) ;
#16314=ORIENTED_EDGE ( 'NONE', *, *, #52590, .F. ) ;
#16327=ADVANCED_FACE ( 'NONE', ( #45216 ), #31720, .T. ) ;
#16328=DIRECTION ( 'NONE',  ( 0.000000000000000000, 0.000000000000000000, -1.000000000000000000 ) ) ;
#16331=CIRCLE ( 'NONE', #52264, 4.000000000000000000 ) ;
#16332=EDGE_LOOP ( 'NONE', ( #11175, #80174, #67997, #43532, #57382 ) ) ;
#16337=DIRECTION ( 'NONE',  ( -0.000000000000000000, 0.000000000000000000, 1.000000000000000000 ) ) ;
#16353=EDGE_CURVE ( 'NONE', #38648, #3292, #6027, .T. ) ;
#16362=CARTESIAN_POINT ( 'NONE',  ( 18.75000000000000000, -7.500000000000000000, 29.75000000000000355 ) ) ;
#16367=CYLINDRICAL_SURFACE ( 'NONE', #959, 4.000000000000000000 ) ;
#16390=CARTESIAN_POINT ( 'NONE',  ( -6.416666666666667851, -3.499999999999999556, 29.75000000000000355 ) ) ;
#16391=EDGE_CURVE ( 'NONE', #75823, #68357, #27171, .T. ) ;
#16424=FACE_OUTER_BOUND ( 'NONE', #13202, .T. ) ;
#16425=DIRECTION ( 'NONE',  ( 0.000000000000000000, 0.000000000000000000, -1.000000000000000000 ) ) ;
#16432=PLANE ( 'NONE',  #54429 ) ;
#16435=DIRECTION ( 'NONE',  ( 1.000000000000000000, 0.000000000000000000, 0.000000000000000000 ) ) ;
#16437=EDGE_CURVE ( 'NONE', #40122, #87461, #13657, .T. ) ;
#16465=DIRECTION ( 'NONE',  ( -0.000000000000000000, 1.000000000000000000, -0.000000000000000000 ) ) ;
#16467=CARTESIAN_POINT ( 'NONE',  ( 7.134615384615385025, -3.499999999999999556, 29.75000000000000355 ) ) ;
#16477=LINE ( 'NONE', #70979, #9790 ) ;
#16481=CARTESIAN_POINT ( 'NONE',  ( 1.326923076923075762, -3.499999999999999556, 29.75000000000000355 ) ) ;
#16484=ORIENTED_EDGE ( 'NONE', *, *, #79684, .F. ) ;
#16488=DIRECTION ( 'NONE',  ( -1.000000000000000000, -0.000000000000000000, -0.000000000000000000 ) ) ;
#16509=DIRECTION ( 'NONE',  ( 1.000000000000000000, 0.000000000000000000, 0.000000000000000000 ) ) ;
#16525=ORIENTED_EDGE ( 'NONE', *, *, #38209, .T. ) ;
#16540=DIRECTION ( 'NONE',  ( -1.000000000000000000, -0.000000000000000000, -0.000000000000000000 ) ) ;
#16575=CARTESIAN_POINT ( 'NONE',  ( -15.84615384615384670, -7.500000000000000000, 29.75000000000000355 ) ) ;
#16576=LINE ( 'NONE', #17476, #85982 ) ;
#16601=EDGE_CURVE ( 'NONE', #76696, #42959, #43350, .T. ) ;
#16608=ORIENTED_EDGE ( 'NONE', *, *, #21707, .T. ) ;
#16615=EDGE_CURVE ( 'NONE', #5809, #34461, #29837, .T. ) ;
#16618=CARTESIAN_POINT ( 'NONE',  ( -2.294871794871794712, -3.499999999999999556, 29.75000000000000355 ) ) ;
#16624=VERTEX_POINT ( 'NONE', #46005 ) ;
#16644=ORIENTED_EDGE ( 'NONE', *, *, #45439, .T. ) ;
#16645=PLANE ( 'NONE',  #63576 ) ;
#16647=LINE ( 'NONE', #10345, #9573 ) ;
#16682=VECTOR ( 'NONE', #14945, 1000.000000000000000 ) ;
#16695=VECTOR ( 'NONE', #35399, 1000.000000000000000 ) ;
#16696=ORIENTED_EDGE ( 'NONE', *, *, #82783, .F. ) ;
#16712=EDGE_CURVE ( 'NONE', #13174, #27068, #80247, .T. ) ;
#16732=DIRECTION ( 'NONE',  ( 0.000000000000000000, 0.000000000000000000, 1.000000000000000000 ) ) ;
#16745=DIRECTION ( 'NONE',  ( -1.000000000000000000, -0.000000000000000000, -0.000000000000000000 ) ) ;
#16765=LINE ( 'NONE', #46020, #68484 ) ;
#16766=LINE ( 'NONE', #79368, #20930 ) ;
#16779=EDGE_CURVE ( 'NONE', #33955, #2392, #33393, .T. ) ;
#16782=DIRECTION ( 'NONE',  ( 1.000000000000000000, 0.000000000000000000, 0.000000000000000000 ) ) ;
#16790=DIRECTION ( 'NONE',  ( -1.000000000000000000, -0.000000000000000000, 0.000000000000000000 ) ) ;
#16796=DIRECTION ( 'NONE',  ( 0.000000000000000000, 0.000000000000000000, -1.000000000000000000 ) ) ;
#16812=ORIENTED_EDGE ( 'NONE', *, *, #7105, .T. ) ;
#16814=ORIENTED_EDGE ( 'NONE', *, *, #38096, .T. ) ;
#16845=LINE ( 'NONE', #44291, #63238 ) ;
#16860=ORIENTED_EDGE ( 'NONE', *, *, #37599, .F. ) ;
#16870=CARTESIAN_POINT ( 'NONE',  ( 11.00641025641025550, -7.500000000000000000, 29.75000000000000355 ) ) ;
#16908=ADVANCED_FACE ( 'NONE', ( #15336 ), #70273, .F. ) ;
#16912=ORIENTED_EDGE ( 'NONE', *, *, #87067, .T. ) ;
#16913=PLANE ( 'NONE',  #51458 ) ;
#16916=DIRECTION ( 'NONE',  ( -1.000000000000000000, -0.000000000000000000, -0.000000000000000000 ) ) ;
#16919=AXIS2_PLACEMENT_3D ( 'NONE', #53292, #18642, #81228 ) ;
#16929=VECTOR ( 'NONE', #66090, 1000.000000000000000 ) ;
#16931=FACE_OUTER_BOUND ( 'NONE', #9395, .T. ) ;
#16933=ADVANCED_FACE ( 'NONE', ( #72930 ), #16645, .F. ) ;
#16936=VERTEX_POINT ( 'NONE', #78344 ) ;
#16937=EDGE_CURVE ( 'NONE', #70729, #77416, #24742, .T. ) ;
#16964=DIRECTION ( 'NONE',  ( -1.000000000000000000, -0.000000000000000000, -0.000000000000000000 ) ) ;
#16983=DIRECTION ( 'NONE',  ( -1.000000000000000000, -0.000000000000000000, 0.000000000000000000 ) ) ;
#17008=ORIENTED_EDGE ( 'NONE', *, *, #73824, .F. ) ;
#17035=CARTESIAN_POINT ( 'NONE',  ( -19.50000000000000000, -3.499999999999999556, 29.75000000000000355 ) ) ;
#17069=DIRECTION ( 'NONE',  ( -0.000000000000000000, 1.000000000000000000, -0.000000000000000000 ) ) ;
#17072=ORIENTED_EDGE ( 'NONE', *, *, #15824, .T. ) ;
#17105=ORIENTED_EDGE ( 'NONE', *, *, #88396, .T. ) ;
#17115=AXIS2_PLACEMENT_3D ( 'NONE', #65377, #79345, #46444 ) ;
#17132=LINE ( 'NONE', #44592, #6244 ) ;
#17137=VECTOR ( 'NONE', #18161, 1000.000000000000000 ) ;
#17149=EDGE_LOOP ( 'NONE', ( #59097, #7381, #58226, #21308, #68307 ) ) ;
#17150=EDGE_LOOP ( 'NONE', ( #29483, #79524, #57031, #49280 ) ) ;
#17159=ORIENTED_EDGE ( 'NONE', *, *, #44371, .T. ) ;
#17165=ADVANCED_FACE ( 'NONE', ( #19328 ), #74271, .T. ) ;
#17170=ORIENTED_EDGE ( 'NONE', *, *, #16937, .F. ) ;
#17194=ORIENTED_EDGE ( 'NONE', *, *, #55161, .F. ) ;
#17208=VERTEX_POINT ( 'NONE', #28747 ) ;
#17254=VERTEX_POINT ( 'NONE', #27851 ) ;
#17258=ORIENTED_EDGE ( 'NONE', *, *, #14074, .T. ) ;
#17265=ADVANCED_FACE ( 'NONE', ( #2144 ), #8027, .F. ) ;
#17276=EDGE_CURVE ( 'NONE', #74633, #37657, #53557, .T. ) ;
#17327=CIRCLE ( 'NONE', #4331, 4.000000000000000000 ) ;
#17333=EDGE_CURVE ( 'NONE', #30874, #6322, #51637, .T. ) ;
#17337=ORIENTED_EDGE ( 'NONE', *, *, #19916, .T. ) ;
#17357=ORIENTED_EDGE ( 'NONE', *, *, #43153, .F. ) ;
#17358=ORIENTED_EDGE ( 'NONE', *, *, #71061, .F. ) ;
#17360=DIRECTION ( 'NONE',  ( 0.000000000000000000, 0.000000000000000000, -1.000000000000000000 ) ) ;
#17369=VERTEX_POINT ( 'NONE', #79590 ) ;
#17383=VECTOR ( 'NONE', #42693, 1000.000000000000000 ) ;
#17397=CIRCLE ( 'NONE', #43313, 4.000000000000000000 ) ;
#17400=VERTEX_POINT ( 'NONE', #39943 ) ;
#17401=EDGE_CURVE ( 'NONE', #17400, #57207, #47565, .T. ) ;
#17410=DIRECTION ( 'NONE',  ( 0.000000000000000000, 0.000000000000000000, -1.000000000000000000 ) ) ;
#17423=VECTOR ( 'NONE', #56364, 1000.000000000000000 ) ;
#17427=PLANE ( 'NONE',  #54289 ) ;
#17436=AXIS2_PLACEMENT_3D ( 'NONE', #27640, #13246, #76719 ) ;
#17445=CARTESIAN_POINT ( 'NONE',  ( -20.00000000000000000, -3.499999999999999556, 29.75000000000000355 ) ) ;
#17455=DIRECTION ( 'NONE',  ( -0.000000000000000000, 1.000000000000000000, -0.000000000000000000 ) ) ;
#17456=EDGE_CURVE ( 'NONE', #81637, #64401, #63649, .T. ) ;
#17475=VECTOR ( 'NONE', #86081, 1000.000000000000000 ) ;
#17476=CARTESIAN_POINT ( 'NONE',  ( 0.000000000000000000, -11.00000000000000000, 29.75000000000000355 ) ) ;
#17480=EDGE_CURVE ( 'NONE', #17254, #47272, #88147, .T. ) ;
#17481=LINE ( 'NONE', #10721, #29356 ) ;
#17493=ORIENTED_EDGE ( 'NONE', *, *, #13382, .F. ) ;
#17499=CARTESIAN_POINT ( 'NONE',  ( -18.03205128205128105, -7.500000000000000000, 29.75000000000000355 ) ) ;
#17500=CARTESIAN_POINT ( 'NONE',  ( 8.352564102564102200, -11.00000000000000000, 29.75000000000000355 ) ) ;
#17513=EDGE_CURVE ( 'NONE', #17369, #17400, #59308, .T. ) ;
#17519=VECTOR ( 'NONE', #71026, 1000.000000000000000 ) ;
#17529=ORIENTED_EDGE ( 'NONE', *, *, #5870, .F. ) ;
#17530=ORIENTED_EDGE ( 'NONE', *, *, #13715, .F. ) ;
#17542=DIRECTION ( 'NONE',  ( -0.000000000000000000, 1.000000000000000000, -0.000000000000000000 ) ) ;
#17565=LINE ( 'NONE', #73395, #78935 ) ;
#17570=VECTOR ( 'NONE', #14826, 1000.000000000000000 ) ;
#17572=ORIENTED_EDGE ( 'NONE', *, *, #3945, .F. ) ;
#17573=PLANE ( 'NONE',  #22615 ) ;
#17583=CARTESIAN_POINT ( 'NONE',  ( 19.50000000000000000, -3.499999999999999556, 29.75000000000000355 ) ) ;
#17586=CARTESIAN_POINT ( 'NONE',  ( -15.84615384615384670, -7.500000000000000000, 29.75000000000000355 ) ) ;
#17587=ORIENTED_EDGE ( 'NONE', *, *, #28048, .T. ) ;
#17594=CARTESIAN_POINT ( 'NONE',  ( -19.50000000000000000, -3.499999999999999556, 29.75000000000000355 ) ) ;
#17595=ORIENTED_EDGE ( 'NONE', *, *, #64595, .F. ) ;
#17598=CIRCLE ( 'NONE', #72219, 4.000000000000000000 ) ;
#17607=AXIS2_PLACEMENT_3D ( 'NONE', #8741, #69542, #7850 ) ;
#17610=DIRECTION ( 'NONE',  ( -1.000000000000000000, -0.000000000000000000, -0.000000000000000000 ) ) ;
#17616=EDGE_LOOP ( 'NONE', ( #77075, #3091, #65989, #68506 ) ) ;
#17622=ORIENTED_EDGE ( 'NONE', *, *, #68801, .F. ) ;
#17643=DIRECTION ( 'NONE',  ( 0.000000000000000000, 0.000000000000000000, 1.000000000000000000 ) ) ;
#17647=DIRECTION ( 'NONE',  ( -1.000000000000000000, -0.000000000000000000, -0.000000000000000000 ) ) ;
#17654=AXIS2_PLACEMENT_3D ( 'NONE', #63, #82492, #20771 ) ;
#17656=ORIENTED_EDGE ( 'NONE', *, *, #38096, .F. ) ;
#17665=DIRECTION ( 'NONE',  ( -0.000000000000000000, 0.000000000000000000, 1.000000000000000000 ) ) ;
#17668=ORIENTED_EDGE ( 'NONE', *, *, #84407, .F. ) ;
#17672=CARTESIAN_POINT ( 'NONE',  ( -10.03846153846153832, -7.500000000000000000, 29.75000000000000355 ) ) ;
#17674=EDGE_CURVE ( 'NONE', #21236, #68727, #43034, .T. ) ;
#17680=CARTESIAN_POINT ( 'NONE',  ( 0.000000000000000000, -11.00000000000000000, 29.75000000000000355 ) ) ;
#17685=CARTESIAN_POINT ( 'NONE',  ( 1.576923076923075762, -7.500000000000000000, 33.75000000000000000 ) ) ;
#17691=CARTESIAN_POINT ( 'NONE',  ( 18.03205128205128105, -3.499999999999999556, 29.75000000000000355 ) ) ;
#17694=EDGE_CURVE ( 'NONE', #75640, #1333, #29139, .T. ) ;
#17707=ORIENTED_EDGE ( 'NONE', *, *, #11303, .T. ) ;
#17708=EDGE_CURVE ( 'NONE', #72244, #5990, #58310, .T. ) ;
#17722=FACE_OUTER_BOUND ( 'NONE', #78041, .T. ) ;
#17727=EDGE_LOOP ( 'NONE', ( #78379, #49234, #1473, #21840 ) ) ;
#17730=VERTEX_POINT ( 'NONE', #78145 ) ;
#17779=DIRECTION ( 'NONE',  ( -1.000000000000000000, -0.000000000000000000, -0.000000000000000000 ) ) ;
#17783=EDGE_CURVE ( 'NONE', #80137, #38748, #23385, .T. ) ;
#17791=ORIENTED_EDGE ( 'NONE', *, *, #76801, .T. ) ;
#17795=EDGE_LOOP ( 'NONE', ( #58488, #1284, #15173, #62216, #72136 ) ) ;
#17798=CARTESIAN_POINT ( 'NONE',  ( 17.06410256410256565, -3.499999999999999556, 29.75000000000000355 ) ) ;
#17832=ORIENTED_EDGE ( 'NONE', *, *, #80007, .F. ) ;
#17840=EDGE_CURVE ( 'NONE', #15955, #48246, #14804, .T. ) ;
#17849=VERTEX_POINT ( 'NONE', #20341 ) ;
#17853=DIRECTION ( 'NONE',  ( -1.000000000000000000, 0.000000000000000000, -0.000000000000000000 ) ) ;
#17869=EDGE_CURVE ( 'NONE', #21320, #86419, #19446, .T. ) ;
#17871=DIRECTION ( 'NONE',  ( -1.000000000000000000, -0.000000000000000000, -0.000000000000000000 ) ) ;
#17889=DIRECTION ( 'NONE',  ( 0.000000000000000000, 0.000000000000000000, -1.000000000000000000 ) ) ;
#17897=CARTESIAN_POINT ( 'NONE',  ( 15.12820512820512953, -7.500000000000000000, 29.75000000000000355 ) ) ;
#17914=DIRECTION ( 'NONE',  ( 1.000000000000000000, 0.000000000000000000, 0.000000000000000000 ) ) ;
#17948=ORIENTED_EDGE ( 'NONE', *, *, #62576, .T. ) ;
#17955=AXIS2_PLACEMENT_3D ( 'NONE', #73353, #26058, #53515 ) ;
#17957=VERTEX_POINT ( 'NONE', #83824 ) ;
#17958=EDGE_CURVE ( 'NONE', #57194, #75095, #22983, .T. ) ;
#17963=PLANE ( 'NONE',  #48504 ) ;
#17972=DIRECTION ( 'NONE',  ( -0.000000000000000000, 0.000000000000000000, 1.000000000000000000 ) ) ;
#17975=EDGE_CURVE ( 'NONE', #72564, #61394, #53617, .T. ) ;
#17982=LINE ( 'NONE', #5353, #47614 ) ;
#18045=DIRECTION ( 'NONE',  ( 1.000000000000000000, 0.000000000000000000, 0.000000000000000000 ) ) ;
#18046=DIRECTION ( 'NONE',  ( -1.000000000000000000, -0.000000000000000000, -0.000000000000000000 ) ) ;
#18051=ORIENTED_EDGE ( 'NONE', *, *, #71995, .T. ) ;
#18052=EDGE_LOOP ( 'NONE', ( #64594, #21372, #31903, #18058 ) ) ;
#18058=ORIENTED_EDGE ( 'NONE', *, *, #85750, .T. ) ;
#18073=CARTESIAN_POINT ( 'NONE',  ( 20.00000000000000000, -4.000000000000000000, 29.75000000000000355 ) ) ;
#18077=VERTEX_POINT ( 'NONE', #24760 ) ;
#18094=CARTESIAN_POINT ( 'NONE',  ( -1.576923076923076872, -11.00000000000000000, 29.75000000000000355 ) ) ;
#18097=ORIENTED_EDGE ( 'NONE', *, *, #16937, .T. ) ;
#18098=EDGE_CURVE ( 'NONE', #76696, #25471, #64680, .T. ) ;
#18105=AXIS2_PLACEMENT_3D ( 'NONE', #26051, #55284, #53506 ) ;
#18129=ORIENTED_EDGE ( 'NONE', *, *, #84407, .T. ) ;
#18146=ORIENTED_EDGE ( 'NONE', *, *, #61909, .F. ) ;
#18155=LINE ( 'NONE', #19920, #40076 ) ;
#18161=DIRECTION ( 'NONE',  ( -0.000000000000000000, 1.000000000000000000, -0.000000000000000000 ) ) ;
#18163=VECTOR ( 'NONE', #62233, 1000.000000000000000 ) ;
#18170=VERTEX_POINT ( 'NONE', #29155 ) ;
#18175=DIRECTION ( 'NONE',  ( 1.000000000000000000, 0.000000000000000000, 0.000000000000000000 ) ) ;
#18185=VECTOR ( 'NONE', #52539, 1000.000000000000000 ) ;
#18193=EDGE_CURVE ( 'NONE', #63742, #81234, #15630, .T. ) ;
#18195=ORIENTED_EDGE ( 'NONE', *, *, #62417, .F. ) ;
#18196=VECTOR ( 'NONE', #45793, 1000.000000000000000 ) ;
#18202=CARTESIAN_POINT ( 'NONE',  ( -19.50000000000000000, -11.50000000000000000, 29.75000000000000355 ) ) ;
#18236=ORIENTED_EDGE ( 'NONE', *, *, #17480, .F. ) ;
#18250=VERTEX_POINT ( 'NONE', #64234 ) ;
#18268=FACE_OUTER_BOUND ( 'NONE', #82250, .T. ) ;
#18270=EDGE_CURVE ( 'NONE', #6115, #7880, #8876, .T. ) ;
#18276=EDGE_CURVE ( 'NONE', #12463, #1012, #43533, .T. ) ;
#18285=ORIENTED_EDGE ( 'NONE', *, *, #71275, .F. ) ;
#18287=LINE ( 'NONE', #52942, #45877 ) ;
#18297=ORIENTED_EDGE ( 'NONE', *, *, #48877, .T. ) ;
#18302=DIRECTION ( 'NONE',  ( 1.000000000000000000, 0.000000000000000000, 0.000000000000000000 ) ) ;
#18306=DIRECTION ( 'NONE',  ( 0.000000000000000000, 0.000000000000000000, -1.000000000000000000 ) ) ;
#18312=VERTEX_POINT ( 'NONE', #44855 ) ;
#18313=DIRECTION ( 'NONE',  ( 0.000000000000000000, 0.000000000000000000, 1.000000000000000000 ) ) ;
#18314=CARTESIAN_POINT ( 'NONE',  ( -13.19230769230769162, -3.499999999999999556, 29.75000000000000355 ) ) ;
#18315=FACE_OUTER_BOUND ( 'NONE', #48149, .T. ) ;
#18327=DIRECTION ( 'NONE',  ( 1.000000000000000000, 0.000000000000000000, 0.000000000000000000 ) ) ;
#18346=DIRECTION ( 'NONE',  ( 1.000000000000000000, 0.000000000000000000, 0.000000000000000000 ) ) ;
#18358=LINE ( 'NONE', #72398, #7122 ) ;
#18361=CARTESIAN_POINT ( 'NONE',  ( -6.166666666666667851, -7.500000000000000000, 29.75000000000000355 ) ) ;
#18370=VERTEX_POINT ( 'NONE', #38563 ) ;
#18394=ORIENTED_EDGE ( 'NONE', *, *, #79201, .F. ) ;
#18396=ORIENTED_EDGE ( 'NONE', *, *, #40494, .T. ) ;
#18398=VECTOR ( 'NONE', #42575, 1000.000000000000000 ) ;
#18401=LINE ( 'NONE', #38666, #41704 ) ;
#18412=DIRECTION ( 'NONE',  ( 1.000000000000000000, 0.000000000000000000, 0.000000000000000000 ) ) ;
#18414=EDGE_CURVE ( 'NONE', #34255, #87211, #3188, .T. ) ;
#18421=DIRECTION ( 'NONE',  ( 1.000000000000000000, 0.000000000000000000, 0.000000000000000000 ) ) ;
#18426=DIRECTION ( 'NONE',  ( 0.000000000000000000, 0.000000000000000000, -1.000000000000000000 ) ) ;
#18428=PLANE ( 'NONE',  #20231 ) ;
#18454=CARTESIAN_POINT ( 'NONE',  ( -19.50000000000000000, -3.499999999999999556, 29.75000000000000355 ) ) ;
#18470=ORIENTED_EDGE ( 'NONE', *, *, #56793, .T. ) ;
#18485=VECTOR ( 'NONE', #8230, 1000.000000000000000 ) ;
#18486=ORIENTED_EDGE ( 'NONE', *, *, #76117, .F. ) ;
#18501=VECTOR ( 'NONE', #29313, 1000.000000000000000 ) ;
#18510=DIRECTION ( 'NONE',  ( -0.000000000000000000, 1.000000000000000000, -0.000000000000000000 ) ) ;
#18521=LINE ( 'NONE', #18963, #39449 ) ;
#18536=CARTESIAN_POINT ( 'NONE',  ( 0.6089743589743582541, -3.499999999999999556, 29.75000000000000355 ) ) ;
#18560=DIRECTION ( 'NONE',  ( 0.000000000000000000, 0.000000000000000000, 1.000000000000000000 ) ) ;
#18570=AXIS2_PLACEMENT_3D ( 'NONE', #52819, #65886, #10958 ) ;
#18578=EDGE_CURVE ( 'NONE', #26148, #48943, #14723, .T. ) ;
#18583=DIRECTION ( 'NONE',  ( -1.000000000000000000, -0.000000000000000000, 0.000000000000000000 ) ) ;
#18587=ORIENTED_EDGE ( 'NONE', *, *, #78682, .T. ) ;
#18607=CIRCLE ( 'NONE', #60250, 4.000000000000000000 ) ;
#18611=DIRECTION ( 'NONE',  ( 1.000000000000000000, 0.000000000000000000, 0.000000000000000000 ) ) ;
#18619=ORIENTED_EDGE ( 'NONE', *, *, #38778, .F. ) ;
#18624=CARTESIAN_POINT ( 'NONE',  ( -13.19230769230769162, -7.500000000000000000, 29.75000000000000355 ) ) ;
#18630=DIRECTION ( 'NONE',  ( 1.000000000000000000, 0.000000000000000000, 0.000000000000000000 ) ) ;
#18633=CIRCLE ( 'NONE', #30125, 4.000000000000000000 ) ;
#18642=DIRECTION ( 'NONE',  ( 1.000000000000000000, 0.000000000000000000, 0.000000000000000000 ) ) ;
#18646=ORIENTED_EDGE ( 'NONE', *, *, #84038, .T. ) ;
#18654=LINE ( 'NONE', #18202, #43428 ) ;
#18657=CARTESIAN_POINT ( 'NONE',  ( -20.00000000000000000, -3.499999999999999556, 28.25000000000000000 ) ) ;
#18670=DIRECTION ( 'NONE',  ( -0.000000000000000000, 1.000000000000000000, -0.000000000000000000 ) ) ;
#18677=CARTESIAN_POINT ( 'NONE',  ( -14.87820512820512953, -3.499999999999999556, 29.75000000000000355 ) ) ;
#18699=EDGE_CURVE ( 'NONE', #61882, #70729, #3853, .T. ) ;
#18719=VERTEX_POINT ( 'NONE', #53378 ) ;
#18730=CARTESIAN_POINT ( 'NONE',  ( -14.87820512820512953, -3.499999999999999556, 29.75000000000000355 ) ) ;
#18743=EDGE_LOOP ( 'NONE', ( #70898, #19812, #72185, #70920 ) ) ;
#18756=FACE_OUTER_BOUND ( 'NONE', #75785, .T. ) ;
#18758=VECTOR ( 'NONE', #46694, 1000.000000000000000 ) ;
#18764=DIRECTION ( 'NONE',  ( 0.000000000000000000, 0.000000000000000000, -1.000000000000000000 ) ) ;
#18780=CARTESIAN_POINT ( 'NONE',  ( 12.94230769230769340, -7.500000000000000000, 29.75000000000000355 ) ) ;
#18811=DIRECTION ( 'NONE',  ( 0.000000000000000000, 0.000000000000000000, -1.000000000000000000 ) ) ;
#18816=ORIENTED_EDGE ( 'NONE', *, *, #1679, .F. ) ;
#18819=VECTOR ( 'NONE', #48775, 1000.000000000000000 ) ;
#18824=AXIS2_PLACEMENT_3D ( 'NONE', #24950, #58733, #51968 ) ;
#18843=VECTOR ( 'NONE', #18045, 1000.000000000000000 ) ;
#18844=DIRECTION ( 'NONE',  ( 0.000000000000000000, 0.000000000000000000, 1.000000000000000000 ) ) ;
#18846=AXIS2_PLACEMENT_3D ( 'NONE', #69039, #75358, #88890 ) ;
#18847=CARTESIAN_POINT ( 'NONE',  ( 8.352564102564102200, -7.500000000000000000, 33.75000000000000000 ) ) ;
#18850=DIRECTION ( 'NONE',  ( -1.000000000000000000, -0.000000000000000000, -0.000000000000000000 ) ) ;
#18851=DIRECTION ( 'NONE',  ( -0.000000000000000000, 1.000000000000000000, -0.000000000000000000 ) ) ;
#18874=DIRECTION ( 'NONE',  ( 0.000000000000000000, 0.000000000000000000, 1.000000000000000000 ) ) ;
#18877=VECTOR ( 'NONE', #32468, 1000.000000000000000 ) ;
#18883=LINE ( 'NONE', #60305, #54611 ) ;
#18897=DIRECTION ( 'NONE',  ( -1.000000000000000000, -0.000000000000000000, -0.000000000000000000 ) ) ;
#18909=ORIENTED_EDGE ( 'NONE', *, *, #19215, .F. ) ;
#18918=EDGE_CURVE ( 'NONE', #87461, #6628, #16331, .T. ) ;
#18944=VERTEX_POINT ( 'NONE', #42099 ) ;
#18946=VECTOR ( 'NONE', #17455, 1000.000000000000000 ) ;
#18959=CARTESIAN_POINT ( 'NONE',  ( -10.03846153846153832, -11.00000000000000000, 29.75000000000000355 ) ) ;
#18963=CARTESIAN_POINT ( 'NONE',  ( -17.06410256410256565, -3.499999999999999556, 29.75000000000000355 ) ) ;
#18965=ORIENTED_EDGE ( 'NONE', *, *, #80007, .T. ) ;
#18966=DIRECTION ( 'NONE',  ( -1.000000000000000000, -0.000000000000000000, -0.000000000000000000 ) ) ;
#18981=VECTOR ( 'NONE', #16465, 1000.000000000000000 ) ;
#19008=FACE_OUTER_BOUND ( 'NONE', #86047, .T. ) ;
#19012=ORIENTED_EDGE ( 'NONE', *, *, #103, .F. ) ;
#19018=DIRECTION ( 'NONE',  ( -0.000000000000000000, 1.000000000000000000, -0.000000000000000000 ) ) ;
#19019=CARTESIAN_POINT ( 'NONE',  ( -0.3589743589743593088, -7.500000000000000000, 29.75000000000000355 ) ) ;
#19029=ADVANCED_FACE ( 'NONE', ( #3303 ), #23138, .F. ) ;
#19052=DIRECTION ( 'NONE',  ( 1.000000000000000000, 0.000000000000000000, 0.000000000000000000 ) ) ;
#19057=ORIENTED_EDGE ( 'NONE', *, *, #7584, .F. ) ;
#19058=EDGE_CURVE ( 'NONE', #72244, #28699, #3750, .T. ) ;
#19063=DIRECTION ( 'NONE',  ( 1.000000000000000000, 0.000000000000000000, 0.000000000000000000 ) ) ;
#19068=CARTESIAN_POINT ( 'NONE',  ( -19.50000000000000000, -3.499999999999999556, 29.75000000000000355 ) ) ;
#19071=AXIS2_PLACEMENT_3D ( 'NONE', #38179, #9821, #72404 ) ;
#19072=ORIENTED_EDGE ( 'NONE', *, *, #32911, .F. ) ;
#19092=DIRECTION ( 'NONE',  ( -0.000000000000000000, 1.000000000000000000, -0.000000000000000000 ) ) ;
#19094=ORIENTED_EDGE ( 'NONE', *, *, #44420, .F. ) ;
#19114=LINE ( 'NONE', #66407, #12298 ) ;
#19117=ORIENTED_EDGE ( 'NONE', *, *, #70213, .T. ) ;
#19135=VECTOR ( 'NONE', #40802, 1000.000000000000000 ) ;
#19137=AXIS2_PLACEMENT_3D ( 'NONE', #48848, #76321, #14628 ) ;
#19139=VERTEX_POINT ( 'NONE', #66791 ) ;
#19141=FACE_OUTER_BOUND ( 'NONE', #78182, .T. ) ;
#19146=AXIS2_PLACEMENT_3D ( 'NONE', #62556, #62993, #48162 ) ;
#19160=EDGE_CURVE ( 'NONE', #26482, #48447, #46076, .T. ) ;
#19182=AXIS2_PLACEMENT_3D ( 'NONE', #68668, #6969, #47057 ) ;
#19197=EDGE_CURVE ( 'NONE', #34055, #78547, #62677, .T. ) ;
#19200=LINE ( 'NONE', #11561, #44388 ) ;
#19215=EDGE_CURVE ( 'NONE', #81105, #57687, #78177, .T. ) ;
#19216=ORIENTED_EDGE ( 'NONE', *, *, #41094, .T. ) ;
#19218=ORIENTED_EDGE ( 'NONE', *, *, #74713, .F. ) ;
#19220=EDGE_LOOP ( 'NONE', ( #51755, #45089, #67399, #54125, #87305 ) ) ;
#19222=DIRECTION ( 'NONE',  ( 0.000000000000000000, 0.000000000000000000, -1.000000000000000000 ) ) ;
#19239=ORIENTED_EDGE ( 'NONE', *, *, #23278, .T. ) ;
#19246=CARTESIAN_POINT ( 'NONE',  ( -3.262820512820514107, -3.499999999999999556, 29.75000000000000355 ) ) ;
#19247=CARTESIAN_POINT ( 'NONE',  ( -19.50000000000000000, -3.499999999999999556, 29.75000000000000355 ) ) ;
#19254=VERTEX_POINT ( 'NONE', #13180 ) ;
#19256=DIRECTION ( 'NONE',  ( -0.000000000000000000, 1.000000000000000000, -0.000000000000000000 ) ) ;
#19257=VECTOR ( 'NONE', #70309, 1000.000000000000000 ) ;
#19271=ORIENTED_EDGE ( 'NONE', *, *, #17975, .T. ) ;
#19279=LINE ( 'NONE', #6645, #13660 ) ;
#19288=LINE ( 'NONE', #26047, #12277 ) ;
#19293=DIRECTION ( 'NONE',  ( 0.000000000000000000, 0.000000000000000000, -1.000000000000000000 ) ) ;
#19313=ADVANCED_FACE ( 'NONE', ( #36119 ), #16278, .T. ) ;
#19318=CARTESIAN_POINT ( 'NONE',  ( -11.00641025641025550, -7.500000000000000000, 29.75000000000000355 ) ) ;
#19325=CIRCLE ( 'NONE', #66825, 4.000000000000000000 ) ;
#19328=FACE_OUTER_BOUND ( 'NONE', #54263, .T. ) ;
#19341=CARTESIAN_POINT ( 'NONE',  ( -19.50000000000000000, -3.499999999999999556, 29.75000000000000355 ) ) ;
#19357=VECTOR ( 'NONE', #53659, 1000.000000000000000 ) ;
#19363=ORIENTED_EDGE ( 'NONE', *, *, #64924, .T. ) ;
#19394=ADVANCED_FACE ( 'NONE', ( #50055 ), #9089, .F. ) ;
#19400=FACE_OUTER_BOUND ( 'NONE', #17795, .T. ) ;
#19401=LINE ( 'NONE', #68469, #89171 ) ;
#19402=DIRECTION ( 'NONE',  ( 0.000000000000000000, 0.000000000000000000, 1.000000000000000000 ) ) ;
#19413=LINE ( 'NONE', #67608, #8785 ) ;
#19414=ORIENTED_EDGE ( 'NONE', *, *, #24899, .T. ) ;
#19425=ORIENTED_EDGE ( 'NONE', *, *, #40988, .T. ) ;
#19429=VERTEX_POINT ( 'NONE', #38772 ) ;
#19430=CYLINDRICAL_SURFACE ( 'NONE', #43861, 4.000000000000000000 ) ;
#19439=DIRECTION ( 'NONE',  ( -1.000000000000000000, -0.000000000000000000, -0.000000000000000000 ) ) ;
#19446=LINE ( 'NONE', #6812, #59402 ) ;
#19454=LINE ( 'NONE', #19894, #33992 ) ;
#19467=FACE_OUTER_BOUND ( 'NONE', #33929, .T. ) ;
#19480=DIRECTION ( 'NONE',  ( -1.000000000000000000, -0.000000000000000000, -0.000000000000000000 ) ) ;
#19487=CARTESIAN_POINT ( 'NONE',  ( 17.06410256410256565, -3.499999999999999556, 29.75000000000000355 ) ) ;
#19488=EDGE_CURVE ( 'NONE', #1493, #80799, #12190, .T. ) ;
#19505=EDGE_CURVE ( 'NONE', #20712, #5961, #51353, .T. ) ;
#19516=ORIENTED_EDGE ( 'NONE', *, *, #16601, .T. ) ;
#19528=DIRECTION ( 'NONE',  ( -1.000000000000000000, -0.000000000000000000, -0.000000000000000000 ) ) ;
#19542=LINE ( 'NONE', #20434, #9519 ) ;
#19556=VERTEX_POINT ( 'NONE', #26587 ) ;
#19566=DIRECTION ( 'NONE',  ( 0.000000000000000000, 0.000000000000000000, -1.000000000000000000 ) ) ;
#19573=FACE_OUTER_BOUND ( 'NONE', #84994, .T. ) ;
#19582=VECTOR ( 'NONE', #27823, 1000.000000000000000 ) ;
#19601=VERTEX_POINT ( 'NONE', #29255 ) ;
#19604=LINE ( 'NONE', #20490, #73153 ) ;
#19607=CARTESIAN_POINT ( 'NONE',  ( 7.384615384615385025, -3.499999999999999556, 29.75000000000000355 ) ) ;
#19614=ORIENTED_EDGE ( 'NONE', *, *, #2716, .T. ) ;
#19629=ORIENTED_EDGE ( 'NONE', *, *, #33937, .T. ) ;
#19720=CARTESIAN_POINT ( 'NONE',  ( -15.12820512820512953, -7.500000000000000000, 29.75000000000000355 ) ) ;
#19746=FILL_AREA_STYLE ('',( #13868 ) ) ;
#19758=DIRECTION ( 'NONE',  ( 0.000000000000000000, 0.000000000000000000, -1.000000000000000000 ) ) ;
#19759=DIRECTION ( 'NONE',  ( 1.000000000000000000, 0.000000000000000000, 0.000000000000000000 ) ) ;
#19785=ORIENTED_EDGE ( 'NONE', *, *, #86511, .T. ) ;
#19791=AXIS2_PLACEMENT_3D ( 'NONE', #59492, #32463, #60378 ) ;
#19795=ORIENTED_EDGE ( 'NONE', *, *, #22921, .T. ) ;
#19812=ORIENTED_EDGE ( 'NONE', *, *, #73551, .F. ) ;
#19821=VECTOR ( 'NONE', #27620, 1000.000000000000000 ) ;
#19843=CYLINDRICAL_SURFACE ( 'NONE', #58204, 4.000000000000000000 ) ;
#19845=VECTOR ( 'NONE', #63387, 1000.000000000000000 ) ;
#19855=DIRECTION ( 'NONE',  ( -1.000000000000000000, -0.000000000000000000, -0.000000000000000000 ) ) ;
#19860=AXIS2_PLACEMENT_3D ( 'NONE', #68983, #6412, #13601 ) ;
#19862=DIRECTION ( 'NONE',  ( -0.000000000000000000, 0.000000000000000000, 1.000000000000000000 ) ) ;
#19868=CARTESIAN_POINT ( 'NONE',  ( 7.384615384615385025, -11.50000000000000000, 29.75000000000000355 ) ) ;
#19893=DIRECTION ( 'NONE',  ( 0.000000000000000000, 0.000000000000000000, -1.000000000000000000 ) ) ;
#19894=CARTESIAN_POINT ( 'NONE',  ( -19.50000000000000000, -3.499999999999999556, 29.75000000000000355 ) ) ;
#19911=DIRECTION ( 'NONE',  ( 1.000000000000000000, 0.000000000000000000, 0.000000000000000000 ) ) ;
#19913=VECTOR ( 'NONE', #82695, 1000.000000000000000 ) ;
#19916=EDGE_CURVE ( 'NONE', #9623, #34447, #19279, .T. ) ;
#19918=VECTOR ( 'NONE', #5468, 1000.000000000000000 ) ;
#19920=CARTESIAN_POINT ( 'NONE',  ( 8.352564102564102200, -11.50000000000000000, 29.75000000000000355 ) ) ;
#19926=EDGE_CURVE ( 'NONE', #43749, #20735, #12520, .T. ) ;
#19931=VERTEX_POINT ( 'NONE', #40007 ) ;
#19979=CIRCLE ( 'NONE', #1331, 4.000000000000000000 ) ;
#19988=DIRECTION ( 'NONE',  ( -0.000000000000000000, 0.000000000000000000, 1.000000000000000000 ) ) ;
#19993=ORIENTED_EDGE ( 'NONE', *, *, #6565, .T. ) ;
#19996=VERTEX_POINT ( 'NONE', #81432 ) ;
#20000=EDGE_LOOP ( 'NONE', ( #20399, #7709, #28855, #21385 ) ) ;
#20003=CARTESIAN_POINT ( 'NONE',  ( 2.294871794871793380, -3.499999999999999556, 29.75000000000000355 ) ) ;
#20035=VECTOR ( 'NONE', #86868, 1000.000000000000000 ) ;
#20036=DIRECTION ( 'NONE',  ( -1.000000000000000000, 0.000000000000000000, -0.000000000000000000 ) ) ;
#20037=EDGE_CURVE ( 'NONE', #77909, #63742, #31234, .T. ) ;
#20055=DIRECTION ( 'NONE',  ( -0.000000000000000000, 1.000000000000000000, -0.000000000000000000 ) ) ;
#20062=DIRECTION ( 'NONE',  ( 0.000000000000000000, 0.000000000000000000, -1.000000000000000000 ) ) ;
#20072=EDGE_CURVE ( 'NONE', #38958, #85779, #76880, .T. ) ;
#20111=EDGE_CURVE ( 'NONE', #42018, #59060, #88525, .T. ) ;
#20124=ORIENTED_EDGE ( 'NONE', *, *, #78640, .F. ) ;
#20129=ORIENTED_EDGE ( 'NONE', *, *, #5682, .T. ) ;
#20138=CARTESIAN_POINT ( 'NONE',  ( -10.28846153846153832, -4.000000000000000000, 29.75000000000000355 ) ) ;
#20161=ADVANCED_FACE ( 'NONE', ( #14967 ), #75765, .T. ) ;
#20174=CARTESIAN_POINT ( 'NONE',  ( -14.87820512820512953, -11.50000000000000000, 29.75000000000000355 ) ) ;
#20189=DIRECTION ( 'NONE',  ( 0.000000000000000000, -1.000000000000000000, 0.000000000000000000 ) ) ;
#20190=DIRECTION ( 'NONE',  ( -0.000000000000000000, 1.000000000000000000, -0.000000000000000000 ) ) ;
#20196=ORIENTED_EDGE ( 'NONE', *, *, #86616, .T. ) ;
#20207=PLANE ( 'NONE',  #22960 ) ;
#20217=DIRECTION ( 'NONE',  ( 0.000000000000000000, 0.000000000000000000, -1.000000000000000000 ) ) ;
#20225=FACE_OUTER_BOUND ( 'NONE', #36055, .T. ) ;
#20231=AXIS2_PLACEMENT_3D ( 'NONE', #23076, #31492, #44991 ) ;
#20233=ORIENTED_EDGE ( 'NONE', *, *, #17975, .F. ) ;
#20234=DIRECTION ( 'NONE',  ( -0.000000000000000000, 1.000000000000000000, -0.000000000000000000 ) ) ;
#20254=ORIENTED_EDGE ( 'NONE', *, *, #33188, .F. ) ;
#20273=EDGE_CURVE ( 'NONE', #74021, #50542, #57272, .T. ) ;
#20287=VECTOR ( 'NONE', #54186, 1000.000000000000000 ) ;
#20296=CARTESIAN_POINT ( 'NONE',  ( 20.00000000000000000, -4.000000000000000000, 29.75000000000000355 ) ) ;
#20309=DIRECTION ( 'NONE',  ( 1.000000000000000000, 0.000000000000000000, 0.000000000000000000 ) ) ;
#20329=CARTESIAN_POINT ( 'NONE',  ( 6.416666666666664298, -7.500000000000000000, 33.75000000000000000 ) ) ;
#20331=PLANE ( 'NONE',  #36853 ) ;
#20336=ADVANCED_FACE ( 'NONE', ( #30682 ), #9967, .T. ) ;
#20341=CARTESIAN_POINT ( 'NONE',  ( 5.448717948717947124, -11.00000000000000000, 29.75000000000000355 ) ) ;
#20350=CARTESIAN_POINT ( 'NONE',  ( 11.97435897435897267, -7.500000000000000000, 29.75000000000000355 ) ) ;
#20356=CARTESIAN_POINT ( 'NONE',  ( 10.28846153846153832, -4.000000000000000000, 29.75000000000000355 ) ) ;
#20358=VERTEX_POINT ( 'NONE', #45079 ) ;
#20359=PRODUCT_DEFINITION_SHAPE ( 'NONE', 'NONE',  #35967 ) ;
#20386=AXIS2_PLACEMENT_3D ( 'NONE', #68252, #34015, #56062 ) ;
#20393=DIRECTION ( 'NONE',  ( 1.000000000000000000, 0.000000000000000000, 0.000000000000000000 ) ) ;
#20399=ORIENTED_EDGE ( 'NONE', *, *, #50439, .F. ) ;
#20401=ORIENTED_EDGE ( 'NONE', *, *, #26310, .T. ) ;
#20434=CARTESIAN_POINT ( 'NONE',  ( -10.03846153846153832, -7.500000000000000000, 33.75000000000000000 ) ) ;
#20441=CARTESIAN_POINT ( 'NONE',  ( 12.22435897435897267, -7.500000000000000000, 29.75000000000000355 ) ) ;
#20442=DIRECTION ( 'NONE',  ( 0.000000000000000000, 0.000000000000000000, 1.000000000000000000 ) ) ;
#20460=DIRECTION ( 'NONE',  ( 1.000000000000000000, 0.000000000000000000, 0.000000000000000000 ) ) ;
#20461=VECTOR ( 'NONE', #57747, 1000.000000000000000 ) ;
#20476=VERTEX_POINT ( 'NONE', #13523 ) ;
#20486=ORIENTED_EDGE ( 'NONE', *, *, #6565, .F. ) ;
#20490=CARTESIAN_POINT ( 'NONE',  ( 6.416666666666664298, -3.499999999999999556, 29.75000000000000355 ) ) ;
#20492=PLANE ( 'NONE',  #75384 ) ;
#20497=ORIENTED_EDGE ( 'NONE', *, *, #39765, .F. ) ;
#20517=LINE ( 'NONE', #88561, #79190 ) ;
#20526=CARTESIAN_POINT ( 'NONE',  ( -0.6089743589743593644, -11.00000000000000000, 29.75000000000000355 ) ) ;
#20527=EDGE_CURVE ( 'NONE', #45384, #30104, #2269, .T. ) ;
#20566=CARTESIAN_POINT ( 'NONE',  ( -12.94230769230769162, -11.00000000000000000, 29.75000000000000355 ) ) ;
#20577=ORIENTED_EDGE ( 'NONE', *, *, #59173, .T. ) ;
#20585=EDGE_CURVE ( 'NONE', #57207, #36536, #42779, .T. ) ;
#20617=CARTESIAN_POINT ( 'NONE',  ( 19.00000000000000000, -3.499999999999999556, 29.75000000000000355 ) ) ;
#20625=DIRECTION ( 'NONE',  ( 1.000000000000000000, 0.000000000000000000, 0.000000000000000000 ) ) ;
#20627=VECTOR ( 'NONE', #41962, 1000.000000000000000 ) ;
#20630=DIRECTION ( 'NONE',  ( -1.000000000000000000, -0.000000000000000000, -0.000000000000000000 ) ) ;
#20631=ORIENTED_EDGE ( 'NONE', *, *, #87488, .T. ) ;
#20658=FACE_OUTER_BOUND ( 'NONE', #75718, .T. ) ;
#20670=AXIS2_PLACEMENT_3D ( 'NONE', #30540, #63880, #22019 ) ;
#20677=ORIENTED_EDGE ( 'NONE', *, *, #77500, .T. ) ;
#20683=DIRECTION ( 'NONE',  ( -1.000000000000000000, 0.000000000000000000, -0.000000000000000000 ) ) ;
#20712=VERTEX_POINT ( 'NONE', #59825 ) ;
#20714=CARTESIAN_POINT ( 'NONE',  ( -19.50000000000000000, -4.000000000000000000, 29.75000000000000355 ) ) ;
#20730=DIRECTION ( 'NONE',  ( -1.000000000000000000, -0.000000000000000000, 0.000000000000000000 ) ) ;
#20735=VERTEX_POINT ( 'NONE', #86438 ) ;
#20766=DIRECTION ( 'NONE',  ( 1.000000000000000000, 0.000000000000000000, 0.000000000000000000 ) ) ;
#20771=DIRECTION ( 'NONE',  ( 0.000000000000000000, 0.000000000000000000, -1.000000000000000000 ) ) ;
#20777=CARTESIAN_POINT ( 'NONE',  ( -0.3589743589743586982, -11.50000000000000000, 29.75000000000000355 ) ) ;
#20794=ADVANCED_FACE ( 'NONE', ( #82330 ), #48078, .T. ) ;
#20798=LINE ( 'NONE', #1415, #80238 ) ;
#20799=FACE_OUTER_BOUND ( 'NONE', #72355, .T. ) ;
#20804=EDGE_CURVE ( 'NONE', #85054, #77909, #22400, .T. ) ;
#20809=EDGE_CURVE ( 'NONE', #6970, #80662, #53958, .T. ) ;
#20826=DIRECTION ( 'NONE',  ( 0.000000000000000000, 0.000000000000000000, -1.000000000000000000 ) ) ;
#20827=EDGE_CURVE ( 'NONE', #48447, #78324, #77065, .T. ) ;
#20828=DIRECTION ( 'NONE',  ( -0.000000000000000000, 1.000000000000000000, -0.000000000000000000 ) ) ;
#20865=LINE ( 'NONE', #26298, #31204 ) ;
#20873=DIRECTION ( 'NONE',  ( -1.000000000000000000, -0.000000000000000000, -0.000000000000000000 ) ) ;
#20878=PLANE ( 'NONE',  #17436 ) ;
#20882=VERTEX_POINT ( 'NONE', #62912 ) ;
#20886=DIRECTION ( 'NONE',  ( 1.000000000000000000, 0.000000000000000000, 0.000000000000000000 ) ) ;
#20888=AXIS2_PLACEMENT_3D ( 'NONE', #45409, #67479, #53053 ) ;
#20892=EDGE_CURVE ( 'NONE', #37401, #17730, #23266, .T. ) ;
#20914=EDGE_LOOP ( 'NONE', ( #18396, #53695, #10707, #8858, #77225 ) ) ;
#20916=DIRECTION ( 'NONE',  ( 1.000000000000000000, 0.000000000000000000, 0.000000000000000000 ) ) ;
#20920=DIRECTION ( 'NONE',  ( -1.000000000000000000, 0.000000000000000000, -0.000000000000000000 ) ) ;
#20924=VERTEX_POINT ( 'NONE', #69686 ) ;
#20930=VECTOR ( 'NONE', #58637, 1000.000000000000000 ) ;
#20950=DIRECTION ( 'NONE',  ( -0.000000000000000000, 0.000000000000000000, 1.000000000000000000 ) ) ;
#20967=LINE ( 'NONE', #42153, #53393 ) ;
#20969=ORIENTED_EDGE ( 'NONE', *, *, #21788, .T. ) ;
#20978=VECTOR ( 'NONE', #24895, 1000.000000000000000 ) ;
#20985=FACE_OUTER_BOUND ( 'NONE', #77381, .T. ) ;
#20988=CARTESIAN_POINT ( 'NONE',  ( -3.262820512820514107, -3.499999999999999556, 29.75000000000000355 ) ) ;
#20993=FACE_OUTER_BOUND ( 'NONE', #13318, .T. ) ;
#20996=DIRECTION ( 'NONE',  ( 1.000000000000000000, 0.000000000000000000, 0.000000000000000000 ) ) ;
#21000=CARTESIAN_POINT ( 'NONE',  ( -13.91025641025641058, -7.500000000000000000, 29.75000000000000355 ) ) ;
#21005=EDGE_CURVE ( 'NONE', #83848, #50855, #76454, .T. ) ;
#21021=ORIENTED_EDGE ( 'NONE', *, *, #14828, .F. ) ;
#21027=ADVANCED_FACE ( 'NONE', ( #29162 ), #16075, .F. ) ;
#21034=FACE_OUTER_BOUND ( 'NONE', #79897, .T. ) ;
#21038=VERTEX_POINT ( 'NONE', #31818 ) ;
#21061=ORIENTED_EDGE ( 'NONE', *, *, #79422, .T. ) ;
#21076=CARTESIAN_POINT ( 'NONE',  ( -14.16025641025641058, -7.500000000000000000, 29.75000000000000355 ) ) ;
#21082=LINE ( 'NONE', #89135, #61375 ) ;
#21093=CARTESIAN_POINT ( 'NONE',  ( -15.84615384615384670, -3.499999999999999556, 29.75000000000000355 ) ) ;
#21095=AXIS2_PLACEMENT_3D ( 'NONE', #78150, #15130, #23645 ) ;
#21112=VECTOR ( 'NONE', #12937, 1000.000000000000000 ) ;
#21122=CARTESIAN_POINT ( 'NONE',  ( -6.416666666666667851, -7.500000000000000000, 29.75000000000000355 ) ) ;
#21123=CARTESIAN_POINT ( 'NONE',  ( 19.00000000000000000, -4.000000000000000000, 29.75000000000000355 ) ) ;
#21136=PLANE ( 'NONE',  #46638 ) ;
#21141=VECTOR ( 'NONE', #20234, 1000.000000000000000 ) ;
#21144=ORIENTED_EDGE ( 'NONE', *, *, #84869, .F. ) ;
#21146=ORIENTED_EDGE ( 'NONE', *, *, #78074, .F. ) ;
#21155=DIRECTION ( 'NONE',  ( -0.000000000000000000, 1.000000000000000000, -0.000000000000000000 ) ) ;
#21162=AXIS2_PLACEMENT_3D ( 'NONE', #83079, #20916, #6531 ) ;
#21164=CARTESIAN_POINT ( 'NONE',  ( -14.87820512820512953, -3.499999999999999556, 29.75000000000000355 ) ) ;
#21171=VECTOR ( 'NONE', #28100, 1000.000000000000000 ) ;
#21181=ORIENTED_EDGE ( 'NONE', *, *, #22122, .T. ) ;
#21182=EDGE_CURVE ( 'NONE', #62448, #83471, #52685, .T. ) ;
#21218=CARTESIAN_POINT ( 'NONE',  ( -14.87820512820512953, -3.499999999999999556, 29.75000000000000355 ) ) ;
#21236=VERTEX_POINT ( 'NONE', #39910 ) ;
#21269=DIRECTION ( 'NONE',  ( 1.000000000000000000, 0.000000000000000000, 0.000000000000000000 ) ) ;
#21270=ORIENTED_EDGE ( 'NONE', *, *, #5870, .T. ) ;
#21280=DIRECTION ( 'NONE',  ( -1.000000000000000000, -0.000000000000000000, -0.000000000000000000 ) ) ;
#21284=CARTESIAN_POINT ( 'NONE',  ( 19.00000000000000000, -7.500000000000000000, 29.75000000000000355 ) ) ;
#21291=EDGE_CURVE ( 'NONE', #12551, #24740, #45166, .T. ) ;
#21294=LINE ( 'NONE', #69486, #73459 ) ;
#21296=CARTESIAN_POINT ( 'NONE',  ( -10.03846153846153832, -3.499999999999999556, 29.75000000000000355 ) ) ;
#21298=ORIENTED_EDGE ( 'NONE', *, *, #25571, .F. ) ;
#21308=ORIENTED_EDGE ( 'NONE', *, *, #64257, .F. ) ;
#21316=EDGE_CURVE ( 'NONE', #16624, #88786, #38421, .T. ) ;
#21320=VERTEX_POINT ( 'NONE', #4184 ) ;
#21323=ORIENTED_EDGE ( 'NONE', *, *, #88510, .F. ) ;
#21340=ADVANCED_FACE ( 'NONE', ( #53704 ), #28011, .F. ) ;
#21341=EDGE_CURVE ( 'NONE', #8541, #55049, #82961, .T. ) ;
#21348=EDGE_LOOP ( 'NONE', ( #10664, #7379, #17159, #80582 ) ) ;
#21356=DIRECTION ( 'NONE',  ( -0.000000000000000000, 1.000000000000000000, -0.000000000000000000 ) ) ;
#21372=ORIENTED_EDGE ( 'NONE', *, *, #4959, .F. ) ;
#21385=ORIENTED_EDGE ( 'NONE', *, *, #15674, .T. ) ;
#21400=VERTEX_POINT ( 'NONE', #74879 ) ;
#21408=CARTESIAN_POINT ( 'NONE',  ( 17.06410256410256565, -7.500000000000000000, 29.75000000000000355 ) ) ;
#21423=DIRECTION ( 'NONE',  ( -0.000000000000000000, 1.000000000000000000, -0.000000000000000000 ) ) ;
#21431=ORIENTED_EDGE ( 'NONE', *, *, #39883, .F. ) ;
#21434=VERTEX_POINT ( 'NONE', #1865 ) ;
#21443=FACE_OUTER_BOUND ( 'NONE', #75094, .T. ) ;
#21448=CARTESIAN_POINT ( 'NONE',  ( 20.00000000000000000, -4.000000000000000000, 29.75000000000000355 ) ) ;
#21459=VERTEX_POINT ( 'NONE', #56370 ) ;
#21471=CARTESIAN_POINT ( 'NONE',  ( -19.50000000000000000, -3.499999999999999556, 29.75000000000000355 ) ) ;
#21473=PLANE ( 'NONE',  #9295 ) ;
#21478=ORIENTED_EDGE ( 'NONE', *, *, #42861, .F. ) ;
#21500=EDGE_CURVE ( 'NONE', #53616, #19601, #2293, .T. ) ;
#21526=CARTESIAN_POINT ( 'NONE',  ( -19.50000000000000000, -3.499999999999999556, 29.75000000000000355 ) ) ;
#21544=LINE ( 'NONE', #82375, #2174 ) ;
#21548=EDGE_CURVE ( 'NONE', #19601, #51674, #36107, .T. ) ;
#21556=ADVANCED_FACE ( 'NONE', ( #35662 ), #15391, .T. ) ;
#21562=VERTEX_POINT ( 'NONE', #42863 ) ;
#21616=EDGE_CURVE ( 'NONE', #53616, #55785, #62667, .T. ) ;
#21627=DIRECTION ( 'NONE',  ( 0.000000000000000000, 0.000000000000000000, -1.000000000000000000 ) ) ;
#21636=VECTOR ( 'NONE', #2763, 1000.000000000000000 ) ;
#21653=DIRECTION ( 'NONE',  ( 1.000000000000000000, 0.000000000000000000, 0.000000000000000000 ) ) ;
#21667=EDGE_CURVE ( 'NONE', #85035, #2085, #41344, .T. ) ;
#21692=ORIENTED_EDGE ( 'NONE', *, *, #84869, .T. ) ;
#21694=AXIS2_PLACEMENT_3D ( 'NONE', #56951, #10553, #51059 ) ;
#21699=AXIS2_PLACEMENT_3D ( 'NONE', #59601, #18630, #51946 ) ;
#21701=ADVANCED_FACE ( 'NONE', ( #61156 ), #28716, .T. ) ;
#21702=DIRECTION ( 'NONE',  ( -1.000000000000000000, -0.000000000000000000, 0.000000000000000000 ) ) ;
#21705=CIRCLE ( 'NONE', #11694, 4.000000000000000000 ) ;
#21706=ORIENTED_EDGE ( 'NONE', *, *, #64542, .T. ) ;
#21707=EDGE_CURVE ( 'NONE', #58726, #62375, #54404, .T. ) ;
#21715=ORIENTED_EDGE ( 'NONE', *, *, #68415, .F. ) ;
#21719=LINE ( 'NONE', #82983, #69646 ) ;
#21735=ORIENTED_EDGE ( 'NONE', *, *, #7400, .T. ) ;
#21750=LINE ( 'NONE', #30283, #37989 ) ;
#21751=PLANE ( 'NONE',  #69148 ) ;
#21763=DIRECTION ( 'NONE',  ( -1.000000000000000000, -0.000000000000000000, -0.000000000000000000 ) ) ;
#21766=AXIS2_PLACEMENT_3D ( 'NONE', #20441, #36181, #42050 ) ;
#21775=CARTESIAN_POINT ( 'NONE',  ( 4.480769230769229061, -11.00000000000000000, 29.75000000000000355 ) ) ;
#21788=EDGE_CURVE ( 'NONE', #32252, #24890, #71455, .T. ) ;
#21794=DIRECTION ( 'NONE',  ( 0.000000000000000000, 0.000000000000000000, -1.000000000000000000 ) ) ;
#21819=ADVANCED_FACE ( 'NONE', ( #34357 ), #73705, .F. ) ;
#21821=LINE ( 'NONE', #51035, #11417 ) ;
#21837=CARTESIAN_POINT ( 'NONE',  ( -12.94230769230769162, -7.500000000000000000, 29.75000000000000355 ) ) ;
#21840=ORIENTED_EDGE ( 'NONE', *, *, #12768, .T. ) ;
#21850=CARTESIAN_POINT ( 'NONE',  ( 0.6089743589743582541, -7.500000000000000000, 29.75000000000000355 ) ) ;
#21866=VECTOR ( 'NONE', #65425, 1000.000000000000000 ) ;
#21877=EDGE_CURVE ( 'NONE', #54838, #56977, #5185, .T. ) ;
#21900=DIRECTION ( 'NONE',  ( 1.000000000000000000, 0.000000000000000000, 0.000000000000000000 ) ) ;
#21912=ADVANCED_FACE ( 'NONE', ( #75357 ), #80001, .F. ) ;
#21913=ORIENTED_EDGE ( 'NONE', *, *, #50439, .T. ) ;
#21915=DIRECTION ( 'NONE',  ( 0.000000000000000000, 0.000000000000000000, -1.000000000000000000 ) ) ;
#21922=AXIS2_PLACEMENT_3D ( 'NONE', #12570, #40057, #26532 ) ;
#21924=VERTEX_POINT ( 'NONE', #59729 ) ;
#21942=DIRECTION ( 'NONE',  ( 0.000000000000000000, 0.000000000000000000, -1.000000000000000000 ) ) ;
#21947=ORIENTED_EDGE ( 'NONE', *, *, #89019, .T. ) ;
#21958=CARTESIAN_POINT ( 'NONE',  ( 14.16025641025641235, -7.500000000000000000, 29.75000000000000355 ) ) ;
#21972=DIRECTION ( 'NONE',  ( -1.000000000000000000, -0.000000000000000000, -0.000000000000000000 ) ) ;
#21995=VECTOR ( 'NONE', #63804, 1000.000000000000000 ) ;
#22007=ORIENTED_EDGE ( 'NONE', *, *, #70919, .T. ) ;
#22019=DIRECTION ( 'NONE',  ( 0.000000000000000000, 0.000000000000000000, -1.000000000000000000 ) ) ;
#22053=EDGE_CURVE ( 'NONE', #50855, #69909, #76686, .T. ) ;
#22054=DIRECTION ( 'NONE',  ( 1.000000000000000000, 0.000000000000000000, 0.000000000000000000 ) ) ;
#22055=VERTEX_POINT ( 'NONE', #7345 ) ;
#22063=LINE ( 'NONE', #8554, #78306 ) ;
#22065=ORIENTED_EDGE ( 'NONE', *, *, #38287, .F. ) ;
#22083=DIRECTION ( 'NONE',  ( 1.000000000000000000, 0.000000000000000000, 0.000000000000000000 ) ) ;
#22084=ORIENTED_EDGE ( 'NONE', *, *, #2287, .T. ) ;
#22091=CARTESIAN_POINT ( 'NONE',  ( -18.03205128205128105, -7.500000000000000000, 33.75000000000000000 ) ) ;
#22092=DIRECTION ( 'NONE',  ( 0.000000000000000000, 0.000000000000000000, -1.000000000000000000 ) ) ;
#22100=ORIENTED_EDGE ( 'NONE', *, *, #39651, .F. ) ;
#22101=DIRECTION ( 'NONE',  ( 0.000000000000000000, 0.000000000000000000, 1.000000000000000000 ) ) ;
#22107=CARTESIAN_POINT ( 'NONE',  ( -19.50000000000000000, -11.50000000000000000, 29.75000000000000355 ) ) ;
#22115=ORIENTED_EDGE ( 'NONE', *, *, #14548, .F. ) ;
#22122=EDGE_CURVE ( 'NONE', #81634, #18370, #49210, .T. ) ;
#22132=EDGE_LOOP ( 'NONE', ( #24283, #43612, #54464, #81921 ) ) ;
#22133=DIRECTION ( 'NONE',  ( -1.000000000000000000, 0.000000000000000000, -0.000000000000000000 ) ) ;
#22141=CARTESIAN_POINT ( 'NONE',  ( -10.03846153846153832, -1.926643599941765039, 28.25000000000000000 ) ) ;
#22147=ORIENTED_EDGE ( 'NONE', *, *, #73999, .F. ) ;
#22186=CARTESIAN_POINT ( 'NONE',  ( -11.00641025641025550, -3.499999999999999556, 29.75000000000000355 ) ) ;
#22187=LINE ( 'NONE', #83457, #36733 ) ;
#22192=DIRECTION ( 'NONE',  ( -1.000000000000000000, -0.000000000000000000, -0.000000000000000000 ) ) ;
#22206=DIRECTION ( 'NONE',  ( -1.000000000000000000, -0.000000000000000000, -0.000000000000000000 ) ) ;
#22218=VERTEX_POINT ( 'NONE', #18094 ) ;
#22219=ORIENTED_EDGE ( 'NONE', *, *, #16353, .F. ) ;
#22233=DIRECTION ( 'NONE',  ( 1.000000000000000000, 0.000000000000000000, 0.000000000000000000 ) ) ;
#22240=VERTEX_POINT ( 'NONE', #6784 ) ;
#22252=DIRECTION ( 'NONE',  ( -1.000000000000000000, -0.000000000000000000, -0.000000000000000000 ) ) ;
#22262=VECTOR ( 'NONE', #82450, 1000.000000000000000 ) ;
#22283=ADVANCED_FACE ( 'NONE', ( #42805 ), #55858, .F. ) ;
#22289=CARTESIAN_POINT ( 'NONE',  ( 0.000000000000000000, -11.00000000000000000, 29.75000000000000355 ) ) ;
#22295=DIRECTION ( 'NONE',  ( 1.000000000000000000, 0.000000000000000000, 0.000000000000000000 ) ) ;
#22298=AXIS2_PLACEMENT_3D ( 'NONE', #66635, #34172, #75597 ) ;
#22326=DIRECTION ( 'NONE',  ( -1.000000000000000000, -0.000000000000000000, -0.000000000000000000 ) ) ;
#22346=CARTESIAN_POINT ( 'NONE',  ( -19.50000000000000000, -3.499999999999999556, 29.75000000000000355 ) ) ;
#22370=DIRECTION ( 'NONE',  ( 0.000000000000000000, 0.000000000000000000, -1.000000000000000000 ) ) ;
#22374=ORIENTED_EDGE ( 'NONE', *, *, #26438, .F. ) ;
#22381=CARTESIAN_POINT ( 'NONE',  ( 4.480769230769229061, -7.500000000000000000, 29.75000000000000355 ) ) ;
#22393=DIRECTION ( 'NONE',  ( 0.000000000000000000, 0.000000000000000000, 1.000000000000000000 ) ) ;
#22400=CIRCLE ( 'NONE', #15211, 4.000000000000000000 ) ;
#22402=ORIENTED_EDGE ( 'NONE', *, *, #25917, .T. ) ;
#22411=CARTESIAN_POINT ( 'NONE',  ( -19.50000000000000000, -3.499999999999999556, 29.75000000000000355 ) ) ;
#22412=DIRECTION ( 'NONE',  ( 0.000000000000000000, 0.000000000000000000, -1.000000000000000000 ) ) ;
#22433=CARTESIAN_POINT ( 'NONE',  ( -19.50000000000000000, -3.499999999999999556, 29.75000000000000355 ) ) ;
#22438=ORIENTED_EDGE ( 'NONE', *, *, #8573, .T. ) ;
#22457=EDGE_CURVE ( 'NONE', #13929, #1333, #72920, .T. ) ;
#22461=ORIENTED_EDGE ( 'NONE', *, *, #55685, .T. ) ;
#22463=EDGE_CURVE ( 'NONE', #75823, #43796, #12835, .T. ) ;
#22478=ORIENTED_EDGE ( 'NONE', *, *, #38447, .F. ) ;
#22515=ORIENTED_EDGE ( 'NONE', *, *, #53126, .F. ) ;
#22521=DIRECTION ( 'NONE',  ( -0.000000000000000000, 1.000000000000000000, -0.000000000000000000 ) ) ;
#22553=AXIS2_PLACEMENT_3D ( 'NONE', #15549, #55632, #36703 ) ;
#22579=VECTOR ( 'NONE', #84839, 1000.000000000000000 ) ;
#22593=CARTESIAN_POINT ( 'NONE',  ( -18.03205128205128105, -11.50000000000000000, 29.75000000000000355 ) ) ;
#22595=CARTESIAN_POINT ( 'NONE',  ( 11.25641025641025550, -7.500000000000000000, 29.75000000000000355 ) ) ;
#22596=CARTESIAN_POINT ( 'NONE',  ( 9.320512820512821150, -3.499999999999999556, 29.75000000000000355 ) ) ;
#22600=VECTOR ( 'NONE', #41006, 1000.000000000000000 ) ;
#22615=AXIS2_PLACEMENT_3D ( 'NONE', #45474, #30626, #72501 ) ;
#22635=VERTEX_POINT ( 'NONE', #68826 ) ;
#22640=CARTESIAN_POINT ( 'NONE',  ( -1.326923076923076872, -11.00000000000000000, 29.75000000000000355 ) ) ;
#22644=CARTESIAN_POINT ( 'NONE',  ( -19.50000000000000000, -11.50000000000000000, 29.75000000000000355 ) ) ;
#22657=VECTOR ( 'NONE', #64516, 1000.000000000000000 ) ;
#22669=DIRECTION ( 'NONE',  ( 0.000000000000000000, 0.000000000000000000, 1.000000000000000000 ) ) ;
#22670=LINE ( 'NONE', #49702, #22579 ) ;
#22678=ORIENTED_EDGE ( 'NONE', *, *, #20072, .F. ) ;
#22682=AXIS2_PLACEMENT_3D ( 'NONE', #77040, #71153, #15341 ) ;
#22684=DIRECTION ( 'NONE',  ( 1.000000000000000000, 0.000000000000000000, 0.000000000000000000 ) ) ;
#22686=AXIS2_PLACEMENT_3D ( 'NONE', #38623, #3048, #66082 ) ;
#22708=EDGE_CURVE ( 'NONE', #17208, #82422, #8465, .T. ) ;
#22723=CARTESIAN_POINT ( 'NONE',  ( -19.50000000000000000, -3.499999999999999556, 29.75000000000000355 ) ) ;
#22729=EDGE_CURVE ( 'NONE', #18077, #57194, #84793, .T. ) ;
#22745=CARTESIAN_POINT ( 'NONE',  ( -1.576923076923076428, -3.499999999999999556, 29.75000000000000355 ) ) ;
#22750=EDGE_CURVE ( 'NONE', #78293, #50090, #76919, .T. ) ;
#22751=DIRECTION ( 'NONE',  ( -0.000000000000000000, 1.000000000000000000, -0.000000000000000000 ) ) ;
#22752=ORIENTED_EDGE ( 'NONE', *, *, #55497, .T. ) ;
#22777=CARTESIAN_POINT ( 'NONE',  ( -20.00000000000000000, -11.50000000000000000, 29.75000000000000355 ) ) ;
#22780=DIRECTION ( 'NONE',  ( 1.000000000000000000, 0.000000000000000000, 0.000000000000000000 ) ) ;
#22785=ORIENTED_EDGE ( 'NONE', *, *, #11739, .F. ) ;
#22788=CARTESIAN_POINT ( 'NONE',  ( 7.134615384615385025, -7.500000000000000000, 29.75000000000000355 ) ) ;
#22795=EDGE_LOOP ( 'NONE', ( #49670, #69749, #63124, #53664, #38911 ) ) ;
#22798=VECTOR ( 'NONE', #37185, 1000.000000000000000 ) ;
#22811=ORIENTED_EDGE ( 'NONE', *, *, #22912, .T. ) ;
#22828=DIRECTION ( 'NONE',  ( 1.000000000000000000, 0.000000000000000000, 0.000000000000000000 ) ) ;
#22837=EDGE_CURVE ( 'NONE', #18370, #80137, #38140, .T. ) ;
#22846=DIRECTION ( 'NONE',  ( 1.000000000000000000, 0.000000000000000000, 0.000000000000000000 ) ) ;
#22874=CARTESIAN_POINT ( 'NONE',  ( 6.166666666666664298, -11.50000000000000000, 29.75000000000000355 ) ) ;
#22883=DIRECTION ( 'NONE',  ( -0.000000000000000000, 1.000000000000000000, -0.000000000000000000 ) ) ;
#22901=ORIENTED_EDGE ( 'NONE', *, *, #16779, .F. ) ;
#22912=EDGE_CURVE ( 'NONE', #34205, #856, #52534, .T. ) ;
#22921=EDGE_CURVE ( 'NONE', #55647, #32571, #39933, .T. ) ;
#22922=ORIENTED_EDGE ( 'NONE', *, *, #52688, .F. ) ;
#22931=LINE ( 'NONE', #27589, #47978 ) ;
#22947=LINE ( 'NONE', #71130, #86408 ) ;
#22949=EDGE_CURVE ( 'NONE', #19931, #65515, #31604, .T. ) ;
#22960=AXIS2_PLACEMENT_3D ( 'NONE', #54873, #19759, #27402 ) ;
#22983=LINE ( 'NONE', #22107, #62290 ) ;
#22999=AXIS2_PLACEMENT_3D ( 'NONE', #52062, #11987, #17853 ) ;
#23002=EDGE_CURVE ( 'NONE', #77088, #24805, #6135, .T. ) ;
#23021=DIRECTION ( 'NONE',  ( 0.000000000000000000, -1.000000000000000000, 0.000000000000000000 ) ) ;
#23026=ORIENTED_EDGE ( 'NONE', *, *, #23071, .T. ) ;
#23027=LINE ( 'NONE', #56809, #14138 ) ;
#23032=ORIENTED_EDGE ( 'NONE', *, *, #13385, .T. ) ;
#23038=VECTOR ( 'NONE', #53062, 1000.000000000000000 ) ;
#23040=CARTESIAN_POINT ( 'NONE',  ( 0.000000000000000000, -11.00000000000000000, 29.75000000000000355 ) ) ;
#23049=CARTESIAN_POINT ( 'NONE',  ( -19.50000000000000000, -3.499999999999999556, 29.75000000000000355 ) ) ;
#23065=ORIENTED_EDGE ( 'NONE', *, *, #61590, .T. ) ;
#23070=VERTEX_POINT ( 'NONE', #62827 ) ;
#23071=EDGE_CURVE ( 'NONE', #7366, #68357, #46001, .T. ) ;
#23076=CARTESIAN_POINT ( 'NONE',  ( -16.81410256410256565, -3.499999999999999556, 29.75000000000000355 ) ) ;
#23087=DIRECTION ( 'NONE',  ( -1.000000000000000000, 0.000000000000000000, -0.000000000000000000 ) ) ;
#23094=FACE_OUTER_BOUND ( 'NONE', #29583, .T. ) ;
#23095=AXIS2_PLACEMENT_3D ( 'NONE', #25438, #86270, #52895 ) ;
#23099=CARTESIAN_POINT ( 'NONE',  ( 16.81410256410256565, -3.499999999999999556, 29.75000000000000355 ) ) ;
#23114=AXIS2_PLACEMENT_3D ( 'NONE', #6134, #5245, #39491 ) ;
#23119=VECTOR ( 'NONE', #7093, 1000.000000000000000 ) ;
#23135=EDGE_CURVE ( 'NONE', #49385, #71780, #81972, .T. ) ;
#23138=PLANE ( 'NONE',  #59471 ) ;
#23159=ORIENTED_EDGE ( 'NONE', *, *, #88924, .F. ) ;
#23167=AXIS2_PLACEMENT_3D ( 'NONE', #81705, #19988, #40722 ) ;
#23181=LINE ( 'NONE', #50643, #29913 ) ;
#23193=DIRECTION ( 'NONE',  ( -1.000000000000000000, -0.000000000000000000, -0.000000000000000000 ) ) ;
#23209=LINE ( 'NONE', #3826, #41768 ) ;
#23210=LINE ( 'NONE', #16017, #54712 ) ;
#23225=DIRECTION ( 'NONE',  ( 0.000000000000000000, 0.000000000000000000, -1.000000000000000000 ) ) ;
#23228=CARTESIAN_POINT ( 'NONE',  ( -19.50000000000000000, -3.499999999999999556, 29.75000000000000355 ) ) ;
#23229=EDGE_CURVE ( 'NONE', #58726, #63997, #64162, .T. ) ;
#23231=ORIENTED_EDGE ( 'NONE', *, *, #54826, .F. ) ;
#23250=CARTESIAN_POINT ( 'NONE',  ( -9.070512820512819374, -7.500000000000000000, 29.75000000000000355 ) ) ;
#23255=ORIENTED_EDGE ( 'NONE', *, *, #26323, .F. ) ;
#23258=DIRECTION ( 'NONE',  ( -1.000000000000000000, -0.000000000000000000, 0.000000000000000000 ) ) ;
#23263=ORIENTED_EDGE ( 'NONE', *, *, #23071, .F. ) ;
#23265=AXIS2_PLACEMENT_3D ( 'NONE', #37057, #29878, #3275 ) ;
#23266=LINE ( 'NONE', #78211, #49724 ) ;
#23270=CARTESIAN_POINT ( 'NONE',  ( 4.230769230769229061, -7.500000000000000000, 29.75000000000000355 ) ) ;
#23278=EDGE_CURVE ( 'NONE', #79307, #84442, #87143, .T. ) ;
#23282=DIRECTION ( 'NONE',  ( -1.000000000000000000, -0.000000000000000000, -0.000000000000000000 ) ) ;
#23294=CYLINDRICAL_SURFACE ( 'NONE', #7390, 4.000000000000000000 ) ;
#23310=CARTESIAN_POINT ( 'NONE',  ( 9.320512820512821150, -3.499999999999999556, 29.75000000000000355 ) ) ;
#23323=FACE_OUTER_BOUND ( 'NONE', #68027, .T. ) ;
#23328=EDGE_CURVE ( 'NONE', #60613, #74633, #65508, .T. ) ;
#23333=VECTOR ( 'NONE', #64380, 1000.000000000000000 ) ;
#23335=CARTESIAN_POINT ( 'NONE',  ( -5.198717948717948012, -7.500000000000000000, 29.75000000000000355 ) ) ;
#23344=ADVANCED_FACE ( 'NONE', ( #58754 ), #86249, .F. ) ;
#23346=CARTESIAN_POINT ( 'NONE',  ( -10.03846153846153832, -7.500000000000000000, 29.75000000000000355 ) ) ;
#23353=AXIS2_PLACEMENT_3D ( 'NONE', #33068, #26752, #11920 ) ;
#23364=ADVANCED_FACE ( 'NONE', ( #61854 ), #41596, .T. ) ;
#23382=VERTEX_POINT ( 'NONE', #55547 ) ;
#23385=CIRCLE ( 'NONE', #70867, 4.000000000000000000 ) ;
#23401=ADVANCED_FACE ( 'NONE', ( #47454 ), #41157, .T. ) ;
#23417=PLANE ( 'NONE',  #77816 ) ;
#23420=DIRECTION ( 'NONE',  ( 0.000000000000000000, 0.000000000000000000, -1.000000000000000000 ) ) ;
#23429=AXIS2_PLACEMENT_3D ( 'NONE', #56159, #36768, #15621 ) ;
#23442=DIRECTION ( 'NONE',  ( 0.000000000000000000, 0.000000000000000000, -1.000000000000000000 ) ) ;
#23452=EDGE_CURVE ( 'NONE', #13160, #21459, #64762, .T. ) ;
#23465=ORIENTED_EDGE ( 'NONE', *, *, #78074, .T. ) ;
#23474=DIRECTION ( 'NONE',  ( -1.000000000000000000, -0.000000000000000000, 0.000000000000000000 ) ) ;
#23479=EDGE_CURVE ( 'NONE', #3262, #84195, #57320, .T. ) ;
#23489=CARTESIAN_POINT ( 'NONE',  ( 4.480769230769229061, -4.000000000000000000, 29.75000000000000355 ) ) ;
#23490=CARTESIAN_POINT ( 'NONE',  ( 0.6089743589743589203, -4.000000000000000000, 29.75000000000000355 ) ) ;
#23492=DIRECTION ( 'NONE',  ( -0.000000000000000000, 1.000000000000000000, -0.000000000000000000 ) ) ;
#23496=ORIENTED_EDGE ( 'NONE', *, *, #29613, .T. ) ;
#23497=DIRECTION ( 'NONE',  ( 1.000000000000000000, 0.000000000000000000, 0.000000000000000000 ) ) ;
#23517=VECTOR ( 'NONE', #45042, 1000.000000000000000 ) ;
#23520=VERTEX_POINT ( 'NONE', #45006 ) ;
#23525=CARTESIAN_POINT ( 'NONE',  ( -5.198717948717948012, -3.499999999999999556, 29.75000000000000355 ) ) ;
#23529=EDGE_CURVE ( 'NONE', #5501, #13929, #33144, .T. ) ;
#23533=ORIENTED_EDGE ( 'NONE', *, *, #15133, .F. ) ;
#23542=VERTEX_POINT ( 'NONE', #58973 ) ;
#23572=ORIENTED_EDGE ( 'NONE', *, *, #82150, .F. ) ;
#23584=CARTESIAN_POINT ( 'NONE',  ( 5.448717948717947124, -3.499999999999999556, 29.75000000000000355 ) ) ;
#23586=CARTESIAN_POINT ( 'NONE',  ( 18.03205128205128105, -11.50000000000000000, 29.75000000000000355 ) ) ;
#23596=LINE ( 'NONE', #2869, #10005 ) ;
#23605=LINE ( 'NONE', #26279, #48576 ) ;
#23618=CARTESIAN_POINT ( 'NONE',  ( -5.198717948717948012, -3.499999999999999556, 29.75000000000000355 ) ) ;
#23619=VERTEX_POINT ( 'NONE', #6269 ) ;
#23642=EDGE_CURVE ( 'NONE', #6970, #79996, #88700, .T. ) ;
#23645=DIRECTION ( 'NONE',  ( 0.000000000000000000, 0.000000000000000000, 1.000000000000000000 ) ) ;
#23648=EDGE_CURVE ( 'NONE', #74633, #52479, #26981, .T. ) ;
#23652=VECTOR ( 'NONE', #12233, 1000.000000000000000 ) ;
#23663=LINE ( 'NONE', #51116, #1148 ) ;
#23698=DIRECTION ( 'NONE',  ( 1.000000000000000000, 0.000000000000000000, 0.000000000000000000 ) ) ;
#23703=ORIENTED_EDGE ( 'NONE', *, *, #45447, .F. ) ;
#23711=ORIENTED_EDGE ( 'NONE', *, *, #72858, .F. ) ;
#23724=CARTESIAN_POINT ( 'NONE',  ( -19.50000000000000000, -3.499999999999999556, 29.75000000000000355 ) ) ;
#23732=ORIENTED_EDGE ( 'NONE', *, *, #80, .F. ) ;
#23735=DIRECTION ( 'NONE',  ( 0.000000000000000000, -1.000000000000000000, 0.000000000000000000 ) ) ;
#23751=PLANE ( 'NONE',  #65780 ) ;
#23761=DIRECTION ( 'NONE',  ( -1.000000000000000000, -0.000000000000000000, -0.000000000000000000 ) ) ;
#23805=DIRECTION ( 'NONE',  ( 1.000000000000000000, 0.000000000000000000, 0.000000000000000000 ) ) ;
#23808=CARTESIAN_POINT ( 'NONE',  ( -2.544871794871794268, -7.500000000000000000, 29.75000000000000355 ) ) ;
#23812=ORIENTED_EDGE ( 'NONE', *, *, #66122, .F. ) ;
#23816=EDGE_CURVE ( 'NONE', #76951, #19931, #24527, .T. ) ;
#23830=EDGE_LOOP ( 'NONE', ( #76973, #25363, #59895, #40704 ) ) ;
#23879=DIRECTION ( 'NONE',  ( 1.000000000000000000, 0.000000000000000000, 0.000000000000000000 ) ) ;
#23882=DIRECTION ( 'NONE',  ( -1.000000000000000000, -0.000000000000000000, -0.000000000000000000 ) ) ;
#23897=ORIENTED_EDGE ( 'NONE', *, *, #85198, .F. ) ;
#23931=LINE ( 'NONE', #50947, #78755 ) ;
#23938=CARTESIAN_POINT ( 'NONE',  ( 10.03846153846153832, -11.50000000000000000, 29.75000000000000355 ) ) ;
#23946=ORIENTED_EDGE ( 'NONE', *, *, #13960, .F. ) ;
#23970=DIRECTION ( 'NONE',  ( 1.000000000000000000, 0.000000000000000000, 0.000000000000000000 ) ) ;
#23996=FACE_OUTER_BOUND ( 'NONE', #17616, .T. ) ;
#23999=EDGE_CURVE ( 'NONE', #17208, #15714, #62845, .T. ) ;
#24002=DIRECTION ( 'NONE',  ( -1.000000000000000000, 0.000000000000000000, -0.000000000000000000 ) ) ;
#24012=CARTESIAN_POINT ( 'NONE',  ( -11.97435897435897267, -3.499999999999999556, 29.75000000000000355 ) ) ;
#24013=CYLINDRICAL_SURFACE ( 'NONE', #18570, 4.000000000000000000 ) ;
#24028=CARTESIAN_POINT ( 'NONE',  ( -6.416666666666667851, -11.00000000000000000, 29.75000000000000355 ) ) ;
#24038=EDGE_CURVE ( 'NONE', #46042, #80082, #37436, .T. ) ;
#24039=ORIENTED_EDGE ( 'NONE', *, *, #39883, .T. ) ;
#24048=DIRECTION ( 'NONE',  ( 0.000000000000000000, 0.000000000000000000, -1.000000000000000000 ) ) ;
#24058=VECTOR ( 'NONE', #31411, 1000.000000000000000 ) ;
#24074=EDGE_CURVE ( 'NONE', #21038, #33780, #7244, .T. ) ;
#24085=VECTOR ( 'NONE', #54958, 1000.000000000000000 ) ;
#24086=ORIENTED_EDGE ( 'NONE', *, *, #52712, .T. ) ;
#24087=LINE ( 'NONE', #70952, #88746 ) ;
#24131=EDGE_CURVE ( 'NONE', #35014, #23070, #23209, .T. ) ;
#24134=VECTOR ( 'NONE', #53528, 1000.000000000000000 ) ;
#24136=EDGE_CURVE ( 'NONE', #11498, #35739, #71388, .T. ) ;
#24142=VECTOR ( 'NONE', #50434, 1000.000000000000000 ) ;
#24167=DIRECTION ( 'NONE',  ( -1.000000000000000000, -0.000000000000000000, 0.000000000000000000 ) ) ;
#24190=DIRECTION ( 'NONE',  ( -1.000000000000000000, -0.000000000000000000, -0.000000000000000000 ) ) ;
#24202=CARTESIAN_POINT ( 'NONE',  ( -0.3589743589743593088, -3.499999999999999556, 29.75000000000000355 ) ) ;
#24210=CARTESIAN_POINT ( 'NONE',  ( 15.84615384615384670, -3.499999999999999556, 29.75000000000000355 ) ) ;
#24217=VECTOR ( 'NONE', #68504, 1000.000000000000000 ) ;
#24219=CLOSED_SHELL ( 'NONE', ( #72577, #75317, #79081, #79121, #70166, #48705, #83284, #35996, #52238, #57899, #59276, #59206, #68998, #65103, #23364, #62457, #24985, #31495, #25791, #48204, #65810, #30859, #59576, #46365, #74433, #65543, #377, #66666, #49380, #16246, #78857, #58243, #7969, #84139, #53251, #87559, #71495, #12469, #43103, #58407, #1031, #83320, #83514, #76791, #87832, #74737, #44335, #83469, #55359, #59873, #51357, #50168, #47850, #68474, #35112, #45383, #22283, #68067, #4294, #31820, #4693, #30976, #49508, #76155, #69576, #25257, #5091, #87322, #88743, #44273, #16908, #74082, #59074, #37290, #64487, #10612, #41087, #29905, #26160, #2576, #35233, #79574, #40672, #9730, #4790, #52684, #27427, #15885, #47970, #2915, #75750, #12090, #32253, #77071, #30491, #68929, #29557, #1501, #12183, #56287, #33442, #3195, #79469, #47541, #76769, #69414, #71425, #44464, #26881, #41982, #85890, #43846, #42189, #71240, #75327, #1877, #2319, #68333, #23344, #89002, #12047, #88950, #60919, #84920, #11155, #77346, #73118, #27298, #86193, #79305, #82959, #21912, #86262, #10135, #25137, #41467, #85758, #33557, #37985, #32097, #55916, #6918, #27450, #21819, #75648, #19313, #16327, #37114, #21027, #77201, #36971, #19029, #11807, #73010, #62317, #10743, #71666, #61305, #35247, #86709, #27910, #21701, #60164, #44382, #62443, #6169, #34650, #31125, #51983, #85796, #6064, #54933, #2620, #20336, #38783, #1908, #3235, #25810, #12256, #55822, #16933, #75745, #65353, #21340, #39868, #63933, #47519, #17265, #75273, #68777, #52131, #43572, #59730, #46082, #16158, #16163, #64775, #45885, #77385, #9174, #505, #5055, #32306, #61072, #44669, #31268, #14438, #30649, #56481, #26309, #11856, #25815, #8729, #70671, #43618, #28569, #6939, #84590, #57029, #4763, #181, #62775, #72318, #60456, #45378, #32029, #38985, #69075, #52436, #37503, #65936, #83966, #73478, #82671, #20161, #62705, #79394, #68687, #52066, #70127, #85913, #37102, #45632, #38534, #87427, #74096, #75497, #29507, #49369, #82643, #72755, #63907, #9647, #34974, #51114, #75661, #75415, #25564, #17165, #42686, #5743, #61573, #51375, #28119, #28452, #66480, #21556, #81220, #36995, #79049, #12869, #62455, #55679, #6433, #15313, #39044, #19394, #81271, #63976, #9049, #79710, #20794, #48378, #5184, #28220, #55104, #68989, #30000, #85006, #71420, #8633, #41499, #2191, #85963, #68654, #28421, #84068, #51464, #67549, #23401, #41780, #42659, #85399 ) ) ;
#24223=ORIENTED_EDGE ( 'NONE', *, *, #36445, .T. ) ;
#24239=ORIENTED_EDGE ( 'NONE', *, *, #38614, .F. ) ;
#24251=FACE_OUTER_BOUND ( 'NONE', #8124, .T. ) ;
#24268=AXIS2_PLACEMENT_3D ( 'NONE', #40939, #76043, #40507 ) ;
#24272=ORIENTED_EDGE ( 'NONE', *, *, #35449, .T. ) ;
#24280=DIRECTION ( 'NONE',  ( -1.000000000000000000, 0.000000000000000000, -0.000000000000000000 ) ) ;
#24283=ORIENTED_EDGE ( 'NONE', *, *, #56784, .F. ) ;
#24285=VERTEX_POINT ( 'NONE', #60993 ) ;
#24288=EDGE_CURVE ( 'NONE', #17254, #4690, #59214, .T. ) ;
#24297=ORIENTED_EDGE ( 'NONE', *, *, #83655, .F. ) ;
#24343=ORIENTED_EDGE ( 'NONE', *, *, #29120, .F. ) ;
#24346=ORIENTED_EDGE ( 'NONE', *, *, #19916, .F. ) ;
#24371=ORIENTED_EDGE ( 'NONE', *, *, #26628, .F. ) ;
#24390=ORIENTED_EDGE ( 'NONE', *, *, #31781, .T. ) ;
#24400=AXIS2_PLACEMENT_3D ( 'NONE', #37704, #50323, #44898 ) ;
#24417=EDGE_LOOP ( 'NONE', ( #9960, #79627, #50621, #51237 ) ) ;
#24427=EDGE_CURVE ( 'NONE', #44538, #2392, #47534, .T. ) ;
#24463=AXIS2_PLACEMENT_3D ( 'NONE', #31359, #51597, #25931 ) ;
#24480=ORIENTED_EDGE ( 'NONE', *, *, #19197, .F. ) ;
#24481=DIRECTION ( 'NONE',  ( -0.000000000000000000, 1.000000000000000000, -0.000000000000000000 ) ) ;
#24498=ORIENTED_EDGE ( 'NONE', *, *, #26771, .F. ) ;
#24500=DIRECTION ( 'NONE',  ( -1.000000000000000000, -0.000000000000000000, -0.000000000000000000 ) ) ;
#24507=ORIENTED_EDGE ( 'NONE', *, *, #42568, .T. ) ;
#24510=ORIENTED_EDGE ( 'NONE', *, *, #27140, .T. ) ;
#24516=FACE_OUTER_BOUND ( 'NONE', #10341, .T. ) ;
#24518=DIRECTION ( 'NONE',  ( 0.000000000000000000, 0.000000000000000000, -1.000000000000000000 ) ) ;
#24522=EDGE_CURVE ( 'NONE', #2843, #66098, #37493, .T. ) ;
#24527=CIRCLE ( 'NONE', #40355, 4.000000000000000000 ) ;
#24532=VERTEX_POINT ( 'NONE', #57333 ) ;
#24533=DIRECTION ( 'NONE',  ( -1.000000000000000000, -0.000000000000000000, -0.000000000000000000 ) ) ;
#24536=CIRCLE ( 'NONE', #36063, 4.000000000000000000 ) ;
#24545=EDGE_CURVE ( 'NONE', #50957, #58964, #86601, .T. ) ;
#24551=EDGE_CURVE ( 'NONE', #5501, #85209, #11821, .T. ) ;
#24555=CARTESIAN_POINT ( 'NONE',  ( -19.50000000000000000, -3.499999999999999556, 29.75000000000000355 ) ) ;
#24557=DIRECTION ( 'NONE',  ( 1.000000000000000000, 0.000000000000000000, 0.000000000000000000 ) ) ;
#24565=VECTOR ( 'NONE', #79162, 1000.000000000000000 ) ;
#24576=EDGE_CURVE ( 'NONE', #17369, #43749, #32083, .T. ) ;
#24579=ORIENTED_EDGE ( 'NONE', *, *, #28553, .F. ) ;
#24580=VECTOR ( 'NONE', #87800, 1000.000000000000000 ) ;
#24584=AXIS2_PLACEMENT_3D ( 'NONE', #35452, #7543, #15186 ) ;
#24585=AXIS2_PLACEMENT_3D ( 'NONE', #32169, #49871, #85439 ) ;
#24592=ORIENTED_EDGE ( 'NONE', *, *, #53689, .F. ) ;
#24596=PLANE ( 'NONE',  #22999 ) ;
#24597=DIRECTION ( 'NONE',  ( 1.000000000000000000, 0.000000000000000000, 0.000000000000000000 ) ) ;
#24621=CARTESIAN_POINT ( 'NONE',  ( -18.03205128205128105, -11.00000000000000000, 29.75000000000000355 ) ) ;
#24626=CARTESIAN_POINT ( 'NONE',  ( -19.50000000000000000, -3.499999999999999556, 29.75000000000000355 ) ) ;
#24630=VECTOR ( 'NONE', #69413, 1000.000000000000000 ) ;
#24636=EDGE_CURVE ( 'NONE', #58140, #35531, #3102, .T. ) ;
#24651=LINE ( 'NONE', #53902, #61474 ) ;
#24653=CARTESIAN_POINT ( 'NONE',  ( 9.070512820512819374, -4.000000000000000000, 29.75000000000000355 ) ) ;
#24656=EDGE_CURVE ( 'NONE', #21434, #58816, #36464, .T. ) ;
#24657=CIRCLE ( 'NONE', #70631, 4.000000000000000000 ) ;
#24672=EDGE_CURVE ( 'NONE', #29224, #54838, #44972, .T. ) ;
#24691=ORIENTED_EDGE ( 'NONE', *, *, #18270, .F. ) ;
#24693=VECTOR ( 'NONE', #16790, 1000.000000000000000 ) ;
#24695=DIRECTION ( 'NONE',  ( 0.000000000000000000, 0.000000000000000000, -1.000000000000000000 ) ) ;
#24718=AXIS2_PLACEMENT_3D ( 'NONE', #29903, #75863, #8302 ) ;
#24740=VERTEX_POINT ( 'NONE', #25160 ) ;
#24742=LINE ( 'NONE', #4476, #23333 ) ;
#24760=CARTESIAN_POINT ( 'NONE',  ( 13.19230769230769340, -7.500000000000000000, 33.75000000000000000 ) ) ;
#24785=ORIENTED_EDGE ( 'NONE', *, *, #43695, .F. ) ;
#24794=LINE ( 'NONE', #3629, #31999 ) ;
#24803=CARTESIAN_POINT ( 'NONE',  ( 3.262820512820511443, -3.499999999999999556, 29.75000000000000355 ) ) ;
#24804=DIRECTION ( 'NONE',  ( -0.000000000000000000, 1.000000000000000000, -0.000000000000000000 ) ) ;
#24805=VERTEX_POINT ( 'NONE', #74694 ) ;
#24808=ORIENTED_EDGE ( 'NONE', *, *, #55789, .T. ) ;
#24809=AXIS2_PLACEMENT_3D ( 'NONE', #33172, #66519, #12026 ) ;
#24827=CARTESIAN_POINT ( 'NONE',  ( -1.326923076923076872, -7.500000000000000000, 29.75000000000000355 ) ) ;
#24828=PLANE ( 'NONE',  #58755 ) ;
#24839=ORIENTED_EDGE ( 'NONE', *, *, #32593, .T. ) ;
#24846=DIRECTION ( 'NONE',  ( -0.000000000000000000, 0.000000000000000000, 1.000000000000000000 ) ) ;
#24848=VECTOR ( 'NONE', #18046, 1000.000000000000000 ) ;
#24881=CARTESIAN_POINT ( 'NONE',  ( -19.00000000000000000, -7.500000000000000000, 33.75000000000000000 ) ) ;
#24890=VERTEX_POINT ( 'NONE', #60259 ) ;
#24892=FACE_OUTER_BOUND ( 'NONE', #71462, .T. ) ;
#24893=CARTESIAN_POINT ( 'NONE',  ( 1.326923076923075762, -7.500000000000000000, 29.75000000000000355 ) ) ;
#24895=DIRECTION ( 'NONE',  ( -1.000000000000000000, -0.000000000000000000, 0.000000000000000000 ) ) ;
#24899=EDGE_CURVE ( 'NONE', #56816, #26148, #81882, .T. ) ;
#24907=LINE ( 'NONE', #60026, #17137 ) ;
#24913=ORIENTED_EDGE ( 'NONE', *, *, #56571, .T. ) ;
#24921=DIRECTION ( 'NONE',  ( -1.000000000000000000, -0.000000000000000000, -0.000000000000000000 ) ) ;
#24923=DIRECTION ( 'NONE',  ( 1.000000000000000000, 0.000000000000000000, 0.000000000000000000 ) ) ;
#24943=VERTEX_POINT ( 'NONE', #48069 ) ;
#24947=DIRECTION ( 'NONE',  ( 1.000000000000000000, 0.000000000000000000, 0.000000000000000000 ) ) ;
#24950=CARTESIAN_POINT ( 'NONE',  ( -20.00000000000000000, -7.500000000000000000, 29.75000000000000355 ) ) ;
#24970=DIRECTION ( 'NONE',  ( -0.000000000000000000, 1.000000000000000000, -0.000000000000000000 ) ) ;
#24985=ADVANCED_FACE ( 'NONE', ( #75992 ), #76441, .T. ) ;
#24989=LINE ( 'NONE', #53347, #57580 ) ;
#24991=FACE_OUTER_BOUND ( 'NONE', #88723, .T. ) ;
#25007=VECTOR ( 'NONE', #19855, 1000.000000000000000 ) ;
#25011=ORIENTED_EDGE ( 'NONE', *, *, #39153, .T. ) ;
#25012=EDGE_CURVE ( 'NONE', #58001, #18170, #36342, .T. ) ;
#25018=EDGE_CURVE ( 'NONE', #5565, #79802, #27435, .T. ) ;
#25027=EDGE_CURVE ( 'NONE', #43796, #21320, #41326, .T. ) ;
#25034=DIRECTION ( 'NONE',  ( 0.000000000000000000, 0.000000000000000000, 1.000000000000000000 ) ) ;
#25037=ORIENTED_EDGE ( 'NONE', *, *, #26323, .T. ) ;
#25051=DIRECTION ( 'NONE',  ( 0.000000000000000000, 0.000000000000000000, -1.000000000000000000 ) ) ;
#25056=EDGE_CURVE ( 'NONE', #31713, #72564, #38451, .T. ) ;
#25064=EDGE_CURVE ( 'NONE', #50717, #14174, #60540, .T. ) ;
#25067=DIRECTION ( 'NONE',  ( -0.000000000000000000, 1.000000000000000000, -0.000000000000000000 ) ) ;
#25083=LINE ( 'NONE', #73275, #2792 ) ;
#25114=LINE ( 'NONE', #59339, #16929 ) ;
#25123=ORIENTED_EDGE ( 'NONE', *, *, #24636, .T. ) ;
#25136=LINE ( 'NONE', #60248, #54556 ) ;
#25137=ADVANCED_FACE ( 'NONE', ( #79881 ), #5554, .F. ) ;
#25144=CARTESIAN_POINT ( 'NONE',  ( -19.50000000000000000, -3.499999999999999556, 29.75000000000000355 ) ) ;
#25154=EDGE_CURVE ( 'NONE', #53616, #30978, #46538, .T. ) ;
#25155=CYLINDRICAL_SURFACE ( 'NONE', #35605, 4.000000000000000000 ) ;
#25160=CARTESIAN_POINT ( 'NONE',  ( 0.3589743589743586982, -11.50000000000000000, 29.75000000000000355 ) ) ;
#25162=FACE_OUTER_BOUND ( 'NONE', #21348, .T. ) ;
#25163=EDGE_LOOP ( 'NONE', ( #13803, #8434, #1029, #24913 ) ) ;
#25174=CARTESIAN_POINT ( 'NONE',  ( -5.198717948717948012, -3.499999999999999556, 29.75000000000000355 ) ) ;
#25178=EDGE_CURVE ( 'NONE', #68357, #75345, #24657, .T. ) ;
#25198=AXIS2_PLACEMENT_3D ( 'NONE', #72597, #15898, #23087 ) ;
#25214=LINE ( 'NONE', #65302, #57742 ) ;
#25221=DIRECTION ( 'NONE',  ( -1.000000000000000000, 0.000000000000000000, -0.000000000000000000 ) ) ;
#25234=FACE_OUTER_BOUND ( 'NONE', #59474, .T. ) ;
#25257=ADVANCED_FACE ( 'NONE', ( #9529 ), #63589, .F. ) ;
#25259=CARTESIAN_POINT ( 'NONE',  ( -9.320512820512821150, -11.00000000000000000, 29.25000000000000000 ) ) ;
#25268=PLANE ( 'NONE',  #29761 ) ;
#25270=FACE_OUTER_BOUND ( 'NONE', #74088, .T. ) ;
#25275=EDGE_CURVE ( 'NONE', #69909, #18250, #50070, .T. ) ;
#25292=ORIENTED_EDGE ( 'NONE', *, *, #82278, .T. ) ;
#25327=CARTESIAN_POINT ( 'NONE',  ( 0.000000000000000000, -11.00000000000000000, 29.75000000000000355 ) ) ;
#25329=DIRECTION ( 'NONE',  ( 0.000000000000000000, 0.000000000000000000, -1.000000000000000000 ) ) ;
#25330=LINE ( 'NONE', #59552, #86857 ) ;
#25341=CARTESIAN_POINT ( 'NONE',  ( 3.262820512820511443, -11.50000000000000000, 29.75000000000000355 ) ) ;
#25349=AXIS2_PLACEMENT_3D ( 'NONE', #15993, #36702, #64155 ) ;
#25357=VECTOR ( 'NONE', #23021, 1000.000000000000000 ) ;
#25358=CARTESIAN_POINT ( 'NONE',  ( 11.25641025641025550, -7.500000000000000000, 29.75000000000000355 ) ) ;
#25363=ORIENTED_EDGE ( 'NONE', *, *, #63468, .T. ) ;
#25373=EDGE_CURVE ( 'NONE', #83780, #7366, #86092, .T. ) ;
#25375=CARTESIAN_POINT ( 'NONE',  ( -12.22435897435897267, -7.500000000000000000, 29.75000000000000355 ) ) ;
#25378=EDGE_LOOP ( 'NONE', ( #81787, #5739, #20196, #41903 ) ) ;
#25400=EDGE_LOOP ( 'NONE', ( #42207, #36019, #79628, #46086 ) ) ;
#25410=FACE_OUTER_BOUND ( 'NONE', #8747, .T. ) ;
#25417=VECTOR ( 'NONE', #31300, 1000.000000000000000 ) ;
#25421=DIRECTION ( 'NONE',  ( -0.000000000000000000, 1.000000000000000000, -0.000000000000000000 ) ) ;
#25438=CARTESIAN_POINT ( 'NONE',  ( 15.84615384615384670, -7.500000000000000000, 29.75000000000000355 ) ) ;
#25450=VECTOR ( 'NONE', #24557, 1000.000000000000000 ) ;
#25460=CARTESIAN_POINT ( 'NONE',  ( 20.00000000000000000, -4.000000000000000000, 29.75000000000000355 ) ) ;
#25462=VERTEX_POINT ( 'NONE', #10873 ) ;
#25471=VERTEX_POINT ( 'NONE', #79779 ) ;
#25477=CARTESIAN_POINT ( 'NONE',  ( 0.000000000000000000, -11.00000000000000000, 29.75000000000000355 ) ) ;
#25478=VECTOR ( 'NONE', #227, 1000.000000000000000 ) ;
#25482=LINE ( 'NONE', #40335, #70949 ) ;
#25507=DIRECTION ( 'NONE',  ( 0.000000000000000000, 0.000000000000000000, 1.000000000000000000 ) ) ;
#25513=CARTESIAN_POINT ( 'NONE',  ( 17.06410256410256565, -7.500000000000000000, 29.75000000000000355 ) ) ;
#25519=VECTOR ( 'NONE', #77610, 1000.000000000000000 ) ;
#25520=CARTESIAN_POINT ( 'NONE',  ( -3.512820512820513663, -11.00000000000000000, 29.75000000000000355 ) ) ;
#25527=FACE_OUTER_BOUND ( 'NONE', #20914, .T. ) ;
#25543=DIRECTION ( 'NONE',  ( -1.000000000000000000, -0.000000000000000000, -0.000000000000000000 ) ) ;
#25551=CARTESIAN_POINT ( 'NONE',  ( 9.320512820512821150, -4.000000000000000000, 29.65000000000000213 ) ) ;
#25563=DIRECTION ( 'NONE',  ( -1.000000000000000000, -0.000000000000000000, -0.000000000000000000 ) ) ;
#25564=ADVANCED_FACE ( 'NONE', ( #7226 ), #67597, .T. ) ;
#25570=VERTEX_POINT ( 'NONE', #13532 ) ;
#25571=EDGE_CURVE ( 'NONE', #27642, #82422, #47311, .T. ) ;
#25572=VECTOR ( 'NONE', #83459, 1000.000000000000000 ) ;
#25581=AXIS2_PLACEMENT_3D ( 'NONE', #48263, #69431, #27560 ) ;
#25585=DIRECTION ( 'NONE',  ( -0.000000000000000000, 0.000000000000000000, 1.000000000000000000 ) ) ;
#25591=EDGE_CURVE ( 'NONE', #23520, #76927, #12208, .T. ) ;
#25599=DIRECTION ( 'NONE',  ( 0.000000000000000000, 0.000000000000000000, 1.000000000000000000 ) ) ;
#25600=DIRECTION ( 'NONE',  ( 1.000000000000000000, 0.000000000000000000, 0.000000000000000000 ) ) ;
#25602=VECTOR ( 'NONE', #22828, 1000.000000000000000 ) ;
#25604=DIRECTION ( 'NONE',  ( -0.000000000000000000, -1.000000000000000000, -0.000000000000000000 ) ) ;
#25628=LINE ( 'NONE', #39607, #74097 ) ;
#25630=DIRECTION ( 'NONE',  ( -1.000000000000000000, 0.000000000000000000, 0.000000000000000000 ) ) ;
#25635=VECTOR ( 'NONE', #76710, 1000.000000000000000 ) ;
#25639=CARTESIAN_POINT ( 'NONE',  ( 9.320512820512821150, -7.500000000000000000, 29.75000000000000355 ) ) ;
#25640=CARTESIAN_POINT ( 'NONE',  ( -2.544871794871794268, -7.500000000000000000, 29.75000000000000355 ) ) ;
#25650=LINE ( 'NONE', #58524, #3489 ) ;
#25653=VECTOR ( 'NONE', #88784, 1000.000000000000000 ) ;
#25683=CARTESIAN_POINT ( 'NONE',  ( -16.81410256410256565, -3.499999999999999556, 29.75000000000000355 ) ) ;
#25708=VECTOR ( 'NONE', #64270, 1000.000000000000000 ) ;
#25718=LINE ( 'NONE', #20296, #61799 ) ;
#25728=CARTESIAN_POINT ( 'NONE',  ( 7.384615384615385025, -7.500000000000000000, 29.75000000000000355 ) ) ;
#25730=LINE ( 'NONE', #5016, #87893 ) ;
#25783=ORIENTED_EDGE ( 'NONE', *, *, #49926, .F. ) ;
#25791=ADVANCED_FACE ( 'NONE', ( #87334 ), #79226, .T. ) ;
#25795=CARTESIAN_POINT ( 'NONE',  ( -0.3589743589743586982, -4.000000000000000000, 29.75000000000000355 ) ) ;
#25797=EDGE_CURVE ( 'NONE', #21038, #40946, #10319, .T. ) ;
#25807=CYLINDRICAL_SURFACE ( 'NONE', #14762, 4.000000000000000000 ) ;
#25809=CARTESIAN_POINT ( 'NONE',  ( -19.50000000000000000, -3.499999999999999556, 29.75000000000000355 ) ) ;
#25810=ADVANCED_FACE ( 'NONE', ( #25162 ), #39138, .T. ) ;
#25815=ADVANCED_FACE ( 'NONE', ( #80111 ), #65689, .F. ) ;
#25816=ORIENTED_EDGE ( 'NONE', *, *, #31768, .F. ) ;
#25823=VECTOR ( 'NONE', #73679, 1000.000000000000000 ) ;
#25856=EDGE_LOOP ( 'NONE', ( #40346, #13340, #35079, #35557 ) ) ;
#25868=LINE ( 'NONE', #11465, #35315 ) ;
#25872=EDGE_LOOP ( 'NONE', ( #50725, #35743, #53285, #50249 ) ) ;
#25891=AXIS2_PLACEMENT_3D ( 'NONE', #27963, #83360, #56322 ) ;
#25893=AXIS2_PLACEMENT_3D ( 'NONE', #9250, #71368, #51524 ) ;
#25902=AXIS2_PLACEMENT_3D ( 'NONE', #9975, #16732, #79332 ) ;
#25905=ORIENTED_EDGE ( 'NONE', *, *, #4458, .F. ) ;
#25917=EDGE_CURVE ( 'NONE', #74851, #496, #27389, .T. ) ;
#25923=CARTESIAN_POINT ( 'NONE',  ( -19.00000000000000000, -3.499999999999999556, 29.75000000000000355 ) ) ;
#25925=ORIENTED_EDGE ( 'NONE', *, *, #3398, .F. ) ;
#25931=DIRECTION ( 'NONE',  ( 0.000000000000000000, 0.000000000000000000, -1.000000000000000000 ) ) ;
#25934=AXIS2_PLACEMENT_3D ( 'NONE', #89107, #20189, #53512 ) ;
#25941=VECTOR ( 'NONE', #76715, 1000.000000000000000 ) ;
#25945=PLANE ( 'NONE',  #70946 ) ;
#25950=LINE ( 'NONE', #53866, #4165 ) ;
#25957=DIRECTION ( 'NONE',  ( 1.000000000000000000, 0.000000000000000000, 0.000000000000000000 ) ) ;
#25978=DIRECTION ( 'NONE',  ( -1.000000000000000000, 0.000000000000000000, -0.000000000000000000 ) ) ;
#25999=ORIENTED_EDGE ( 'NONE', *, *, #13358, .F. ) ;
#26015=ORIENTED_EDGE ( 'NONE', *, *, #23328, .F. ) ;
#26016=VECTOR ( 'NONE', #17069, 1000.000000000000000 ) ;
#26033=EDGE_CURVE ( 'NONE', #955, #78324, #68813, .T. ) ;
#26036=DIRECTION ( 'NONE',  ( 0.000000000000000000, -1.000000000000000000, 0.000000000000000000 ) ) ;
#26042=CARTESIAN_POINT ( 'NONE',  ( 0.6089743589743582541, -3.499999999999999556, 29.75000000000000355 ) ) ;
#26047=CARTESIAN_POINT ( 'NONE',  ( 0.000000000000000000, -11.00000000000000000, 29.75000000000000355 ) ) ;
#26048=CARTESIAN_POINT ( 'NONE',  ( 19.00000000000000000, -3.499999999999999556, 29.75000000000000355 ) ) ;
#26050=DIRECTION ( 'NONE',  ( 0.000000000000000000, 0.000000000000000000, -1.000000000000000000 ) ) ;
#26051=CARTESIAN_POINT ( 'NONE',  ( -8.352564102564102200, -7.500000000000000000, 29.75000000000000355 ) ) ;
#26058=DIRECTION ( 'NONE',  ( 1.000000000000000000, 0.000000000000000000, 0.000000000000000000 ) ) ;
#26064=EDGE_LOOP ( 'NONE', ( #83523, #33941, #5602, #1708, #15301 ) ) ;
#26070=PLANE ( 'NONE',  #39988 ) ;
#26073=DIRECTION ( 'NONE',  ( 1.000000000000000000, 0.000000000000000000, 0.000000000000000000 ) ) ;
#26074=FACE_OUTER_BOUND ( 'NONE', #77771, .T. ) ;
#26079=VERTEX_POINT ( 'NONE', #362 ) ;
#26093=CYLINDRICAL_SURFACE ( 'NONE', #52626, 4.000000000000000000 ) ;
#26104=EDGE_CURVE ( 'NONE', #50090, #31043, #50293, .T. ) ;
#26114=DIRECTION ( 'NONE',  ( -0.000000000000000000, 1.000000000000000000, -0.000000000000000000 ) ) ;
#26124=CARTESIAN_POINT ( 'NONE',  ( 3.512820512820510555, -3.499999999999999556, 29.75000000000000355 ) ) ;
#26128=EDGE_CURVE ( 'NONE', #61830, #75640, #15208, .T. ) ;
#26132=CARTESIAN_POINT ( 'NONE',  ( -7.134615384615385025, -11.50000000000000000, 29.75000000000000355 ) ) ;
#26136=ORIENTED_EDGE ( 'NONE', *, *, #25154, .T. ) ;
#26148=VERTEX_POINT ( 'NONE', #9764 ) ;
#26159=CARTESIAN_POINT ( 'NONE',  ( -11.97435897435897267, -3.499999999999999556, 29.75000000000000355 ) ) ;
#26160=ADVANCED_FACE ( 'NONE', ( #37229 ), #3886, .F. ) ;
#26164=VERTEX_POINT ( 'NONE', #11100 ) ;
#26168=AXIS2_PLACEMENT_3D ( 'NONE', #8580, #36057, #63506 ) ;
#26183=SHAPE_DEFINITION_REPRESENTATION ( #20359, #60984 ) ;
#26189=DIRECTION ( 'NONE',  ( 1.000000000000000000, 0.000000000000000000, 0.000000000000000000 ) ) ;
#26194=CARTESIAN_POINT ( 'NONE',  ( 10.03846153846153832, -4.000000000000000000, 29.65000000000000213 ) ) ;
#26205=ORIENTED_EDGE ( 'NONE', *, *, #87714, .T. ) ;
#26208=AXIS2_PLACEMENT_3D ( 'NONE', #77467, #22083, #42808 ) ;
#26227=DIRECTION ( 'NONE',  ( 0.000000000000000000, 0.000000000000000000, -1.000000000000000000 ) ) ;
#26236=VECTOR ( 'NONE', #27302, 1000.000000000000000 ) ;
#26261=CARTESIAN_POINT ( 'NONE',  ( -10.03846153846153832, -3.499999999999999556, 29.75000000000000355 ) ) ;
#26279=CARTESIAN_POINT ( 'NONE',  ( 15.12820512820512953, -3.499999999999999556, 29.75000000000000355 ) ) ;
#26286=DIRECTION ( 'NONE',  ( 1.000000000000000000, 0.000000000000000000, 0.000000000000000000 ) ) ;
#26298=CARTESIAN_POINT ( 'NONE',  ( 5.198717948717946236, -3.499999999999999556, 29.75000000000000355 ) ) ;
#26299=AXIS2_PLACEMENT_3D ( 'NONE', #35176, #15799, #43264 ) ;
#26300=ORIENTED_EDGE ( 'NONE', *, *, #22463, .T. ) ;
#26302=CARTESIAN_POINT ( 'NONE',  ( -4.480769230769230838, -3.499999999999999556, 29.75000000000000355 ) ) ;
#26309=ADVANCED_FACE ( 'NONE', ( #46218 ), #74582, .T. ) ;
#26310=EDGE_CURVE ( 'NONE', #48029, #12230, #12002, .T. ) ;
#26311=DIRECTION ( 'NONE',  ( -1.000000000000000000, -0.000000000000000000, -0.000000000000000000 ) ) ;
#26312=LINE ( 'NONE', #18677, #34872 ) ;
#26323=EDGE_CURVE ( 'NONE', #69118, #87423, #88123, .T. ) ;
#26338=ORIENTED_EDGE ( 'NONE', *, *, #31627, .T. ) ;
#26340=CARTESIAN_POINT ( 'NONE',  ( 20.00000000000000000, -11.50000000000000000, 29.75000000000000355 ) ) ;
#26356=DIRECTION ( 'NONE',  ( -1.000000000000000000, 0.000000000000000000, -0.000000000000000000 ) ) ;
#26364=ORIENTED_EDGE ( 'NONE', *, *, #16220, .T. ) ;
#26374=EDGE_LOOP ( 'NONE', ( #24223, #77328, #3925, #37829, #39560 ) ) ;
#26384=ORIENTED_EDGE ( 'NONE', *, *, #76189, .F. ) ;
#26390=LINE ( 'NONE', #5668, #62506 ) ;
#26391=DIRECTION ( 'NONE',  ( 0.000000000000000000, 0.000000000000000000, -1.000000000000000000 ) ) ;
#26392=VECTOR ( 'NONE', #82329, 1000.000000000000000 ) ;
#26393=DIRECTION ( 'NONE',  ( -0.000000000000000000, 1.000000000000000000, -0.000000000000000000 ) ) ;
#26400=ORIENTED_EDGE ( 'NONE', *, *, #46509, .T. ) ;
#26416=CARTESIAN_POINT ( 'NONE',  ( 16.09615384615384670, -3.499999999999999556, 29.75000000000000355 ) ) ;
#26420=ORIENTED_EDGE ( 'NONE', *, *, #14209, .T. ) ;
#26425=ORIENTED_EDGE ( 'NONE', *, *, #37599, .T. ) ;
#26434=DIRECTION ( 'NONE',  ( 1.000000000000000000, 0.000000000000000000, 0.000000000000000000 ) ) ;
#26436=CARTESIAN_POINT ( 'NONE',  ( 13.19230769230769340, -3.499999999999999556, 29.75000000000000355 ) ) ;
#26438=EDGE_CURVE ( 'NONE', #64311, #39901, #36257, .T. ) ;
#26449=FACE_OUTER_BOUND ( 'NONE', #69433, .T. ) ;
#26460=ORIENTED_EDGE ( 'NONE', *, *, #13978, .F. ) ;
#26463=ORIENTED_EDGE ( 'NONE', *, *, #7400, .F. ) ;
#26465=AXIS2_PLACEMENT_3D ( 'NONE', #24893, #19911, #86625 ) ;
#26472=LINE ( 'NONE', #89075, #72221 ) ;
#26473=ORIENTED_EDGE ( 'NONE', *, *, #64542, .F. ) ;
#26474=EDGE_LOOP ( 'NONE', ( #7067, #17572, #14949, #9407 ) ) ;
#26475=VERTEX_POINT ( 'NONE', #48870 ) ;
#26477=ORIENTED_EDGE ( 'NONE', *, *, #2904, .F. ) ;
#26482=VERTEX_POINT ( 'NONE', #62374 ) ;
#26492=LINE ( 'NONE', #67922, #57504 ) ;
#26498=EDGE_CURVE ( 'NONE', #87793, #26079, #56073, .T. ) ;
#26508=ORIENTED_EDGE ( 'NONE', *, *, #83353, .F. ) ;
#26522=EDGE_CURVE ( 'NONE', #37056, #53391, #42569, .T. ) ;
#26529=VECTOR ( 'NONE', #35097, 1000.000000000000000 ) ;
#26532=DIRECTION ( 'NONE',  ( 0.000000000000000000, 0.000000000000000000, -1.000000000000000000 ) ) ;
#26561=FACE_OUTER_BOUND ( 'NONE', #31819, .T. ) ;
#26562=ORIENTED_EDGE ( 'NONE', *, *, #44846, .T. ) ;
#26571=ORIENTED_EDGE ( 'NONE', *, *, #17276, .F. ) ;
#26584=DIRECTION ( 'NONE',  ( 0.000000000000000000, 0.000000000000000000, -1.000000000000000000 ) ) ;
#26587=CARTESIAN_POINT ( 'NONE',  ( 14.16025641025641235, -11.00000000000000000, 29.75000000000000355 ) ) ;
#26608=ORIENTED_EDGE ( 'NONE', *, *, #79661, .F. ) ;
#26610=AXIS2_PLACEMENT_3D ( 'NONE', #87473, #31620, #26639 ) ;
#26615=LINE ( 'NONE', #53187, #42955 ) ;
#26621=CARTESIAN_POINT ( 'NONE',  ( 1.576923076923075762, -3.499999999999999556, 29.75000000000000355 ) ) ;
#26628=EDGE_CURVE ( 'NONE', #3856, #25471, #59242, .T. ) ;
#26636=CARTESIAN_POINT ( 'NONE',  ( -19.50000000000000000, -3.499999999999999556, 29.75000000000000355 ) ) ;
#26639=DIRECTION ( 'NONE',  ( 0.000000000000000000, 0.000000000000000000, 1.000000000000000000 ) ) ;
#26651=CARTESIAN_POINT ( 'NONE',  ( -19.50000000000000000, -3.499999999999999556, 29.75000000000000355 ) ) ;
#26663=LINE ( 'NONE', #80286, #16073 ) ;
#26686=CARTESIAN_POINT ( 'NONE',  ( 18.03205128205128105, -7.500000000000000000, 33.75000000000000000 ) ) ;
#26695=VERTEX_POINT ( 'NONE', #66382 ) ;
#26702=DIRECTION ( 'NONE',  ( -1.000000000000000000, -0.000000000000000000, -0.000000000000000000 ) ) ;
#26704=ORIENTED_EDGE ( 'NONE', *, *, #1829, .F. ) ;
#26706=VECTOR ( 'NONE', #351, 1000.000000000000000 ) ;
#26711=ORIENTED_EDGE ( 'NONE', *, *, #23816, .F. ) ;
#26725=LINE ( 'NONE', #80804, #20287 ) ;
#26738=AXIS2_PLACEMENT_3D ( 'NONE', #88066, #187, #54670 ) ;
#26750=EDGE_CURVE ( 'NONE', #45168, #46953, #18654, .T. ) ;
#26751=EDGE_CURVE ( 'NONE', #86970, #48041, #57822, .T. ) ;
#26752=DIRECTION ( 'NONE',  ( 1.000000000000000000, 0.000000000000000000, 0.000000000000000000 ) ) ;
#26771=EDGE_CURVE ( 'NONE', #85779, #60579, #49986, .T. ) ;
#26796=CARTESIAN_POINT ( 'NONE',  ( -1.576923076923076872, -3.499999999999999556, 29.75000000000000355 ) ) ;
#26803=EDGE_CURVE ( 'NONE', #53825, #40554, #2672, .T. ) ;
#26827=AXIS2_PLACEMENT_3D ( 'NONE', #69618, #47572, #83145 ) ;
#26837=CARTESIAN_POINT ( 'NONE',  ( 19.50000000000000000, -4.000000000000000000, 29.75000000000000355 ) ) ;
#26843=CYLINDRICAL_SURFACE ( 'NONE', #55917, 4.000000000000000000 ) ;
#26856=ORIENTED_EDGE ( 'NONE', *, *, #62576, .F. ) ;
#26859=CARTESIAN_POINT ( 'NONE',  ( 16.09615384615384670, -3.499999999999999556, 29.75000000000000355 ) ) ;
#26873=DIRECTION ( 'NONE',  ( 1.000000000000000000, 0.000000000000000000, 0.000000000000000000 ) ) ;
#26876=EDGE_CURVE ( 'NONE', #7644, #61382, #70828, .T. ) ;
#26879=VECTOR ( 'NONE', #34059, 1000.000000000000000 ) ;
#26881=ADVANCED_FACE ( 'NONE', ( #72924 ), #58069, .F. ) ;
#26890=ORIENTED_EDGE ( 'NONE', *, *, #25154, .F. ) ;
#26894=EDGE_CURVE ( 'NONE', #64220, #34293, #39160, .T. ) ;
#26897=CARTESIAN_POINT ( 'NONE',  ( 16.81410256410256565, -3.499999999999999556, 29.75000000000000355 ) ) ;
#26917=ORIENTED_EDGE ( 'NONE', *, *, #66680, .F. ) ;
#26922=AXIS2_PLACEMENT_3D ( 'NONE', #66488, #10211, #17410 ) ;
#26927=ORIENTED_EDGE ( 'NONE', *, *, #23002, .F. ) ;
#26942=EDGE_CURVE ( 'NONE', #48246, #85269, #37699, .T. ) ;
#26946=DIRECTION ( 'NONE',  ( 0.000000000000000000, 0.000000000000000000, -1.000000000000000000 ) ) ;
#26947=DIRECTION ( 'NONE',  ( 0.000000000000000000, 0.000000000000000000, -1.000000000000000000 ) ) ;
#26950=CARTESIAN_POINT ( 'NONE',  ( -15.84615384615384670, -7.500000000000000000, 33.75000000000000000 ) ) ;
#26952=VECTOR ( 'NONE', #62970, 1000.000000000000000 ) ;
#26953=FACE_OUTER_BOUND ( 'NONE', #6774, .T. ) ;
#26956=DIRECTION ( 'NONE',  ( -1.000000000000000000, -0.000000000000000000, -0.000000000000000000 ) ) ;
#26970=AXIS2_PLACEMENT_3D ( 'NONE', #64399, #72054, #3593 ) ;
#26972=ORIENTED_EDGE ( 'NONE', *, *, #59941, .F. ) ;
#26981=LINE ( 'NONE', #54436, #35991 ) ;
#26992=DIRECTION ( 'NONE',  ( 1.000000000000000000, 0.000000000000000000, 0.000000000000000000 ) ) ;
#27006=DIRECTION ( 'NONE',  ( -1.000000000000000000, -0.000000000000000000, -0.000000000000000000 ) ) ;
#27008=VECTOR ( 'NONE', #46712, 1000.000000000000000 ) ;
#27026=ORIENTED_EDGE ( 'NONE', *, *, #81198, .F. ) ;
#27028=AXIS2_PLACEMENT_3D ( 'NONE', #55793, #54913, #69321 ) ;
#27038=EDGE_CURVE ( 'NONE', #58148, #38566, #17598, .T. ) ;
#27059=DIRECTION ( 'NONE',  ( -0.000000000000000000, 1.000000000000000000, -0.000000000000000000 ) ) ;
#27063=VECTOR ( 'NONE', #23882, 1000.000000000000000 ) ;
#27068=VERTEX_POINT ( 'NONE', #62070 ) ;
#27069=EDGE_LOOP ( 'NONE', ( #32331, #25783, #73355, #81468 ) ) ;
#27072=DIRECTION ( 'NONE',  ( -0.000000000000000000, 1.000000000000000000, -0.000000000000000000 ) ) ;
#27075=DIRECTION ( 'NONE',  ( -1.000000000000000000, -0.000000000000000000, -0.000000000000000000 ) ) ;
#27077=ORIENTED_EDGE ( 'NONE', *, *, #59451, .T. ) ;
#27104=DIRECTION ( 'NONE',  ( 0.000000000000000000, 0.000000000000000000, 1.000000000000000000 ) ) ;
#27107=DIRECTION ( 'NONE',  ( 1.000000000000000000, 0.000000000000000000, 0.000000000000000000 ) ) ;
#27123=AXIS2_PLACEMENT_3D ( 'NONE', #81303, #39436, #67779 ) ;
#27129=CARTESIAN_POINT ( 'NONE',  ( -17.78205128205128105, -7.500000000000000000, 33.75000000000000000 ) ) ;
#27134=VERTEX_POINT ( 'NONE', #78237 ) ;
#27140=EDGE_CURVE ( 'NONE', #59157, #53967, #64271, .T. ) ;
#27147=EDGE_CURVE ( 'NONE', #22218, #5644, #36812, .T. ) ;
#27157=PLANE ( 'NONE',  #39888 ) ;
#27161=DIRECTION ( 'NONE',  ( 1.000000000000000000, 0.000000000000000000, 0.000000000000000000 ) ) ;
#27171=LINE ( 'NONE', #27615, #325 ) ;
#27172=DIRECTION ( 'NONE',  ( 1.000000000000000000, 0.000000000000000000, 0.000000000000000000 ) ) ;
#27215=CARTESIAN_POINT ( 'NONE',  ( -20.00000000000000000, -7.500000000000000000, 33.75000000000000000 ) ) ;
#27230=ORIENTED_EDGE ( 'NONE', *, *, #23642, .F. ) ;
#27235=VECTOR ( 'NONE', #33078, 1000.000000000000000 ) ;
#27253=CARTESIAN_POINT ( 'NONE',  ( -7.384615384615385025, -3.499999999999999556, 29.75000000000000355 ) ) ;
#27291=AXIS2_PLACEMENT_3D ( 'NONE', #80254, #46011, #33830 ) ;
#27293=DIRECTION ( 'NONE',  ( 0.000000000000000000, 0.000000000000000000, -1.000000000000000000 ) ) ;
#27298=ADVANCED_FACE ( 'NONE', ( #64716 ), #11117, .T. ) ;
#27301=VECTOR ( 'NONE', #3898, 1000.000000000000000 ) ;
#27302=DIRECTION ( 'NONE',  ( -0.000000000000000000, 1.000000000000000000, -0.000000000000000000 ) ) ;
#27312=LINE ( 'NONE', #46693, #10095 ) ;
#27334=EDGE_CURVE ( 'NONE', #19556, #37056, #82246, .T. ) ;
#27341=VERTEX_POINT ( 'NONE', #41259 ) ;
#27344=AXIS2_PLACEMENT_3D ( 'NONE', #26636, #47341, #14003 ) ;
#27366=AXIS2_PLACEMENT_3D ( 'NONE', #26651, #54552, #12249 ) ;
#27381=EDGE_LOOP ( 'NONE', ( #41222, #55946, #3251, #12195 ) ) ;
#27389=LINE ( 'NONE', #26950, #56286 ) ;
#27394=DIRECTION ( 'NONE',  ( 0.000000000000000000, 0.000000000000000000, 1.000000000000000000 ) ) ;
#27395=CYLINDRICAL_SURFACE ( 'NONE', #86468, 4.000000000000000000 ) ;
#27402=DIRECTION ( 'NONE',  ( 0.000000000000000000, 0.000000000000000000, -1.000000000000000000 ) ) ;
#27427=ADVANCED_FACE ( 'NONE', ( #49774 ), #41697, .F. ) ;
#27435=CIRCLE ( 'NONE', #77752, 4.000000000000000000 ) ;
#27437=CARTESIAN_POINT ( 'NONE',  ( 20.00000000000000000, -3.499999999999999556, 28.25000000000000000 ) ) ;
#27446=AXIS2_PLACEMENT_3D ( 'NONE', #73249, #39920, #25507 ) ;
#27448=VERTEX_POINT ( 'NONE', #28631 ) ;
#27450=ADVANCED_FACE ( 'NONE', ( #56095 ), #9253, .T. ) ;
#27464=CARTESIAN_POINT ( 'NONE',  ( -19.50000000000000000, -3.499999999999999556, 29.75000000000000355 ) ) ;
#27481=EDGE_LOOP ( 'NONE', ( #44854, #8560, #2724, #12819 ) ) ;
#27487=CARTESIAN_POINT ( 'NONE',  ( -13.91025641025641058, -3.499999999999999556, 29.75000000000000355 ) ) ;
#27491=DIRECTION ( 'NONE',  ( -1.000000000000000000, -0.000000000000000000, 0.000000000000000000 ) ) ;
#27516=ORIENTED_EDGE ( 'NONE', *, *, #88872, .T. ) ;
#27525=PLANE ( 'NONE',  #30970 ) ;
#27527=DIRECTION ( 'NONE',  ( -1.000000000000000000, -0.000000000000000000, -0.000000000000000000 ) ) ;
#27542=LINE ( 'NONE', #14022, #74867 ) ;
#27549=LINE ( 'NONE', #55022, #14317 ) ;
#27560=DIRECTION ( 'NONE',  ( 0.000000000000000000, 0.000000000000000000, -1.000000000000000000 ) ) ;
#27561=( NAMED_UNIT ( * ) PLANE_ANGLE_UNIT ( ) SI_UNIT ( $, .RADIAN. ) );
#27562=CARTESIAN_POINT ( 'NONE',  ( -19.50000000000000000, -4.000000000000000000, 29.75000000000000355 ) ) ;
#27589=CARTESIAN_POINT ( 'NONE',  ( -19.50000000000000000, -3.499999999999999556, 29.75000000000000355 ) ) ;
#27599=DIRECTION ( 'NONE',  ( -1.000000000000000000, -0.000000000000000000, -0.000000000000000000 ) ) ;
#27615=CARTESIAN_POINT ( 'NONE',  ( -11.00641025641025550, -7.500000000000000000, 33.75000000000000000 ) ) ;
#27620=DIRECTION ( 'NONE',  ( -1.000000000000000000, -0.000000000000000000, -0.000000000000000000 ) ) ;
#27633=CARTESIAN_POINT ( 'NONE',  ( -2.544871794871793824, -11.50000000000000000, 29.75000000000000355 ) ) ;
#27637=LINE ( 'NONE', #34833, #47854 ) ;
#27640=CARTESIAN_POINT ( 'NONE',  ( -19.50000000000000000, -3.499999999999999556, 29.75000000000000355 ) ) ;
#27641=EDGE_LOOP ( 'NONE', ( #13788, #41072, #16172, #23026 ) ) ;
#27642=VERTEX_POINT ( 'NONE', #5152 ) ;
#27653=VECTOR ( 'NONE', #29940, 1000.000000000000000 ) ;
#27657=EDGE_CURVE ( 'NONE', #56816, #66461, #26312, .T. ) ;
#27691=LINE ( 'NONE', #19607, #75824 ) ;
#27696=VERTEX_POINT ( 'NONE', #53328 ) ;
#27714=FACE_OUTER_BOUND ( 'NONE', #20000, .T. ) ;
#27729=PLANE ( 'NONE',  #2662 ) ;
#27736=AXIS2_PLACEMENT_3D ( 'NONE', #78121, #62816, #1583 ) ;
#27739=EDGE_CURVE ( 'NONE', #20476, #29561, #85225, .T. ) ;
#27747=FACE_OUTER_BOUND ( 'NONE', #25378, .T. ) ;
#27752=CARTESIAN_POINT ( 'NONE',  ( 5.198717948717946236, -11.00000000000000000, 29.75000000000000355 ) ) ;
#27765=ORIENTED_EDGE ( 'NONE', *, *, #20809, .F. ) ;
#27778=EDGE_LOOP ( 'NONE', ( #10424, #10876, #34468, #50913 ) ) ;
#27779=EDGE_CURVE ( 'NONE', #31043, #84442, #27637, .T. ) ;
#27784=EDGE_CURVE ( 'NONE', #75345, #16624, #8706, .T. ) ;
#27796=CARTESIAN_POINT ( 'NONE',  ( -19.50000000000000000, -3.499999999999999556, 29.75000000000000355 ) ) ;
#27801=AXIS2_PLACEMENT_3D ( 'NONE', #19720, #6215, #22370 ) ;
#27806=EDGE_CURVE ( 'NONE', #13174, #76927, #56442, .T. ) ;
#27807=ORIENTED_EDGE ( 'NONE', *, *, #1980, .T. ) ;
#27823=DIRECTION ( 'NONE',  ( 0.000000000000000000, 0.000000000000000000, 1.000000000000000000 ) ) ;
#27835=DIRECTION ( 'NONE',  ( -0.000000000000000000, 1.000000000000000000, -0.000000000000000000 ) ) ;
#27849=ORIENTED_EDGE ( 'NONE', *, *, #24545, .F. ) ;
#27851=CARTESIAN_POINT ( 'NONE',  ( -4.230769230769229061, -4.000000000000000000, 29.75000000000000355 ) ) ;
#27864=VECTOR ( 'NONE', #41319, 1000.000000000000000 ) ;
#27881=CARTESIAN_POINT ( 'NONE',  ( -6.166666666666667851, -7.500000000000000000, 29.75000000000000355 ) ) ;
#27887=CARTESIAN_POINT ( 'NONE',  ( -9.320512820512821150, -11.00000000000000000, 29.65000000000000213 ) ) ;
#27904=CIRCLE ( 'NONE', #39433, 4.000000000000000000 ) ;
#27910=ADVANCED_FACE ( 'NONE', ( #23094 ), #70851, .F. ) ;
#27916=EDGE_LOOP ( 'NONE', ( #37990, #17072, #85934, #49521 ) ) ;
#27938=EDGE_CURVE ( 'NONE', #48865, #3633, #9048, .T. ) ;
#27947=DIRECTION ( 'NONE',  ( -0.000000000000000000, 1.000000000000000000, -0.000000000000000000 ) ) ;
#27963=CARTESIAN_POINT ( 'NONE',  ( 20.00000000000000000, -7.500000000000000000, 29.75000000000000355 ) ) ;
#27993=DIRECTION ( 'NONE',  ( 1.000000000000000000, 0.000000000000000000, 0.000000000000000000 ) ) ;
#28002=DIRECTION ( 'NONE',  ( 0.000000000000000000, 0.000000000000000000, 1.000000000000000000 ) ) ;
#28011=PLANE ( 'NONE',  #58383 ) ;
#28019=DIRECTION ( 'NONE',  ( -1.000000000000000000, -0.000000000000000000, -0.000000000000000000 ) ) ;
#28036=ORIENTED_EDGE ( 'NONE', *, *, #2425, .T. ) ;
#28037=ORIENTED_EDGE ( 'NONE', *, *, #75699, .F. ) ;
#28048=EDGE_CURVE ( 'NONE', #12551, #5961, #82045, .T. ) ;
#28053=DIRECTION ( 'NONE',  ( 0.000000000000000000, -1.000000000000000000, 0.000000000000000000 ) ) ;
#28061=VECTOR ( 'NONE', #6345, 1000.000000000000000 ) ;
#28073=LINE ( 'NONE', #75376, #41277 ) ;
#28074=ORIENTED_EDGE ( 'NONE', *, *, #29772, .T. ) ;
#28100=DIRECTION ( 'NONE',  ( -1.000000000000000000, -0.000000000000000000, -0.000000000000000000 ) ) ;
#28106=ORIENTED_EDGE ( 'NONE', *, *, #68461, .F. ) ;
#28119=ADVANCED_FACE ( 'NONE', ( #8153 ), #1386, .F. ) ;
#28124=ORIENTED_EDGE ( 'NONE', *, *, #13715, .T. ) ;
#28134=CYLINDRICAL_SURFACE ( 'NONE', #19137, 4.000000000000000000 ) ;
#28136=EDGE_LOOP ( 'NONE', ( #65212, #43244, #46892, #72328 ) ) ;
#28142=FACE_OUTER_BOUND ( 'NONE', #76742, .T. ) ;
#28147=ORIENTED_EDGE ( 'NONE', *, *, #14110, .T. ) ;
#28176=ORIENTED_EDGE ( 'NONE', *, *, #35171, .T. ) ;
#28178=EDGE_LOOP ( 'NONE', ( #81194, #88098, #61005, #2742 ) ) ;
#28187=DIRECTION ( 'NONE',  ( 0.000000000000000000, 0.000000000000000000, -1.000000000000000000 ) ) ;
#28197=DIRECTION ( 'NONE',  ( 0.000000000000000000, 0.000000000000000000, -1.000000000000000000 ) ) ;
#28204=CIRCLE ( 'NONE', #49804, 4.000000000000000000 ) ;
#28220=ADVANCED_FACE ( 'NONE', ( #69850 ), #14767, .F. ) ;
#28222=CARTESIAN_POINT ( 'NONE',  ( -18.75000000000000000, -11.50000000000000000, 29.75000000000000355 ) ) ;
#28227=CARTESIAN_POINT ( 'NONE',  ( -14.16025641025641058, -3.499999999999999556, 29.75000000000000355 ) ) ;
#28235=ORIENTED_EDGE ( 'NONE', *, *, #52746, .F. ) ;
#28240=CARTESIAN_POINT ( 'NONE',  ( 4.480769230769229061, -3.499999999999999556, 29.75000000000000355 ) ) ;
#28258=CARTESIAN_POINT ( 'NONE',  ( 13.19230769230769340, -3.499999999999999556, 29.75000000000000355 ) ) ;
#28274=CARTESIAN_POINT ( 'NONE',  ( 2.544871794871793824, -4.000000000000000000, 29.75000000000000355 ) ) ;
#28279=FACE_OUTER_BOUND ( 'NONE', #55300, .T. ) ;
#28293=MANIFOLD_SOLID_BREP ( 'Boss-Extrude6', #24219 ) ;
#28302=VECTOR ( 'NONE', #37508, 1000.000000000000000 ) ;
#28308=DIRECTION ( 'NONE',  ( -0.000000000000000000, 1.000000000000000000, -0.000000000000000000 ) ) ;
#28311=FACE_BOUND ( 'NONE', #28932, .T. ) ;
#28317=DIRECTION ( 'NONE',  ( -1.000000000000000000, -0.000000000000000000, -0.000000000000000000 ) ) ;
#28321=CARTESIAN_POINT ( 'NONE',  ( -12.22435897435897267, -7.500000000000000000, 29.75000000000000355 ) ) ;
#28340=DIRECTION ( 'NONE',  ( -0.000000000000000000, 1.000000000000000000, -0.000000000000000000 ) ) ;
#28341=EDGE_LOOP ( 'NONE', ( #9969, #5694, #80227, #60320 ) ) ;
#28352=DIRECTION ( 'NONE',  ( -0.000000000000000000, 0.000000000000000000, 1.000000000000000000 ) ) ;
#28356=ORIENTED_EDGE ( 'NONE', *, *, #33763, .F. ) ;
#28361=VECTOR ( 'NONE', #52388, 1000.000000000000000 ) ;
#28382=LINE ( 'NONE', #35593, #44702 ) ;
#28384=CARTESIAN_POINT ( 'NONE',  ( 6.416666666666664298, -3.499999999999999556, 29.75000000000000355 ) ) ;
#28389=VERTEX_POINT ( 'NONE', #66939 ) ;
#28391=ORIENTED_EDGE ( 'NONE', *, *, #14209, .F. ) ;
#28406=ORIENTED_EDGE ( 'NONE', *, *, #73070, .T. ) ;
#28407=CARTESIAN_POINT ( 'NONE',  ( -5.198717948717948012, -7.500000000000000000, 29.75000000000000355 ) ) ;
#28419=ORIENTED_EDGE ( 'NONE', *, *, #87760, .T. ) ;
#28421=ADVANCED_FACE ( 'NONE', ( #31830 ), #25945, .F. ) ;
#28422=LINE ( 'NONE', #77058, #2852 ) ;
#28430=DIRECTION ( 'NONE',  ( -0.000000000000000000, 1.000000000000000000, -0.000000000000000000 ) ) ;
#28440=VECTOR ( 'NONE', #18851, 1000.000000000000000 ) ;
#28452=ADVANCED_FACE ( 'NONE', ( #27714 ), #44875, .F. ) ;
#28455=CARTESIAN_POINT ( 'NONE',  ( 20.00000000000000000, -11.00000000000000000, 28.25000000000000000 ) ) ;
#28464=DIRECTION ( 'NONE',  ( 0.000000000000000000, 1.000000000000000000, 0.000000000000000000 ) ) ;
#28467=EDGE_LOOP ( 'NONE', ( #12340, #36058, #35583, #65272 ) ) ;
#28468=AXIS2_PLACEMENT_3D ( 'NONE', #9632, #24923, #58259 ) ;
#28469=EDGE_LOOP ( 'NONE', ( #76073, #52887, #40256, #64534 ) ) ;
#28478=EDGE_CURVE ( 'NONE', #42959, #87881, #88562, .T. ) ;
#28485=ORIENTED_EDGE ( 'NONE', *, *, #393, .F. ) ;
#28503=CARTESIAN_POINT ( 'NONE',  ( 15.12820512820512953, -11.50000000000000000, 29.75000000000000355 ) ) ;
#28530=DIRECTION ( 'NONE',  ( -0.000000000000000000, 1.000000000000000000, -0.000000000000000000 ) ) ;
#28538=ORIENTED_EDGE ( 'NONE', *, *, #64257, .T. ) ;
#28545=VECTOR ( 'NONE', #86861, 1000.000000000000000 ) ;
#28553=EDGE_CURVE ( 'NONE', #78547, #15822, #3296, .T. ) ;
#28569=ADVANCED_FACE ( 'NONE', ( #16424 ), #43011, .F. ) ;
#28576=CARTESIAN_POINT ( 'NONE',  ( 17.78205128205128105, -7.500000000000000000, 29.75000000000000355 ) ) ;
#28582=ORIENTED_EDGE ( 'NONE', *, *, #27147, .F. ) ;
#28614=DIRECTION ( 'NONE',  ( 0.000000000000000000, 0.000000000000000000, -1.000000000000000000 ) ) ;
#28615=CARTESIAN_POINT ( 'NONE',  ( -12.94230769230769162, -7.500000000000000000, 29.75000000000000355 ) ) ;
#28624=FACE_OUTER_BOUND ( 'NONE', #57462, .T. ) ;
#28631=CARTESIAN_POINT ( 'NONE',  ( 8.352564102564102200, -3.499999999999999556, 29.75000000000000355 ) ) ;
#28649=DIRECTION ( 'NONE',  ( 1.000000000000000000, 0.000000000000000000, 0.000000000000000000 ) ) ;
#28655=EDGE_CURVE ( 'NONE', #27642, #26164, #33543, .T. ) ;
#28656=CARTESIAN_POINT ( 'NONE',  ( 20.00000000000000000, -4.000000000000000000, 29.75000000000000355 ) ) ;
#28691=EDGE_LOOP ( 'NONE', ( #40318, #46386, #8787, #62171, #75690 ) ) ;
#28699=VERTEX_POINT ( 'NONE', #43452 ) ;
#28700=DIRECTION ( 'NONE',  ( 1.000000000000000000, 0.000000000000000000, 0.000000000000000000 ) ) ;
#28706=ORIENTED_EDGE ( 'NONE', *, *, #21500, .F. ) ;
#28707=LINE ( 'NONE', #62471, #29297 ) ;
#28716=CYLINDRICAL_SURFACE ( 'NONE', #8078, 4.000000000000000000 ) ;
#28721=DIRECTION ( 'NONE',  ( 1.000000000000000000, 0.000000000000000000, 0.000000000000000000 ) ) ;
#28727=EDGE_CURVE ( 'NONE', #83231, #949, #73607, .T. ) ;
#28730=CYLINDRICAL_SURFACE ( 'NONE', #37200, 4.000000000000000000 ) ;
#28744=ORIENTED_EDGE ( 'NONE', *, *, #84632, .T. ) ;
#28747=CARTESIAN_POINT ( 'NONE',  ( 1.326923076923076206, -4.000000000000000000, 29.75000000000000355 ) ) ;
#28750=DIRECTION ( 'NONE',  ( -1.000000000000000000, 0.000000000000000000, -0.000000000000000000 ) ) ;
#28757=CARTESIAN_POINT ( 'NONE',  ( 8.352564102564102200, -7.500000000000000000, 29.75000000000000355 ) ) ;
#28759=FACE_OUTER_BOUND ( 'NONE', #56248, .T. ) ;
#28764=CARTESIAN_POINT ( 'NONE',  ( -3.512820512820513663, -7.500000000000000000, 29.75000000000000355 ) ) ;
#28765=ORIENTED_EDGE ( 'NONE', *, *, #40740, .F. ) ;
#28782=CARTESIAN_POINT ( 'NONE',  ( -4.230769230769230838, -7.500000000000000000, 29.75000000000000355 ) ) ;
#28792=AXIS2_PLACEMENT_3D ( 'NONE', #60179, #25957, #12447 ) ;
#28805=ORIENTED_EDGE ( 'NONE', *, *, #13316, .T. ) ;
#28806=CARTESIAN_POINT ( 'NONE',  ( 11.00641025641025550, -7.500000000000000000, 33.75000000000000000 ) ) ;
#28826=PLANE ( 'NONE',  #31217 ) ;
#28855=ORIENTED_EDGE ( 'NONE', *, *, #64830, .T. ) ;
#28898=EDGE_CURVE ( 'NONE', #70465, #3756, #76587, .T. ) ;
#28932=EDGE_LOOP ( 'NONE', ( #11091, #31645, #299, #18097 ) ) ;
#28938=ORIENTED_EDGE ( 'NONE', *, *, #65778, .T. ) ;
#28943=DIRECTION ( 'NONE',  ( 0.000000000000000000, 0.000000000000000000, -1.000000000000000000 ) ) ;
#28946=ORIENTED_EDGE ( 'NONE', *, *, #29295, .T. ) ;
#28949=DIRECTION ( 'NONE',  ( 0.000000000000000000, 0.000000000000000000, -1.000000000000000000 ) ) ;
#28958=CARTESIAN_POINT ( 'NONE',  ( -14.16025641025641058, -3.499999999999999556, 29.75000000000000355 ) ) ;
#28959=DIRECTION ( 'NONE',  ( 0.000000000000000000, 0.000000000000000000, -1.000000000000000000 ) ) ;
#28965=CARTESIAN_POINT ( 'NONE',  ( 20.00000000000000000, -7.500000000000000000, 29.75000000000000355 ) ) ;
#28974=ORIENTED_EDGE ( 'NONE', *, *, #32130, .F. ) ;
#28977=ORIENTED_EDGE ( 'NONE', *, *, #30551, .T. ) ;
#28986=AXIS2_PLACEMENT_3D ( 'NONE', #65050, #16435, #10573 ) ;
#29014=DIRECTION ( 'NONE',  ( 0.000000000000000000, -1.000000000000000000, 0.000000000000000000 ) ) ;
#29031=DIRECTION ( 'NONE',  ( 1.000000000000000000, 0.000000000000000000, 0.000000000000000000 ) ) ;
#29049=VERTEX_POINT ( 'NONE', #56010 ) ;
#29066=CYLINDRICAL_SURFACE ( 'NONE', #11845, 4.000000000000000000 ) ;
#29072=ORIENTED_EDGE ( 'NONE', *, *, #57744, .T. ) ;
#29078=EDGE_CURVE ( 'NONE', #38958, #42531, #46041, .T. ) ;
#29091=ORIENTED_EDGE ( 'NONE', *, *, #3084, .T. ) ;
#29098=EDGE_LOOP ( 'NONE', ( #88655, #35244, #49215, #1654 ) ) ;
#29106=LINE ( 'NONE', #30419, #32455 ) ;
#29117=LINE ( 'NONE', #8390, #5714 ) ;
#29120=EDGE_CURVE ( 'NONE', #25462, #8541, #25330, .T. ) ;
#29127=EDGE_LOOP ( 'NONE', ( #6668, #28391, #76636, #24239 ) ) ;
#29129=ORIENTED_EDGE ( 'NONE', *, *, #68330, .T. ) ;
#29131=DIRECTION ( 'NONE',  ( 0.000000000000000000, 0.000000000000000000, -1.000000000000000000 ) ) ;
#29134=CARTESIAN_POINT ( 'NONE',  ( 6.123233995736775897E-17, -2.085786437626902856, 29.75000000000000355 ) ) ;
#29139=CIRCLE ( 'NONE', #9007, 4.000000000000000000 ) ;
#29144=CARTESIAN_POINT ( 'NONE',  ( -19.50000000000000000, -3.499999999999999556, 29.75000000000000355 ) ) ;
#29150=ORIENTED_EDGE ( 'NONE', *, *, #36816, .T. ) ;
#29151=ORIENTED_EDGE ( 'NONE', *, *, #5423, .T. ) ;
#29155=CARTESIAN_POINT ( 'NONE',  ( -17.78205128205128105, -11.00000000000000000, 29.75000000000000355 ) ) ;
#29160=EDGE_CURVE ( 'NONE', #37657, #12551, #62323, .T. ) ;
#29162=FACE_OUTER_BOUND ( 'NONE', #9384, .T. ) ;
#29169=AXIS2_PLACEMENT_3D ( 'NONE', #7117, #12990, #20625 ) ;
#29175=CARTESIAN_POINT ( 'NONE',  ( 17.06410256410256565, -4.000000000000000000, 29.75000000000000355 ) ) ;
#29190=CARTESIAN_POINT ( 'NONE',  ( 13.19230769230769340, -7.500000000000000000, 29.75000000000000355 ) ) ;
#29209=DIRECTION ( 'NONE',  ( -1.000000000000000000, 0.000000000000000000, -0.000000000000000000 ) ) ;
#29224=VERTEX_POINT ( 'NONE', #74406 ) ;
#29240=DIRECTION ( 'NONE',  ( -1.000000000000000000, 0.000000000000000000, -0.000000000000000000 ) ) ;
#29255=CARTESIAN_POINT ( 'NONE',  ( -10.03846153846153832, -11.00000000000000000, 28.25000000000000000 ) ) ;
#29265=EDGE_CURVE ( 'NONE', #85537, #45384, #1964, .T. ) ;
#29295=EDGE_CURVE ( 'NONE', #21236, #83780, #68974, .T. ) ;
#29297=VECTOR ( 'NONE', #48974, 1000.000000000000000 ) ;
#29300=ORIENTED_EDGE ( 'NONE', *, *, #68789, .F. ) ;
#29313=DIRECTION ( 'NONE',  ( -1.000000000000000000, -0.000000000000000000, -0.000000000000000000 ) ) ;
#29339=ORIENTED_EDGE ( 'NONE', *, *, #46342, .F. ) ;
#29342=ORIENTED_EDGE ( 'NONE', *, *, #38128, .F. ) ;
#29356=VECTOR ( 'NONE', #3944, 1000.000000000000000 ) ;
#29384=VERTEX_POINT ( 'NONE', #46329 ) ;
#29387=DIRECTION ( 'NONE',  ( -0.000000000000000000, 1.000000000000000000, -0.000000000000000000 ) ) ;
#29399=ORIENTED_EDGE ( 'NONE', *, *, #68044, .F. ) ;
#29414=CARTESIAN_POINT ( 'NONE',  ( 0.3589743589743582541, -7.500000000000000000, 29.75000000000000355 ) ) ;
#29415=ORIENTED_EDGE ( 'NONE', *, *, #33312, .T. ) ;
#29423=FACE_OUTER_BOUND ( 'NONE', #85505, .T. ) ;
#29434=ORIENTED_EDGE ( 'NONE', *, *, #69586, .T. ) ;
#29443=LINE ( 'NONE', #9171, #21866 ) ;
#29447=LINE ( 'NONE', #71736, #29789 ) ;
#29453=CARTESIAN_POINT ( 'NONE',  ( 10.03846153846153832, -11.00000000000000000, 29.25000000000000000 ) ) ;
#29456=CARTESIAN_POINT ( 'NONE',  ( 10.03846153846153832, -7.500000000000000000, 29.75000000000000355 ) ) ;
#29458=EDGE_CURVE ( 'NONE', #47437, #45062, #859, .T. ) ;
#29462=ORIENTED_EDGE ( 'NONE', *, *, #22921, .F. ) ;
#29472=ORIENTED_EDGE ( 'NONE', *, *, #64014, .F. ) ;
#29483=ORIENTED_EDGE ( 'NONE', *, *, #16615, .F. ) ;
#29485=DIRECTION ( 'NONE',  ( -1.000000000000000000, -0.000000000000000000, -0.000000000000000000 ) ) ;
#29500=ORIENTED_EDGE ( 'NONE', *, *, #5385, .T. ) ;
#29507=ADVANCED_FACE ( 'NONE', ( #82404 ), #75621, .F. ) ;
#29525=DIRECTION ( 'NONE',  ( -1.000000000000000000, -0.000000000000000000, -0.000000000000000000 ) ) ;
#29534=CARTESIAN_POINT ( 'NONE',  ( 12.22435897435897267, -7.500000000000000000, 29.75000000000000355 ) ) ;
#29542=VECTOR ( 'NONE', #46886, 1000.000000000000000 ) ;
#29545=DIRECTION ( 'NONE',  ( -0.000000000000000000, 1.000000000000000000, -0.000000000000000000 ) ) ;
#29547=EDGE_CURVE ( 'NONE', #48938, #5501, #9177, .T. ) ;
#29553=LINE ( 'NONE', #50240, #58538 ) ;
#29554=VECTOR ( 'NONE', #24804, 1000.000000000000000 ) ;
#29557=ADVANCED_FACE ( 'NONE', ( #63438 ), #70649, .F. ) ;
#29558=DIRECTION ( 'NONE',  ( 0.000000000000000000, 0.000000000000000000, -1.000000000000000000 ) ) ;
#29561=VERTEX_POINT ( 'NONE', #8951 ) ;
#29580=DIRECTION ( 'NONE',  ( 1.000000000000000000, 0.000000000000000000, 0.000000000000000000 ) ) ;
#29583=EDGE_LOOP ( 'NONE', ( #50383, #45715, #60543, #35150 ) ) ;
#29587=DIRECTION ( 'NONE',  ( 0.000000000000000000, 0.000000000000000000, -1.000000000000000000 ) ) ;
#29589=ORIENTED_EDGE ( 'NONE', *, *, #76670, .F. ) ;
#29591=PLANE ( 'NONE',  #12967 ) ;
#29601=DIRECTION ( 'NONE',  ( 0.000000000000000000, 0.000000000000000000, -1.000000000000000000 ) ) ;
#29613=EDGE_CURVE ( 'NONE', #82495, #81637, #39329, .T. ) ;
#29615=CARTESIAN_POINT ( 'NONE',  ( -3.512820512820514995, -11.50000000000000000, 29.75000000000000355 ) ) ;
#29623=PLANE ( 'NONE',  #71306 ) ;
#29630=VERTEX_POINT ( 'NONE', #37291 ) ;
#29631=DIRECTION ( 'NONE',  ( 1.000000000000000000, 0.000000000000000000, 0.000000000000000000 ) ) ;
#29648=LINE ( 'NONE', #86383, #2421 ) ;
#29653=FACE_OUTER_BOUND ( 'NONE', #32486, .T. ) ;
#29665=DIRECTION ( 'NONE',  ( 0.000000000000000000, 0.000000000000000000, -1.000000000000000000 ) ) ;
#29678=EDGE_CURVE ( 'NONE', #35531, #61773, #17481, .T. ) ;
#29679=CARTESIAN_POINT ( 'NONE',  ( 20.00000000000000000, -4.000000000000000000, 29.75000000000000355 ) ) ;
#29683=ORIENTED_EDGE ( 'NONE', *, *, #55445, .T. ) ;
#29689=ORIENTED_EDGE ( 'NONE', *, *, #57052, .F. ) ;
#29711=DIRECTION ( 'NONE',  ( -0.000000000000000000, 1.000000000000000000, -0.000000000000000000 ) ) ;
#29712=DIRECTION ( 'NONE',  ( 0.000000000000000000, 0.000000000000000000, -1.000000000000000000 ) ) ;
#29724=ORIENTED_EDGE ( 'NONE', *, *, #73427, .T. ) ;
#29761=AXIS2_PLACEMENT_3D ( 'NONE', #52727, #81113, #51827 ) ;
#29772=EDGE_CURVE ( 'NONE', #23619, #42406, #34537, .T. ) ;
#29789=VECTOR ( 'NONE', #56894, 1000.000000000000000 ) ;
#29800=AXIS2_PLACEMENT_3D ( 'NONE', #77405, #36855, #64316 ) ;
#29827=VERTEX_POINT ( 'NONE', #20138 ) ;
#29837=LINE ( 'NONE', #21296, #36265 ) ;
#29860=ORIENTED_EDGE ( 'NONE', *, *, #73380, .F. ) ;
#29864=VERTEX_POINT ( 'NONE', #12499 ) ;
#29878=DIRECTION ( 'NONE',  ( 1.000000000000000000, 0.000000000000000000, 0.000000000000000000 ) ) ;
#29879=CARTESIAN_POINT ( 'NONE',  ( -2.294871794871794712, -3.499999999999999556, 29.75000000000000355 ) ) ;
#29882=LINE ( 'NONE', #57343, #62767 ) ;
#29887=ORIENTED_EDGE ( 'NONE', *, *, #42090, .T. ) ;
#29889=DIRECTION ( 'NONE',  ( 1.000000000000000000, 0.000000000000000000, 0.000000000000000000 ) ) ;
#29892=PLANE ( 'NONE',  #33422 ) ;
#29903=CARTESIAN_POINT ( 'NONE',  ( 11.25641025641025550, -7.500000000000000000, 29.75000000000000355 ) ) ;
#29905=ADVANCED_FACE ( 'NONE', ( #71746 ), #31206, .F. ) ;
#29913=VECTOR ( 'NONE', #64591, 1000.000000000000000 ) ;
#29920=CARTESIAN_POINT ( 'NONE',  ( -20.00000000000000000, -3.499999999999999556, 29.75000000000000355 ) ) ;
#29923=ORIENTED_EDGE ( 'NONE', *, *, #81831, .T. ) ;
#29925=FACE_OUTER_BOUND ( 'NONE', #17150, .T. ) ;
#29929=EDGE_CURVE ( 'NONE', #18944, #34055, #76858, .T. ) ;
#29940=DIRECTION ( 'NONE',  ( -1.000000000000000000, 0.000000000000000000, -0.000000000000000000 ) ) ;
#29951=CARTESIAN_POINT ( 'NONE',  ( 7.384615384615385025, -3.499999999999999556, 29.75000000000000355 ) ) ;
#29967=ORIENTED_EDGE ( 'NONE', *, *, #50921, .T. ) ;
#29985=CIRCLE ( 'NONE', #52917, 0.5000000000000004441 ) ;
#30000=ADVANCED_FACE ( 'NONE', ( #32995 ), #73988, .F. ) ;
#30004=EDGE_CURVE ( 'NONE', #85209, #14132, #79692, .T. ) ;
#30014=VECTOR ( 'NONE', #19480, 1000.000000000000000 ) ;
#30029=CARTESIAN_POINT ( 'NONE',  ( -8.102564102564102200, -7.500000000000000000, 29.75000000000000355 ) ) ;
#30030=EDGE_CURVE ( 'NONE', #20476, #85537, #60459, .T. ) ;
#30046=ORIENTED_EDGE ( 'NONE', *, *, #83855, .T. ) ;
#30049=EDGE_CURVE ( 'NONE', #30362, #61394, #81190, .T. ) ;
#30063=CARTESIAN_POINT ( 'NONE',  ( -10.28846153846153832, -3.499999999999999556, 29.75000000000000355 ) ) ;
#30066=VECTOR ( 'NONE', #45397, 1000.000000000000000 ) ;
#30068=LINE ( 'NONE', #57089, #32587 ) ;
#30095=DIRECTION ( 'NONE',  ( 0.000000000000000000, 0.000000000000000000, -1.000000000000000000 ) ) ;
#30101=DIRECTION ( 'NONE',  ( 0.000000000000000000, 0.000000000000000000, -1.000000000000000000 ) ) ;
#30104=VERTEX_POINT ( 'NONE', #74877 ) ;
#30105=AXIS2_PLACEMENT_3D ( 'NONE', #32483, #87915, #5474 ) ;
#30109=CARTESIAN_POINT ( 'NONE',  ( -19.50000000000000000, -3.499999999999999556, 29.75000000000000355 ) ) ;
#30125=AXIS2_PLACEMENT_3D ( 'NONE', #18780, #74609, #17889 ) ;
#30146=CARTESIAN_POINT ( 'NONE',  ( 6.416666666666664298, -7.500000000000000000, 29.75000000000000355 ) ) ;
#30150=VERTEX_POINT ( 'NONE', #56366 ) ;
#30170=ORIENTED_EDGE ( 'NONE', *, *, #21548, .T. ) ;
#30172=ORIENTED_EDGE ( 'NONE', *, *, #84530, .F. ) ;
#30201=VECTOR ( 'NONE', #60532, 1000.000000000000000 ) ;
#30202=CIRCLE ( 'NONE', #10061, 4.000000000000000000 ) ;
#30205=ORIENTED_EDGE ( 'NONE', *, *, #88647, .F. ) ;
#30210=VECTOR ( 'NONE', #49308, 1000.000000000000000 ) ;
#30214=DIRECTION ( 'NONE',  ( -1.000000000000000000, -0.000000000000000000, -0.000000000000000000 ) ) ;
#30231=ORIENTED_EDGE ( 'NONE', *, *, #4853, .T. ) ;
#30233=VERTEX_POINT ( 'NONE', #3628 ) ;
#30261=AXIS2_PLACEMENT_3D ( 'NONE', #68740, #7036, #34513 ) ;
#30266=FACE_OUTER_BOUND ( 'NONE', #27641, .T. ) ;
#30270=FACE_OUTER_BOUND ( 'NONE', #81143, .T. ) ;
#30271=EDGE_CURVE ( 'NONE', #58140, #5565, #36105, .T. ) ;
#30283=CARTESIAN_POINT ( 'NONE',  ( -3.512820512820513663, -3.499999999999999556, 29.75000000000000355 ) ) ;
#30295=PLANE ( 'NONE',  #33281 ) ;
#30307=CARTESIAN_POINT ( 'NONE',  ( 7.134615384615385025, -7.500000000000000000, 29.75000000000000355 ) ) ;
#30312=VERTEX_POINT ( 'NONE', #30657 ) ;
#30321=VECTOR ( 'NONE', #20309, 1000.000000000000000 ) ;
#30331=EDGE_CURVE ( 'NONE', #55785, #25570, #42521, .T. ) ;
#30333=ORIENTED_EDGE ( 'NONE', *, *, #2867, .F. ) ;
#30342=ORIENTED_EDGE ( 'NONE', *, *, #84991, .F. ) ;
#30346=ORIENTED_EDGE ( 'NONE', *, *, #63023, .T. ) ;
#30357=CARTESIAN_POINT ( 'NONE',  ( 20.00000000000000000, -4.000000000000000000, 29.75000000000000355 ) ) ;
#30361=LINE ( 'NONE', #58713, #1401 ) ;
#30362=VERTEX_POINT ( 'NONE', #58127 ) ;
#30365=LINE ( 'NONE', #31250, #86414 ) ;
#30367=VERTEX_POINT ( 'NONE', #85610 ) ;
#30374=FACE_OUTER_BOUND ( 'NONE', #38280, .T. ) ;
#30378=LINE ( 'NONE', #15098, #27653 ) ;
#30401=ORIENTED_EDGE ( 'NONE', *, *, #2867, .T. ) ;
#30402=EDGE_CURVE ( 'NONE', #19139, #81634, #4977, .T. ) ;
#30410=VERTEX_POINT ( 'NONE', #74323 ) ;
#30411=CYLINDRICAL_SURFACE ( 'NONE', #21095, 4.000000000000000000 ) ;
#30419=CARTESIAN_POINT ( 'NONE',  ( 20.00000000000000000, -4.000000000000000000, 29.75000000000000355 ) ) ;
#30423=CIRCLE ( 'NONE', #43343, 4.000000000000000000 ) ;
#30428=PLANE ( 'NONE',  #1405 ) ;
#30435=LINE ( 'NONE', #16481, #32854 ) ;
#30439=CARTESIAN_POINT ( 'NONE',  ( 12.94230769230769340, -3.499999999999999556, 29.75000000000000355 ) ) ;
#30456=EDGE_CURVE ( 'NONE', #36253, #5298, #32889, .T. ) ;
#30480=ORIENTED_EDGE ( 'NONE', *, *, #25178, .F. ) ;
#30491=ADVANCED_FACE ( 'NONE', ( #34211 ), #21136, .F. ) ;
#30500=AXIS2_PLACEMENT_3D ( 'NONE', #4924, #25630, #18874 ) ;
#30511=AXIS2_PLACEMENT_3D ( 'NONE', #28321, #43170, #63876 ) ;
#30513=DIRECTION ( 'NONE',  ( -0.000000000000000000, 1.000000000000000000, -0.000000000000000000 ) ) ;
#30525=DIRECTION ( 'NONE',  ( 1.000000000000000000, 0.000000000000000000, 0.000000000000000000 ) ) ;
#30537=VECTOR ( 'NONE', #13996, 1000.000000000000000 ) ;
#30538=LINE ( 'NONE', #77403, #30543 ) ;
#30540=CARTESIAN_POINT ( 'NONE',  ( 1.576923076923075762, -7.500000000000000000, 29.75000000000000355 ) ) ;
#30543=VECTOR ( 'NONE', #58009, 1000.000000000000000 ) ;
#30546=EDGE_LOOP ( 'NONE', ( #20254, #32489, #51534, #39278 ) ) ;
#30551=EDGE_CURVE ( 'NONE', #3262, #12929, #61231, .T. ) ;
#30581=CARTESIAN_POINT ( 'NONE',  ( -0.6089743589743589203, -4.000000000000000000, 29.75000000000000355 ) ) ;
#30582=ORIENTED_EDGE ( 'NONE', *, *, #27779, .T. ) ;
#30586=VECTOR ( 'NONE', #29525, 1000.000000000000000 ) ;
#30593=EDGE_CURVE ( 'NONE', #57207, #88166, #30808, .T. ) ;
#30626=DIRECTION ( 'NONE',  ( 1.000000000000000000, 0.000000000000000000, 0.000000000000000000 ) ) ;
#30644=CARTESIAN_POINT ( 'NONE',  ( 2.294871794871793824, -11.50000000000000000, 29.75000000000000355 ) ) ;
#30647=ORIENTED_EDGE ( 'NONE', *, *, #31910, .F. ) ;
#30649=ADVANCED_FACE ( 'NONE', ( #70216 ), #63451, .F. ) ;
#30650=ORIENTED_EDGE ( 'NONE', *, *, #87067, .F. ) ;
#30651=CARTESIAN_POINT ( 'NONE',  ( -14.87820512820512953, -3.499999999999999556, 29.75000000000000355 ) ) ;
#30654=ORIENTED_EDGE ( 'NONE', *, *, #38460, .F. ) ;
#30657=CARTESIAN_POINT ( 'NONE',  ( -2.544871794871793824, -4.000000000000000000, 29.75000000000000355 ) ) ;
#30661=DIRECTION ( 'NONE',  ( -0.000000000000000000, 1.000000000000000000, -0.000000000000000000 ) ) ;
#30663=EDGE_LOOP ( 'NONE', ( #77470, #36534, #76440, #84999 ) ) ;
#30671=EDGE_CURVE ( 'NONE', #34205, #25462, #19325, .T. ) ;
#30680=VECTOR ( 'NONE', #44951, 1000.000000000000000 ) ;
#30682=FACE_OUTER_BOUND ( 'NONE', #31998, .T. ) ;
#30687=VECTOR ( 'NONE', #47858, 1000.000000000000000 ) ;
#30693=ORIENTED_EDGE ( 'NONE', *, *, #87714, .F. ) ;
#30701=ORIENTED_EDGE ( 'NONE', *, *, #25571, .T. ) ;
#30743=LINE ( 'NONE', #52342, #22657 ) ;
#30751=VERTEX_POINT ( 'NONE', #46733 ) ;
#30755=VECTOR ( 'NONE', #67777, 1000.000000000000000 ) ;
#30774=DIRECTION ( 'NONE',  ( 0.000000000000000000, 0.000000000000000000, -1.000000000000000000 ) ) ;
#30795=ORIENTED_EDGE ( 'NONE', *, *, #47807, .F. ) ;
#30808=CIRCLE ( 'NONE', #75440, 4.000000000000000000 ) ;
#30820=LINE ( 'NONE', #45671, #12162 ) ;
#30825=DIRECTION ( 'NONE',  ( 0.000000000000000000, 0.000000000000000000, -1.000000000000000000 ) ) ;
#30853=LINE ( 'NONE', #58324, #59786 ) ;
#30859=ADVANCED_FACE ( 'NONE', ( #5747 ), #81420, .T. ) ;
#30867=CIRCLE ( 'NONE', #42409, 4.000000000000000000 ) ;
#30871=ORIENTED_EDGE ( 'NONE', *, *, #3770, .T. ) ;
#30874=VERTEX_POINT ( 'NONE', #60686 ) ;
#30895=AXIS2_PLACEMENT_3D ( 'NONE', #25640, #53096, #67075 ) ;
#30933=ORIENTED_EDGE ( 'NONE', *, *, #80659, .T. ) ;
#30940=LINE ( 'NONE', #44900, #76104 ) ;
#30961=ORIENTED_EDGE ( 'NONE', *, *, #52688, .T. ) ;
#30968=EDGE_CURVE ( 'NONE', #59060, #45953, #40437, .T. ) ;
#30970=AXIS2_PLACEMENT_3D ( 'NONE', #62191, #61291, #938 ) ;
#30976=ADVANCED_FACE ( 'NONE', ( #67896 ), #21473, .F. ) ;
#30978=VERTEX_POINT ( 'NONE', #6197 ) ;
#30979=ORIENTED_EDGE ( 'NONE', *, *, #20809, .T. ) ;
#30990=EDGE_CURVE ( 'NONE', #40554, #24285, #83639, .T. ) ;
#31000=ORIENTED_EDGE ( 'NONE', *, *, #66414, .F. ) ;
#31004=ORIENTED_EDGE ( 'NONE', *, *, #4011, .F. ) ;
#31019=DIRECTION ( 'NONE',  ( 0.000000000000000000, 0.000000000000000000, 1.000000000000000000 ) ) ;
#31024=VECTOR ( 'NONE', #15685, 1000.000000000000000 ) ;
#31040=ORIENTED_EDGE ( 'NONE', *, *, #46962, .F. ) ;
#31043=VERTEX_POINT ( 'NONE', #14724 ) ;
#31058=CARTESIAN_POINT ( 'NONE',  ( -1.576923076923076428, -11.50000000000000000, 29.75000000000000355 ) ) ;
#31099=ORIENTED_EDGE ( 'NONE', *, *, #2425, .F. ) ;
#31111=EDGE_LOOP ( 'NONE', ( #5791, #44251, #67496, #50808, #70374 ) ) ;
#31123=LINE ( 'NONE', #80219, #78762 ) ;
#31125=ADVANCED_FACE ( 'NONE', ( #16931 ), #4307, .F. ) ;
#31128=VERTEX_POINT ( 'NONE', #59248 ) ;
#31135=CYLINDRICAL_SURFACE ( 'NONE', #83980, 4.000000000000000000 ) ;
#31148=ORIENTED_EDGE ( 'NONE', *, *, #13473, .T. ) ;
#31149=VECTOR ( 'NONE', #47099, 1000.000000000000000 ) ;
#31170=CARTESIAN_POINT ( 'NONE',  ( -12.94230769230769162, -7.500000000000000000, 29.75000000000000355 ) ) ;
#31189=ORIENTED_EDGE ( 'NONE', *, *, #21005, .F. ) ;
#31204=VECTOR ( 'NONE', #41148, 1000.000000000000000 ) ;
#31206=PLANE ( 'NONE',  #78197 ) ;
#31217=AXIS2_PLACEMENT_3D ( 'NONE', #70241, #23805, #14869 ) ;
#31219=EDGE_CURVE ( 'NONE', #70729, #30367, #39885, .T. ) ;
#31224=ORIENTED_EDGE ( 'NONE', *, *, #81031, .F. ) ;
#31226=VERTEX_POINT ( 'NONE', #41204 ) ;
#31228=ORIENTED_EDGE ( 'NONE', *, *, #22729, .F. ) ;
#31230=AXIS2_PLACEMENT_3D ( 'NONE', #10811, #83937, #72058 ) ;
#31234=LINE ( 'NONE', #28240, #3624 ) ;
#31242=ORIENTED_EDGE ( 'NONE', *, *, #41490, .F. ) ;
#31250=CARTESIAN_POINT ( 'NONE',  ( 20.00000000000000000, -4.000000000000000000, 29.75000000000000355 ) ) ;
#31268=ADVANCED_FACE ( 'NONE', ( #88096 ), #81314, .T. ) ;
#31272=ORIENTED_EDGE ( 'NONE', *, *, #52590, .T. ) ;
#31278=ORIENTED_EDGE ( 'NONE', *, *, #49061, .F. ) ;
#31279=DIRECTION ( 'NONE',  ( 0.000000000000000000, 0.000000000000000000, 1.000000000000000000 ) ) ;
#31281=DIRECTION ( 'NONE',  ( 0.000000000000000000, 0.000000000000000000, -1.000000000000000000 ) ) ;
#31300=DIRECTION ( 'NONE',  ( 1.000000000000000000, 0.000000000000000000, 0.000000000000000000 ) ) ;
#31322=DIRECTION ( 'NONE',  ( 0.000000000000000000, 0.000000000000000000, -1.000000000000000000 ) ) ;
#31337=VECTOR ( 'NONE', #11506, 1000.000000000000000 ) ;
#31359=CARTESIAN_POINT ( 'NONE',  ( 11.00641025641025550, -7.500000000000000000, 29.75000000000000355 ) ) ;
#31365=FACE_OUTER_BOUND ( 'NONE', #987, .T. ) ;
#31366=DIRECTION ( 'NONE',  ( 1.000000000000000000, 0.000000000000000000, 0.000000000000000000 ) ) ;
#31380=LINE ( 'NONE', #52529, #37120 ) ;
#31411=DIRECTION ( 'NONE',  ( -0.000000000000000000, 1.000000000000000000, -0.000000000000000000 ) ) ;
#31419=AXIS2_PLACEMENT_3D ( 'NONE', #36704, #83579, #63723 ) ;
#31429=AXIS2_PLACEMENT_3D ( 'NONE', #41091, #82534, #62237 ) ;
#31431=EDGE_LOOP ( 'NONE', ( #54821, #37039, #85287, #24498, #76875 ) ) ;
#31432=AXIS2_PLACEMENT_3D ( 'NONE', #35618, #14005, #35165 ) ;
#31433=LINE ( 'NONE', #87286, #332 ) ;
#31438=ORIENTED_EDGE ( 'NONE', *, *, #31219, .T. ) ;
#31439=ORIENTED_EDGE ( 'NONE', *, *, #5157, .F. ) ;
#31443=CYLINDRICAL_SURFACE ( 'NONE', #34809, 4.000000000000000000 ) ;
#31457=PLANE ( 'NONE',  #86214 ) ;
#31463=ORIENTED_EDGE ( 'NONE', *, *, #3945, .T. ) ;
#31489=CARTESIAN_POINT ( 'NONE',  ( 7.384615384615385025, -3.499999999999999556, 29.75000000000000355 ) ) ;
#31492=DIRECTION ( 'NONE',  ( -0.000000000000000000, 0.000000000000000000, 1.000000000000000000 ) ) ;
#31495=ADVANCED_FACE ( 'NONE', ( #58692 ), #38886, .T. ) ;
#31512=CARTESIAN_POINT ( 'NONE',  ( 5.448717948717947124, -11.50000000000000000, 29.75000000000000355 ) ) ;
#31527=EDGE_CURVE ( 'NONE', #80799, #47713, #14395, .T. ) ;
#31531=DIRECTION ( 'NONE',  ( 1.000000000000000000, 0.000000000000000000, 0.000000000000000000 ) ) ;
#31541=ORIENTED_EDGE ( 'NONE', *, *, #55699, .T. ) ;
#31546=VECTOR ( 'NONE', #26073, 1000.000000000000000 ) ;
#31561=ORIENTED_EDGE ( 'NONE', *, *, #26104, .F. ) ;
#31576=CARTESIAN_POINT ( 'NONE',  ( -11.25641025641025550, -11.50000000000000000, 29.75000000000000355 ) ) ;
#31583=FACE_OUTER_BOUND ( 'NONE', #80866, .T. ) ;
#31595=LINE ( 'NONE', #85217, #74539 ) ;
#31604=CIRCLE ( 'NONE', #28792, 4.000000000000000000 ) ;
#31620=DIRECTION ( 'NONE',  ( -1.000000000000000000, -0.000000000000000000, -0.000000000000000000 ) ) ;
#31623=CARTESIAN_POINT ( 'NONE',  ( 13.91025641025641235, -7.500000000000000000, 29.75000000000000355 ) ) ;
#31627=EDGE_CURVE ( 'NONE', #84168, #66664, #32557, .T. ) ;
#31628=DIRECTION ( 'NONE',  ( 1.000000000000000000, 0.000000000000000000, 0.000000000000000000 ) ) ;
#31639=CARTESIAN_POINT ( 'NONE',  ( 12.22435897435897267, -7.500000000000000000, 29.75000000000000355 ) ) ;
#31645=ORIENTED_EDGE ( 'NONE', *, *, #11739, .T. ) ;
#31651=AXIS2_PLACEMENT_3D ( 'NONE', #74280, #41827, #7147 ) ;
#31680=DIRECTION ( 'NONE',  ( -1.000000000000000000, -0.000000000000000000, -0.000000000000000000 ) ) ;
#31682=CIRCLE ( 'NONE', #57514, 4.000000000000000000 ) ;
#31686=STYLED_ITEM ( 'NONE', ( #53084 ), #923 ) ;
#31699=EDGE_LOOP ( 'NONE', ( #81968, #86507, #60359, #48851 ) ) ;
#31703=CARTESIAN_POINT ( 'NONE',  ( 16.81410256410256565, -11.50000000000000000, 29.75000000000000355 ) ) ;
#31713=VERTEX_POINT ( 'NONE', #1759 ) ;
#31720=PLANE ( 'NONE',  #53483 ) ;
#31732=CARTESIAN_POINT ( 'NONE',  ( 12.22435897435897267, -4.000000000000000000, 29.75000000000000355 ) ) ;
#31744=ORIENTED_EDGE ( 'NONE', *, *, #82783, .T. ) ;
#31762=DIRECTION ( 'NONE',  ( -1.000000000000000000, -0.000000000000000000, 0.000000000000000000 ) ) ;
#31768=EDGE_CURVE ( 'NONE', #26079, #81234, #38653, .T. ) ;
#31775=DIRECTION ( 'NONE',  ( -1.000000000000000000, 0.000000000000000000, -0.000000000000000000 ) ) ;
#31778=ORIENTED_EDGE ( 'NONE', *, *, #50109, .T. ) ;
#31781=EDGE_CURVE ( 'NONE', #20358, #62888, #81053, .T. ) ;
#31788=CARTESIAN_POINT ( 'NONE',  ( 12.94230769230769340, -7.500000000000000000, 29.75000000000000355 ) ) ;
#31798=AXIS2_PLACEMENT_3D ( 'NONE', #23049, #28943, #1892 ) ;
#31807=VECTOR ( 'NONE', #10557, 1000.000000000000000 ) ;
#31812=CARTESIAN_POINT ( 'NONE',  ( -19.00000000000000000, -3.499999999999999556, 29.75000000000000355 ) ) ;
#31818=CARTESIAN_POINT ( 'NONE',  ( 12.22435897435897267, -3.499999999999999556, 29.75000000000000355 ) ) ;
#31819=EDGE_LOOP ( 'NONE', ( #45488, #22065, #55050, #33395 ) ) ;
#31820=ADVANCED_FACE ( 'NONE', ( #38204 ), #65663, .F. ) ;
#31830=FACE_OUTER_BOUND ( 'NONE', #9666, .T. ) ;
#31844=DIRECTION ( 'NONE',  ( 0.000000000000000000, 0.000000000000000000, -1.000000000000000000 ) ) ;
#31879=CARTESIAN_POINT ( 'NONE',  ( -9.070512820512819374, -3.499999999999999556, 29.75000000000000355 ) ) ;
#31897=VECTOR ( 'NONE', #79889, 1000.000000000000000 ) ;
#31903=ORIENTED_EDGE ( 'NONE', *, *, #10581, .T. ) ;
#31904=PLANE ( 'NONE',  #34366 ) ;
#31909=ORIENTED_EDGE ( 'NONE', *, *, #20273, .T. ) ;
#31910=EDGE_CURVE ( 'NONE', #83780, #4543, #88645, .T. ) ;
#31948=FACE_OUTER_BOUND ( 'NONE', #8946, .T. ) ;
#31964=DIRECTION ( 'NONE',  ( 0.000000000000000000, 0.000000000000000000, 1.000000000000000000 ) ) ;
#31967=CARTESIAN_POINT ( 'NONE',  ( 19.50000000000000000, -11.00000000000000000, 29.75000000000000355 ) ) ;
#31972=VECTOR ( 'NONE', #35873, 1000.000000000000000 ) ;
#31974=DIRECTION ( 'NONE',  ( 0.000000000000000000, 0.000000000000000000, -1.000000000000000000 ) ) ;
#31986=CARTESIAN_POINT ( 'NONE',  ( -5.448717948717948012, -3.499999999999999556, 29.75000000000000355 ) ) ;
#31994=EDGE_LOOP ( 'NONE', ( #82175, #76143, #26015, #57420, #67912 ) ) ;
#31995=DIRECTION ( 'NONE',  ( -1.000000000000000000, -0.000000000000000000, -0.000000000000000000 ) ) ;
#31998=EDGE_LOOP ( 'NONE', ( #85844, #2095, #23032, #74760 ) ) ;
#31999=VECTOR ( 'NONE', #17610, 1000.000000000000000 ) ;
#32008=EDGE_CURVE ( 'NONE', #23542, #71435, #8421, .T. ) ;
#32018=ORIENTED_EDGE ( 'NONE', *, *, #25056, .F. ) ;
#32029=ADVANCED_FACE ( 'NONE', ( #43524 ), #9738, .T. ) ;
#32036=ORIENTED_EDGE ( 'NONE', *, *, #33206, .T. ) ;
#32041=CARTESIAN_POINT ( 'NONE',  ( -19.50000000000000000, -3.499999999999999556, 28.25000000000000000 ) ) ;
#32049=ORIENTED_EDGE ( 'NONE', *, *, #44420, .T. ) ;
#32069=EDGE_CURVE ( 'NONE', #19996, #50277, #85405, .T. ) ;
#32083=LINE ( 'NONE', #66309, #86407 ) ;
#32095=ORIENTED_EDGE ( 'NONE', *, *, #24522, .T. ) ;
#32097=ADVANCED_FACE ( 'NONE', ( #49834 ), #70999, .F. ) ;
#32112=EDGE_LOOP ( 'NONE', ( #13234, #34905, #87638, #62446, #80997 ) ) ;
#32113=PLANE ( 'NONE',  #37131 ) ;
#32123=CIRCLE ( 'NONE', #24718, 4.000000000000000000 ) ;
#32130=EDGE_CURVE ( 'NONE', #66664, #12230, #12410, .T. ) ;
#32139=DIRECTION ( 'NONE',  ( -0.000000000000000000, 0.000000000000000000, 1.000000000000000000 ) ) ;
#32169=CARTESIAN_POINT ( 'NONE',  ( 8.102564102564102200, -7.500000000000000000, 29.75000000000000355 ) ) ;
#32185=EDGE_CURVE ( 'NONE', #32252, #56816, #544, .T. ) ;
#32194=AXIS2_PLACEMENT_3D ( 'NONE', #32568, #32139, #4665 ) ;
#32220=DIRECTION ( 'NONE',  ( -1.000000000000000000, -0.000000000000000000, -0.000000000000000000 ) ) ;
#32233=ORIENTED_EDGE ( 'NONE', *, *, #42090, .F. ) ;
#32234=ORIENTED_EDGE ( 'NONE', *, *, #57936, .T. ) ;
#32252=VERTEX_POINT ( 'NONE', #48846 ) ;
#32253=ADVANCED_FACE ( 'NONE', ( #82656 ), #20492, .F. ) ;
#32259=EDGE_CURVE ( 'NONE', #9873, #58140, #5649, .T. ) ;
#32268=ORIENTED_EDGE ( 'NONE', *, *, #77500, .F. ) ;
#32272=ORIENTED_EDGE ( 'NONE', *, *, #68538, .F. ) ;
#32273=DIRECTION ( 'NONE',  ( -1.000000000000000000, -0.000000000000000000, -0.000000000000000000 ) ) ;
#32280=CARTESIAN_POINT ( 'NONE',  ( 10.28846153846153832, -7.500000000000000000, 33.75000000000000000 ) ) ;
#32283=DIRECTION ( 'NONE',  ( 1.000000000000000000, 0.000000000000000000, 0.000000000000000000 ) ) ;
#32284=DIRECTION ( 'NONE',  ( 1.000000000000000000, 0.000000000000000000, 0.000000000000000000 ) ) ;
#32293=PLANE ( 'NONE',  #15052 ) ;
#32298=CARTESIAN_POINT ( 'NONE',  ( 11.00641025641025550, -4.000000000000000000, 29.75000000000000355 ) ) ;
#32300=LINE ( 'NONE', #32734, #18758 ) ;
#32306=ADVANCED_FACE ( 'NONE', ( #67799 ), #14178, .T. ) ;
#32314=LINE ( 'NONE', #66988, #24565 ) ;
#32317=CARTESIAN_POINT ( 'NONE',  ( 1.576923076923075762, -7.500000000000000000, 29.75000000000000355 ) ) ;
#32327=ORIENTED_EDGE ( 'NONE', *, *, #1517, .F. ) ;
#32330=CARTESIAN_POINT ( 'NONE',  ( 0.000000000000000000, -11.00000000000000000, 29.75000000000000355 ) ) ;
#32331=ORIENTED_EDGE ( 'NONE', *, *, #29678, .F. ) ;
#32333=ORIENTED_EDGE ( 'NONE', *, *, #69647, .T. ) ;
#32334=CARTESIAN_POINT ( 'NONE',  ( 18.75000000000000000, -11.00000000000000000, 29.75000000000000355 ) ) ;
#32339=ORIENTED_EDGE ( 'NONE', *, *, #53299, .T. ) ;
#32354=EDGE_CURVE ( 'NONE', #3876, #70755, #78092, .T. ) ;
#32371=ORIENTED_EDGE ( 'NONE', *, *, #84873, .F. ) ;
#32380=DIRECTION ( 'NONE',  ( -0.000000000000000000, 1.000000000000000000, -0.000000000000000000 ) ) ;
#32388=DIRECTION ( 'NONE',  ( 0.000000000000000000, 0.000000000000000000, 1.000000000000000000 ) ) ;
#32393=ORIENTED_EDGE ( 'NONE', *, *, #73999, .T. ) ;
#32395=EDGE_CURVE ( 'NONE', #3633, #17957, #83540, .T. ) ;
#32422=DIRECTION ( 'NONE',  ( 0.000000000000000000, 0.000000000000000000, 1.000000000000000000 ) ) ;
#32447=ORIENTED_EDGE ( 'NONE', *, *, #77565, .F. ) ;
#32455=VECTOR ( 'NONE', #49363, 1000.000000000000000 ) ;
#32463=DIRECTION ( 'NONE',  ( 1.000000000000000000, 0.000000000000000000, 0.000000000000000000 ) ) ;
#32465=DIRECTION ( 'NONE',  ( 0.000000000000000000, 0.000000000000000000, 1.000000000000000000 ) ) ;
#32468=DIRECTION ( 'NONE',  ( 1.000000000000000000, 0.000000000000000000, 0.000000000000000000 ) ) ;
#32479=VERTEX_POINT ( 'NONE', #24028 ) ;
#32480=VECTOR ( 'NONE', #39228, 1000.000000000000000 ) ;
#32481=CARTESIAN_POINT ( 'NONE',  ( 8.352564102564102200, -3.499999999999999556, 29.75000000000000355 ) ) ;
#32483=CARTESIAN_POINT ( 'NONE',  ( -4.480769230769230838, -7.500000000000000000, 29.75000000000000355 ) ) ;
#32486=EDGE_LOOP ( 'NONE', ( #84970, #25037, #13381, #47161 ) ) ;
#32489=ORIENTED_EDGE ( 'NONE', *, *, #6324, .F. ) ;
#32492=ORIENTED_EDGE ( 'NONE', *, *, #79422, .F. ) ;
#32501=ORIENTED_EDGE ( 'NONE', *, *, #52677, .F. ) ;
#32514=AXIS2_PLACEMENT_3D ( 'NONE', #61640, #56221, #62518 ) ;
#32516=ORIENTED_EDGE ( 'NONE', *, *, #76405, .F. ) ;
#32522=CARTESIAN_POINT ( 'NONE',  ( -17.78205128205128105, -3.499999999999999556, 29.75000000000000355 ) ) ;
#32544=ORIENTED_EDGE ( 'NONE', *, *, #30049, .F. ) ;
#32553=CARTESIAN_POINT ( 'NONE',  ( 11.00641025641025550, -7.500000000000000000, 29.75000000000000355 ) ) ;
#32557=LINE ( 'NONE', #60029, #62318 ) ;
#32568=CARTESIAN_POINT ( 'NONE',  ( 6.416666666666664298, -3.499999999999999556, 29.75000000000000355 ) ) ;
#32571=VERTEX_POINT ( 'NONE', #87096 ) ;
#32579=CARTESIAN_POINT ( 'NONE',  ( -7.134615384615385025, -7.500000000000000000, 33.75000000000000000 ) ) ;
#32586=ORIENTED_EDGE ( 'NONE', *, *, #76801, .F. ) ;
#32587=VECTOR ( 'NONE', #36386, 1000.000000000000000 ) ;
#32593=EDGE_CURVE ( 'NONE', #59060, #83471, #46091, .T. ) ;
#32597=DIRECTION ( 'NONE',  ( 1.000000000000000000, 0.000000000000000000, 0.000000000000000000 ) ) ;
#32613=VECTOR ( 'NONE', #69842, 1000.000000000000000 ) ;
#32622=CIRCLE ( 'NONE', #82966, 4.000000000000000000 ) ;
#32623=PLANE ( 'NONE',  #44736 ) ;
#32643=DIRECTION ( 'NONE',  ( -1.000000000000000000, -0.000000000000000000, 0.000000000000000000 ) ) ;
#32658=ORIENTED_EDGE ( 'NONE', *, *, #27334, .F. ) ;
#32671=PLANE ( 'NONE',  #1393 ) ;
#32673=DIRECTION ( 'NONE',  ( 0.000000000000000000, 0.000000000000000000, -1.000000000000000000 ) ) ;
#32694=CIRCLE ( 'NONE', #26922, 4.000000000000000000 ) ;
#32702=CARTESIAN_POINT ( 'NONE',  ( 6.416666666666664298, -7.500000000000000000, 29.75000000000000355 ) ) ;
#32722=ORIENTED_EDGE ( 'NONE', *, *, #45451, .T. ) ;
#32733=DIRECTION ( 'NONE',  ( 0.000000000000000000, 0.000000000000000000, -1.000000000000000000 ) ) ;
#32734=CARTESIAN_POINT ( 'NONE',  ( -2.294871794871794712, -7.500000000000000000, 33.75000000000000000 ) ) ;
#32751=DIRECTION ( 'NONE',  ( -0.000000000000000000, 1.000000000000000000, -0.000000000000000000 ) ) ;
#32766=ORIENTED_EDGE ( 'NONE', *, *, #52737, .F. ) ;
#32780=ORIENTED_EDGE ( 'NONE', *, *, #39256, .T. ) ;
#32783=LINE ( 'NONE', #12516, #20035 ) ;
#32801=CIRCLE ( 'NONE', #83154, 4.000000000000000000 ) ;
#32819=ORIENTED_EDGE ( 'NONE', *, *, #60581, .F. ) ;
#32824=DIRECTION ( 'NONE',  ( -1.000000000000000000, -0.000000000000000000, -0.000000000000000000 ) ) ;
#32826=CARTESIAN_POINT ( 'NONE',  ( -19.50000000000000000, -3.499999999999999556, 29.75000000000000355 ) ) ;
#32841=DIRECTION ( 'NONE',  ( 0.000000000000000000, 0.000000000000000000, -1.000000000000000000 ) ) ;
#32849=DIRECTION ( 'NONE',  ( -1.000000000000000000, -0.000000000000000000, -0.000000000000000000 ) ) ;
#32854=VECTOR ( 'NONE', #57903, 1000.000000000000000 ) ;
#32889=LINE ( 'NONE', #60353, #43806 ) ;
#32891=ORIENTED_EDGE ( 'NONE', *, *, #72180, .T. ) ;
#32893=VERTEX_POINT ( 'NONE', #6547 ) ;
#32907=VECTOR ( 'NONE', #64834, 1000.000000000000000 ) ;
#32908=CARTESIAN_POINT ( 'NONE',  ( -16.81410256410256565, -7.500000000000000000, 33.75000000000000000 ) ) ;
#32911=EDGE_CURVE ( 'NONE', #6496, #28389, #14182, .T. ) ;
#32925=ORIENTED_EDGE ( 'NONE', *, *, #34052, .T. ) ;
#32927=LINE ( 'NONE', #13979, #80622 ) ;
#32947=LINE ( 'NONE', #41816, #34699 ) ;
#32954=ORIENTED_EDGE ( 'NONE', *, *, #43390, .F. ) ;
#32957=FACE_OUTER_BOUND ( 'NONE', #18052, .T. ) ;
#32967=DIRECTION ( 'NONE',  ( 0.000000000000000000, 0.000000000000000000, 1.000000000000000000 ) ) ;
#32979=EDGE_CURVE ( 'NONE', #2085, #47848, #15518, .T. ) ;
#32986=EDGE_LOOP ( 'NONE', ( #88926, #67700, #18965, #40185 ) ) ;
#32991=LINE ( 'NONE', #27562, #11056 ) ;
#32995=FACE_OUTER_BOUND ( 'NONE', #44746, .T. ) ;
#32998=CARTESIAN_POINT ( 'NONE',  ( 10.03846153846153832, -3.499999999999999556, 29.75000000000000355 ) ) ;
#33015=EDGE_CURVE ( 'NONE', #51776, #11880, #50166, .T. ) ;
#33021=VECTOR ( 'NONE', #76230, 1000.000000000000000 ) ;
#33025=CARTESIAN_POINT ( 'NONE',  ( 20.00000000000000000, -4.000000000000000000, 28.25000000000000000 ) ) ;
#33026=ORIENTED_EDGE ( 'NONE', *, *, #32185, .F. ) ;
#33040=ORIENTED_EDGE ( 'NONE', *, *, #1572, .F. ) ;
#33048=CARTESIAN_POINT ( 'NONE',  ( -3.262820512820514107, -3.499999999999999556, 29.75000000000000355 ) ) ;
#33067=CARTESIAN_POINT ( 'NONE',  ( 11.25641025641025550, -11.50000000000000000, 29.75000000000000355 ) ) ;
#33068=CARTESIAN_POINT ( 'NONE',  ( 5.448717948717947124, -7.500000000000000000, 29.75000000000000355 ) ) ;
#33078=DIRECTION ( 'NONE',  ( -0.000000000000000000, 1.000000000000000000, -0.000000000000000000 ) ) ;
#33089=DIRECTION ( 'NONE',  ( -1.000000000000000000, -0.000000000000000000, 0.000000000000000000 ) ) ;
#33094=LINE ( 'NONE', #4285, #57269 ) ;
#33100=LINE ( 'NONE', #47044, #63623 ) ;
#33144=CIRCLE ( 'NONE', #5834, 4.000000000000000000 ) ;
#33154=FACE_OUTER_BOUND ( 'NONE', #56648, .T. ) ;
#33172=CARTESIAN_POINT ( 'NONE',  ( -5.198717948717948012, -7.500000000000000000, 29.75000000000000355 ) ) ;
#33184=DIRECTION ( 'NONE',  ( -1.000000000000000000, -0.000000000000000000, -0.000000000000000000 ) ) ;
#33188=EDGE_CURVE ( 'NONE', #2843, #67618, #73121, .T. ) ;
#33198=ORIENTED_EDGE ( 'NONE', *, *, #70661, .F. ) ;
#33203=DIRECTION ( 'NONE',  ( -1.000000000000000000, -0.000000000000000000, -0.000000000000000000 ) ) ;
#33206=EDGE_CURVE ( 'NONE', #79365, #14132, #4213, .T. ) ;
#33214=EDGE_LOOP ( 'NONE', ( #23703, #48792, #59917, #81341 ) ) ;
#33239=ORIENTED_EDGE ( 'NONE', *, *, #19058, .F. ) ;
#33241=ORIENTED_EDGE ( 'NONE', *, *, #67812, .T. ) ;
#33244=ORIENTED_EDGE ( 'NONE', *, *, #67861, .F. ) ;
#33271=CARTESIAN_POINT ( 'NONE',  ( 6.416666666666664298, -7.500000000000000000, 29.75000000000000355 ) ) ;
#33281=AXIS2_PLACEMENT_3D ( 'NONE', #23525, #16337, #78468 ) ;
#33312=EDGE_CURVE ( 'NONE', #81634, #19254, #46537, .T. ) ;
#33327=CARTESIAN_POINT ( 'NONE',  ( -1.326923076923076872, -7.500000000000000000, 33.75000000000000000 ) ) ;
#33329=ORIENTED_EDGE ( 'NONE', *, *, #13634, .F. ) ;
#33330=CIRCLE ( 'NONE', #44811, 4.000000000000000000 ) ;
#33339=EDGE_CURVE ( 'NONE', #4576, #58726, #62689, .T. ) ;
#33357=EDGE_CURVE ( 'NONE', #19254, #4576, #21719, .T. ) ;
#33360=DIRECTION ( 'NONE',  ( 1.000000000000000000, 0.000000000000000000, 0.000000000000000000 ) ) ;
#33373=ORIENTED_EDGE ( 'NONE', *, *, #10350, .T. ) ;
#33387=LINE ( 'NONE', #40590, #29542 ) ;
#33388=VECTOR ( 'NONE', #64088, 1000.000000000000000 ) ;
#33393=LINE ( 'NONE', #19868, #30537 ) ;
#33395=ORIENTED_EDGE ( 'NONE', *, *, #17783, .T. ) ;
#33422=AXIS2_PLACEMENT_3D ( 'NONE', #43836, #78503, #58676 ) ;
#33442=ADVANCED_FACE ( 'NONE', ( #37896 ), #59497, .F. ) ;
#33443=VECTOR ( 'NONE', #40385, 1000.000000000000000 ) ;
#33458=ORIENTED_EDGE ( 'NONE', *, *, #87789, .F. ) ;
#33459=FACE_OUTER_BOUND ( 'NONE', #15614, .T. ) ;
#33475=LINE ( 'NONE', #33907, #87706 ) ;
#33498=ORIENTED_EDGE ( 'NONE', *, *, #88741, .T. ) ;
#33500=CARTESIAN_POINT ( 'NONE',  ( 11.25641025641025550, -7.500000000000000000, 33.75000000000000000 ) ) ;
#33524=FACE_OUTER_BOUND ( 'NONE', #88973, .T. ) ;
#33543=CIRCLE ( 'NONE', #76666, 4.000000000000000000 ) ;
#33544=VECTOR ( 'NONE', #54831, 1000.000000000000000 ) ;
#33549=DIRECTION ( 'NONE',  ( -1.000000000000000000, -0.000000000000000000, -0.000000000000000000 ) ) ;
#33556=EDGE_CURVE ( 'NONE', #12929, #58001, #18521, .T. ) ;
#33557=ADVANCED_FACE ( 'NONE', ( #80223 ), #5895, .T. ) ;
#33595=VECTOR ( 'NONE', #70577, 1000.000000000000000 ) ;
#33621=LINE ( 'NONE', #73274, #65678 ) ;
#33633=LINE ( 'NONE', #61532, #16695 ) ;
#33639=CARTESIAN_POINT ( 'NONE',  ( -5.198717948717948012, -11.50000000000000000, 29.75000000000000355 ) ) ;
#33642=LINE ( 'NONE', #6611, #64867 ) ;
#33646=DIRECTION ( 'NONE',  ( -1.000000000000000000, 0.000000000000000000, -0.000000000000000000 ) ) ;
#33664=CIRCLE ( 'NONE', #60983, 4.000000000000000000 ) ;
#33672=ORIENTED_EDGE ( 'NONE', *, *, #23452, .T. ) ;
#33680=PLANE ( 'NONE',  #75263 ) ;
#33684=VECTOR ( 'NONE', #8346, 1000.000000000000000 ) ;
#33697=CARTESIAN_POINT ( 'NONE',  ( 9.320512820512821150, -11.00000000000000000, 28.25000000000000000 ) ) ;
#33725=ORIENTED_EDGE ( 'NONE', *, *, #1970, .T. ) ;
#33742=EDGE_CURVE ( 'NONE', #81743, #5990, #61705, .T. ) ;
#33748=EDGE_CURVE ( 'NONE', #18312, #2392, #54962, .T. ) ;
#33758=VECTOR ( 'NONE', #61523, 1000.000000000000000 ) ;
#33763=EDGE_CURVE ( 'NONE', #52641, #87211, #75669, .T. ) ;
#33780=VERTEX_POINT ( 'NONE', #83776 ) ;
#33783=ORIENTED_EDGE ( 'NONE', *, *, #23229, .F. ) ;
#33799=EDGE_CURVE ( 'NONE', #22240, #19556, #22063, .T. ) ;
#33800=CARTESIAN_POINT ( 'NONE',  ( 13.19230769230769340, -3.499999999999999556, 29.75000000000000355 ) ) ;
#33822=VERTEX_POINT ( 'NONE', #58939 ) ;
#33830=DIRECTION ( 'NONE',  ( 0.000000000000000000, 0.000000000000000000, 1.000000000000000000 ) ) ;
#33865=EDGE_CURVE ( 'NONE', #69118, #18312, #61098, .T. ) ;
#33867=FACE_OUTER_BOUND ( 'NONE', #25872, .T. ) ;
#33893=CIRCLE ( 'NONE', #2256, 4.000000000000000000 ) ;
#33904=AXIS2_PLACEMENT_3D ( 'NONE', #54157, #13193, #20826 ) ;
#33907=CARTESIAN_POINT ( 'NONE',  ( -9.320512820512821150, -1.926643599941765039, 28.25000000000000000 ) ) ;
#33927=DIRECTION ( 'NONE',  ( 0.000000000000000000, 0.000000000000000000, -1.000000000000000000 ) ) ;
#33929=EDGE_LOOP ( 'NONE', ( #38656, #14999, #46881, #34655, #7168 ) ) ;
#33936=VECTOR ( 'NONE', #23225, 1000.000000000000000 ) ;
#33937=EDGE_CURVE ( 'NONE', #28389, #83231, #30867, .T. ) ;
#33941=ORIENTED_EDGE ( 'NONE', *, *, #77262, .T. ) ;
#33943=DIRECTION ( 'NONE',  ( -0.000000000000000000, 1.000000000000000000, -0.000000000000000000 ) ) ;
#33947=DIRECTION ( 'NONE',  ( 1.000000000000000000, 0.000000000000000000, 0.000000000000000000 ) ) ;
#33953=CARTESIAN_POINT ( 'NONE',  ( -3.262820512820514107, -11.00000000000000000, 29.75000000000000355 ) ) ;
#33955=VERTEX_POINT ( 'NONE', #6237 ) ;
#33960=LINE ( 'NONE', #20003, #2725 ) ;
#33965=CYLINDRICAL_SURFACE ( 'NONE', #26738, 4.000000000000000000 ) ;
#33972=EDGE_CURVE ( 'NONE', #80082, #45222, #48099, .T. ) ;
#33992=VECTOR ( 'NONE', #47813, 1000.000000000000000 ) ;
#33996=ORIENTED_EDGE ( 'NONE', *, *, #29547, .T. ) ;
#34006=DIRECTION ( 'NONE',  ( -1.000000000000000000, -0.000000000000000000, -0.000000000000000000 ) ) ;
#34015=DIRECTION ( 'NONE',  ( 1.000000000000000000, 0.000000000000000000, 0.000000000000000000 ) ) ;
#34023=ORIENTED_EDGE ( 'NONE', *, *, #57744, .F. ) ;
#34029=CARTESIAN_POINT ( 'NONE',  ( -2.294871794871794712, -3.499999999999999556, 29.75000000000000355 ) ) ;
#34042=CARTESIAN_POINT ( 'NONE',  ( -13.91025641025641058, -7.500000000000000000, 29.75000000000000355 ) ) ;
#34052=EDGE_CURVE ( 'NONE', #54472, #26695, #62922, .T. ) ;
#34055=VERTEX_POINT ( 'NONE', #29175 ) ;
#34059=DIRECTION ( 'NONE',  ( 1.000000000000000000, 0.000000000000000000, 0.000000000000000000 ) ) ;
#34063=CARTESIAN_POINT ( 'NONE',  ( -12.94230769230769162, -3.499999999999999556, 29.75000000000000355 ) ) ;
#34079=DIRECTION ( 'NONE',  ( -1.000000000000000000, -0.000000000000000000, -0.000000000000000000 ) ) ;
#34091=VECTOR ( 'NONE', #28317, 1000.000000000000000 ) ;
#34097=ORIENTED_EDGE ( 'NONE', *, *, #19160, .F. ) ;
#34128=FACE_OUTER_BOUND ( 'NONE', #31111, .T. ) ;
#34137=CARTESIAN_POINT ( 'NONE',  ( 3.512820512820510555, -3.499999999999999556, 29.75000000000000355 ) ) ;
#34145=FACE_OUTER_BOUND ( 'NONE', #63032, .T. ) ;
#34150=CARTESIAN_POINT ( 'NONE',  ( -18.03205128205128105, -7.500000000000000000, 29.75000000000000355 ) ) ;
#34163=AXIS2_PLACEMENT_3D ( 'NONE', #12258, #39746, #67210 ) ;
#34172=DIRECTION ( 'NONE',  ( 0.000000000000000000, 0.000000000000000000, -1.000000000000000000 ) ) ;
#34192=CARTESIAN_POINT ( 'NONE',  ( -19.50000000000000000, -3.499999999999999556, 29.75000000000000355 ) ) ;
#34201=CARTESIAN_POINT ( 'NONE',  ( 0.000000000000000000, -11.00000000000000000, 29.75000000000000355 ) ) ;
#34205=VERTEX_POINT ( 'NONE', #35469 ) ;
#34211=FACE_OUTER_BOUND ( 'NONE', #41317, .T. ) ;
#34222=CIRCLE ( 'NONE', #75963, 4.000000000000000000 ) ;
#34232=VERTEX_POINT ( 'NONE', #85428 ) ;
#34242=LINE ( 'NONE', #5894, #66106 ) ;
#34255=VERTEX_POINT ( 'NONE', #10217 ) ;
#34264=EDGE_LOOP ( 'NONE', ( #49040, #43510, #22461, #37871 ) ) ;
#34265=VERTEX_POINT ( 'NONE', #3885 ) ;
#34288=ORIENTED_EDGE ( 'NONE', *, *, #28898, .F. ) ;
#34293=VERTEX_POINT ( 'NONE', #41567 ) ;
#34295=FACE_OUTER_BOUND ( 'NONE', #12071, .T. ) ;
#34333=VERTEX_POINT ( 'NONE', #79568 ) ;
#34357=FACE_OUTER_BOUND ( 'NONE', #45428, .T. ) ;
#34365=LINE ( 'NONE', #7353, #10184 ) ;
#34366=AXIS2_PLACEMENT_3D ( 'NONE', #52600, #25585, #47175 ) ;
#34374=CARTESIAN_POINT ( 'NONE',  ( 0.000000000000000000, -11.00000000000000000, 29.25000000000000000 ) ) ;
#34400=ORIENTED_EDGE ( 'NONE', *, *, #37353, .T. ) ;
#34404=PLANE ( 'NONE',  #71190 ) ;
#34410=EDGE_CURVE ( 'NONE', #24943, #87423, #36666, .T. ) ;
#34417=EDGE_CURVE ( 'NONE', #77757, #22218, #22187, .T. ) ;
#34424=LINE ( 'NONE', #26340, #38829 ) ;
#34438=CARTESIAN_POINT ( 'NONE',  ( 10.28846153846153832, -7.500000000000000000, 29.75000000000000355 ) ) ;
#34447=VERTEX_POINT ( 'NONE', #42908 ) ;
#34461=VERTEX_POINT ( 'NONE', #56414 ) ;
#34468=ORIENTED_EDGE ( 'NONE', *, *, #27784, .T. ) ;
#34469=CARTESIAN_POINT ( 'NONE',  ( 2.294871794871793380, -3.499999999999999556, 29.75000000000000355 ) ) ;
#34472=DIRECTION ( 'NONE',  ( -1.000000000000000000, -0.000000000000000000, -0.000000000000000000 ) ) ;
#34497=ORIENTED_EDGE ( 'NONE', *, *, #51470, .T. ) ;
#34501=AXIS2_PLACEMENT_3D ( 'NONE', #3093, #4432, #72890 ) ;
#34504=CARTESIAN_POINT ( 'NONE',  ( -19.50000000000000000, -11.50000000000000000, 29.75000000000000355 ) ) ;
#34510=AXIS2_PLACEMENT_3D ( 'NONE', #12049, #40409, #67866 ) ;
#34512=PLANE ( 'NONE',  #7285 ) ;
#34513=DIRECTION ( 'NONE',  ( 0.000000000000000000, 0.000000000000000000, -1.000000000000000000 ) ) ;
#34531=EDGE_LOOP ( 'NONE', ( #15653, #79342, #14280, #36160 ) ) ;
#34537=LINE ( 'NONE', #26897, #82607 ) ;
#34539=EDGE_LOOP ( 'NONE', ( #10114, #14335, #36857, #70225 ) ) ;
#34546=DIRECTION ( 'NONE',  ( -1.000000000000000000, -0.000000000000000000, -0.000000000000000000 ) ) ;
#34553=EDGE_CURVE ( 'NONE', #21434, #34265, #33387, .T. ) ;
#34556=ORIENTED_EDGE ( 'NONE', *, *, #2680, .F. ) ;
#34567=VECTOR ( 'NONE', #43045, 1000.000000000000000 ) ;
#34568=EDGE_LOOP ( 'NONE', ( #9684, #65939, #48183, #88854 ) ) ;
#34569=ORIENTED_EDGE ( 'NONE', *, *, #47763, .F. ) ;
#34575=EDGE_LOOP ( 'NONE', ( #16696, #4101, #19117, #87411 ) ) ;
#34576=DIRECTION ( 'NONE',  ( 1.000000000000000000, 0.000000000000000000, 0.000000000000000000 ) ) ;
#34646=DIRECTION ( 'NONE',  ( 0.000000000000000000, 0.000000000000000000, -1.000000000000000000 ) ) ;
#34650=ADVANCED_FACE ( 'NONE', ( #47326 ), #68488, .T. ) ;
#34655=ORIENTED_EDGE ( 'NONE', *, *, #68461, .T. ) ;
#34673=VERTEX_POINT ( 'NONE', #69385 ) ;
#34674=AXIS2_PLACEMENT_3D ( 'NONE', #26416, #5254, #18327 ) ;
#34699=VECTOR ( 'NONE', #67176, 1000.000000000000000 ) ;
#34701=DIRECTION ( 'NONE',  ( 0.000000000000000000, 0.000000000000000000, -1.000000000000000000 ) ) ;
#34719=CARTESIAN_POINT ( 'NONE',  ( -0.3589743589743593088, -3.499999999999999556, 29.75000000000000355 ) ) ;
#34728=LINE ( 'NONE', #9037, #18501 ) ;
#34738=EDGE_CURVE ( 'NONE', #58816, #75080, #50419, .T. ) ;
#34741=PLANE ( 'NONE',  #75744 ) ;
#34751=PLANE ( 'NONE',  #88761 ) ;
#34755=DIRECTION ( 'NONE',  ( 1.000000000000000000, 0.000000000000000000, 0.000000000000000000 ) ) ;
#34773=ORIENTED_EDGE ( 'NONE', *, *, #866, .F. ) ;
#34789=ORIENTED_EDGE ( 'NONE', *, *, #69448, .T. ) ;
#34809=AXIS2_PLACEMENT_3D ( 'NONE', #23346, #11172, #57581 ) ;
#34832=DIRECTION ( 'NONE',  ( 0.000000000000000000, 0.000000000000000000, -1.000000000000000000 ) ) ;
#34833=CARTESIAN_POINT ( 'NONE',  ( 14.87820512820512953, -3.499999999999999556, 29.75000000000000355 ) ) ;
#34839=EDGE_LOOP ( 'NONE', ( #13685, #1559, #15568, #69777 ) ) ;
#34848=CARTESIAN_POINT ( 'NONE',  ( -4.480769230769230838, -7.500000000000000000, 29.75000000000000355 ) ) ;
#34870=EDGE_CURVE ( 'NONE', #18944, #44728, #64816, .T. ) ;
#34872=VECTOR ( 'NONE', #66855, 1000.000000000000000 ) ;
#34875=CARTESIAN_POINT ( 'NONE',  ( -19.50000000000000000, -3.499999999999999556, 29.75000000000000355 ) ) ;
#34894=ORIENTED_EDGE ( 'NONE', *, *, #75843, .F. ) ;
#34896=ORIENTED_EDGE ( 'NONE', *, *, #61453, .F. ) ;
#34905=ORIENTED_EDGE ( 'NONE', *, *, #24131, .F. ) ;
#34914=CARTESIAN_POINT ( 'NONE',  ( 0.000000000000000000, -11.00000000000000000, 29.75000000000000355 ) ) ;
#34944=EDGE_CURVE ( 'NONE', #53967, #40946, #44100, .T. ) ;
#34956=ORIENTED_EDGE ( 'NONE', *, *, #75531, .T. ) ;
#34974=ADVANCED_FACE ( 'NONE', ( #31948 ), #40490, .T. ) ;
#34995=EDGE_CURVE ( 'NONE', #28389, #72492, #25628, .T. ) ;
#35014=VERTEX_POINT ( 'NONE', #11681 ) ;
#35020=CYLINDRICAL_SURFACE ( 'NONE', #77688, 4.000000000000000000 ) ;
#35023=DIRECTION ( 'NONE',  ( 1.000000000000000000, 0.000000000000000000, 0.000000000000000000 ) ) ;
#35036=EDGE_CURVE ( 'NONE', #7995, #34447, #13442, .T. ) ;
#35042=CARTESIAN_POINT ( 'NONE',  ( -1.576923076923076872, -3.499999999999999556, 29.75000000000000355 ) ) ;
#35047=DIRECTION ( 'NONE',  ( 0.000000000000000000, 0.000000000000000000, -1.000000000000000000 ) ) ;
#35064=DIRECTION ( 'NONE',  ( -0.000000000000000000, 0.000000000000000000, 1.000000000000000000 ) ) ;
#35079=ORIENTED_EDGE ( 'NONE', *, *, #6944, .T. ) ;
#35082=ORIENTED_EDGE ( 'NONE', *, *, #34944, .T. ) ;
#35084=DIRECTION ( 'NONE',  ( -1.000000000000000000, -0.000000000000000000, -0.000000000000000000 ) ) ;
#35097=DIRECTION ( 'NONE',  ( -1.000000000000000000, -0.000000000000000000, -0.000000000000000000 ) ) ;
#35100=LINE ( 'NONE', #83745, #43499 ) ;
#35112=ADVANCED_FACE ( 'NONE', ( #70602 ), #69276, .F. ) ;
#35114=FACE_OUTER_BOUND ( 'NONE', #85603, .T. ) ;
#35127=VECTOR ( 'NONE', #72193, 1000.000000000000000 ) ;
#35150=ORIENTED_EDGE ( 'NONE', *, *, #39912, .T. ) ;
#35157=CARTESIAN_POINT ( 'NONE',  ( 2.544871794871792936, -7.500000000000000000, 29.75000000000000355 ) ) ;
#35165=DIRECTION ( 'NONE',  ( 0.000000000000000000, 0.000000000000000000, -1.000000000000000000 ) ) ;
#35168=CARTESIAN_POINT ( 'NONE',  ( 13.19230769230769340, -3.499999999999999556, 29.75000000000000355 ) ) ;
#35171=EDGE_CURVE ( 'NONE', #19139, #1878, #10675, .T. ) ;
#35176=CARTESIAN_POINT ( 'NONE',  ( 18.75000000000000000, -7.500000000000000000, 29.75000000000000355 ) ) ;
#35178=EDGE_LOOP ( 'NONE', ( #26473, #69228, #84774, #19094, #85669 ) ) ;
#35191=VECTOR ( 'NONE', #49964, 1000.000000000000000 ) ;
#35197=AXIS2_PLACEMENT_3D ( 'NONE', #4196, #31680, #66347 ) ;
#35213=LINE ( 'NONE', #76651, #30066 ) ;
#35216=ORIENTED_EDGE ( 'NONE', *, *, #6924, .F. ) ;
#35217=VECTOR ( 'NONE', #36619, 1000.000000000000000 ) ;
#35222=ORIENTED_EDGE ( 'NONE', *, *, #86616, .F. ) ;
#35233=ADVANCED_FACE ( 'NONE', ( #64269 ), #29623, .F. ) ;
#35244=ORIENTED_EDGE ( 'NONE', *, *, #62968, .F. ) ;
#35247=ADVANCED_FACE ( 'NONE', ( #16100 ), #51627, .T. ) ;
#35283=VERTEX_POINT ( 'NONE', #25520 ) ;
#35294=CARTESIAN_POINT ( 'NONE',  ( 14.87820512820512953, -11.50000000000000000, 29.75000000000000355 ) ) ;
#35307=DIRECTION ( 'NONE',  ( 1.000000000000000000, 0.000000000000000000, 0.000000000000000000 ) ) ;
#35315=VECTOR ( 'NONE', #24970, 1000.000000000000000 ) ;
#35322=AXIS2_PLACEMENT_3D ( 'NONE', #12979, #60266, #14301 ) ;
#35326=ORIENTED_EDGE ( 'NONE', *, *, #74713, .T. ) ;
#35360=PLANE ( 'NONE',  #2928 ) ;
#35365=EDGE_LOOP ( 'NONE', ( #30172, #73302, #48406, #20677 ) ) ;
#35375=LINE ( 'NONE', #76817, #43930 ) ;
#35377=DIRECTION ( 'NONE',  ( -1.000000000000000000, 0.000000000000000000, -0.000000000000000000 ) ) ;
#35387=ORIENTED_EDGE ( 'NONE', *, *, #49265, .F. ) ;
#35397=CARTESIAN_POINT ( 'NONE',  ( 14.87820512820512953, -11.00000000000000000, 29.75000000000000355 ) ) ;
#35399=DIRECTION ( 'NONE',  ( -0.000000000000000000, 1.000000000000000000, -0.000000000000000000 ) ) ;
#35404=CARTESIAN_POINT ( 'NONE',  ( -0.6089743589743593644, -7.500000000000000000, 29.75000000000000355 ) ) ;
#35409=AXIS2_PLACEMENT_3D ( 'NONE', #38715, #4488, #46360 ) ;
#35436=AXIS2_PLACEMENT_3D ( 'NONE', #62193, #21653, #65174 ) ;
#35448=ORIENTED_EDGE ( 'NONE', *, *, #38128, .T. ) ;
#35449=EDGE_CURVE ( 'NONE', #20712, #86240, #35375, .T. ) ;
#35450=EDGE_LOOP ( 'NONE', ( #18285, #31242, #11471, #12749 ) ) ;
#35452=CARTESIAN_POINT ( 'NONE',  ( -3.262820512820514107, -7.500000000000000000, 29.75000000000000355 ) ) ;
#35462=ORIENTED_EDGE ( 'NONE', *, *, #68716, .F. ) ;
#35465=CARTESIAN_POINT ( 'NONE',  ( -12.94230769230769162, -7.500000000000000000, 29.75000000000000355 ) ) ;
#35466=CARTESIAN_POINT ( 'NONE',  ( -11.00641025641025550, -7.500000000000000000, 29.75000000000000355 ) ) ;
#35469=CARTESIAN_POINT ( 'NONE',  ( 10.28846153846153832, -7.500000000000000000, 33.75000000000000000 ) ) ;
#35480=LINE ( 'NONE', #70597, #19845 ) ;
#35512=VECTOR ( 'NONE', #31995, 1000.000000000000000 ) ;
#35530=AXIS2_PLACEMENT_3D ( 'NONE', #83735, #16146, #15267 ) ;
#35531=VERTEX_POINT ( 'NONE', #36709 ) ;
#35552=VECTOR ( 'NONE', #18670, 1000.000000000000000 ) ;
#35557=ORIENTED_EDGE ( 'NONE', *, *, #6817, .F. ) ;
#35575=VECTOR ( 'NONE', #11078, 1000.000000000000000 ) ;
#35583=ORIENTED_EDGE ( 'NONE', *, *, #17694, .T. ) ;
#35593=CARTESIAN_POINT ( 'NONE',  ( -8.102564102564102200, -3.499999999999999556, 29.75000000000000355 ) ) ;
#35594=ORIENTED_EDGE ( 'NONE', *, *, #77412, .T. ) ;
#35605=AXIS2_PLACEMENT_3D ( 'NONE', #80567, #18850, #86440 ) ;
#35618=CARTESIAN_POINT ( 'NONE',  ( 8.352564102564102200, -7.500000000000000000, 29.75000000000000355 ) ) ;
#35636=CARTESIAN_POINT ( 'NONE',  ( 13.91025641025641235, -3.499999999999999556, 29.75000000000000355 ) ) ;
#35651=EDGE_CURVE ( 'NONE', #54682, #82221, #19114, .T. ) ;
#35657=LINE ( 'NONE', #55036, #17423 ) ;
#35662=FACE_OUTER_BOUND ( 'NONE', #55984, .T. ) ;
#35665=EDGE_CURVE ( 'NONE', #15081, #50717, #25868, .T. ) ;
#35671=LINE ( 'NONE', #85953, #55969 ) ;
#35673=DIRECTION ( 'NONE',  ( -0.000000000000000000, 0.000000000000000000, 1.000000000000000000 ) ) ;
#35678=ORIENTED_EDGE ( 'NONE', *, *, #67022, .F. ) ;
#35687=EDGE_CURVE ( 'NONE', #34255, #21400, #38494, .T. ) ;
#35691=CARTESIAN_POINT ( 'NONE',  ( 20.00000000000000000, -4.000000000000000000, 29.75000000000000355 ) ) ;
#35703=ORIENTED_EDGE ( 'NONE', *, *, #6817, .T. ) ;
#35706=DIRECTION ( 'NONE',  ( 1.000000000000000000, 0.000000000000000000, 0.000000000000000000 ) ) ;
#35710=AXIS2_PLACEMENT_3D ( 'NONE', #18536, #50953, #23497 ) ;
#35711=ORIENTED_EDGE ( 'NONE', *, *, #16155, .T. ) ;
#35718=VECTOR ( 'NONE', #69216, 1000.000000000000000 ) ;
#35724=ORIENTED_EDGE ( 'NONE', *, *, #47807, .T. ) ;
#35739=VERTEX_POINT ( 'NONE', #85189 ) ;
#35743=ORIENTED_EDGE ( 'NONE', *, *, #25275, .F. ) ;
#35748=AXIS2_PLACEMENT_3D ( 'NONE', #30109, #76079, #29240 ) ;
#35754=CIRCLE ( 'NONE', #9876, 4.000000000000000000 ) ;
#35762=ORIENTED_EDGE ( 'NONE', *, *, #50921, .F. ) ;
#35791=DIRECTION ( 'NONE',  ( -1.000000000000000000, -0.000000000000000000, -0.000000000000000000 ) ) ;
#35802=ORIENTED_EDGE ( 'NONE', *, *, #25797, .T. ) ;
#35806=VECTOR ( 'NONE', #45706, 1000.000000000000000 ) ;
#35809=CIRCLE ( 'NONE', #70328, 4.000000000000000000 ) ;
#35818=LINE ( 'NONE', #50189, #47546 ) ;
#35851=LINE ( 'NONE', #63310, #56162 ) ;
#35862=VECTOR ( 'NONE', #65994, 1000.000000000000000 ) ;
#35869=DIRECTION ( 'NONE',  ( -1.000000000000000000, 0.000000000000000000, -0.000000000000000000 ) ) ;
#35873=DIRECTION ( 'NONE',  ( -0.000000000000000000, 1.000000000000000000, -0.000000000000000000 ) ) ;
#35894=CARTESIAN_POINT ( 'NONE',  ( -19.50000000000000000, -11.50000000000000000, 29.75000000000000355 ) ) ;
#35924=FACE_OUTER_BOUND ( 'NONE', #9456, .T. ) ;
#35927=ORIENTED_EDGE ( 'NONE', *, *, #64141, .T. ) ;
#35950=LINE ( 'NONE', #62949, #73021 ) ;
#35967=PRODUCT_DEFINITION ( 'UNKNOWN', '', #72043, #57280 ) ;
#35971=ORIENTED_EDGE ( 'NONE', *, *, #50109, .F. ) ;
#35973=LINE ( 'NONE', #24210, #56938 ) ;
#35981=ORIENTED_EDGE ( 'NONE', *, *, #77434, .F. ) ;
#35986=EDGE_CURVE ( 'NONE', #3292, #345, #11751, .T. ) ;
#35991=VECTOR ( 'NONE', #68399, 1000.000000000000000 ) ;
#35996=ADVANCED_FACE ( 'NONE', ( #16062 ), #75655, .T. ) ;
#35998=AXIS2_PLACEMENT_3D ( 'NONE', #88216, #58926, #3972 ) ;
#36001=EDGE_CURVE ( 'NONE', #27696, #15288, #54950, .T. ) ;
#36019=ORIENTED_EDGE ( 'NONE', *, *, #66122, .T. ) ;
#36026=CYLINDRICAL_SURFACE ( 'NONE', #62941, 4.000000000000000000 ) ;
#36029=DIRECTION ( 'NONE',  ( -0.000000000000000000, 1.000000000000000000, -0.000000000000000000 ) ) ;
#36055=EDGE_LOOP ( 'NONE', ( #35387, #3887, #7126, #47074 ) ) ;
#36057=DIRECTION ( 'NONE',  ( 0.000000000000000000, 0.000000000000000000, -1.000000000000000000 ) ) ;
#36058=ORIENTED_EDGE ( 'NONE', *, *, #26128, .T. ) ;
#36063=AXIS2_PLACEMENT_3D ( 'NONE', #44295, #3778, #10092 ) ;
#36070=DIRECTION ( 'NONE',  ( 1.000000000000000000, 0.000000000000000000, 0.000000000000000000 ) ) ;
#36105=LINE ( 'NONE', #77964, #56671 ) ;
#36107=LINE ( 'NONE', #28455, #16682 ) ;
#36110=ORIENTED_EDGE ( 'NONE', *, *, #33799, .F. ) ;
#36115=EDGE_CURVE ( 'NONE', #72492, #949, #33893, .T. ) ;
#36119=FACE_OUTER_BOUND ( 'NONE', #61582, .T. ) ;
#36135=DIRECTION ( 'NONE',  ( 0.000000000000000000, 0.000000000000000000, -1.000000000000000000 ) ) ;
#36146=LINE ( 'NONE', #75781, #84506 ) ;
#36157=ORIENTED_EDGE ( 'NONE', *, *, #6580, .F. ) ;
#36160=ORIENTED_EDGE ( 'NONE', *, *, #1614, .T. ) ;
#36181=DIRECTION ( 'NONE',  ( -1.000000000000000000, -0.000000000000000000, -0.000000000000000000 ) ) ;
#36184=AXIS2_PLACEMENT_3D ( 'NONE', #58641, #9151, #37481 ) ;
#36191=AXIS2_PLACEMENT_3D ( 'NONE', #50834, #78321, #31019 ) ;
#36201=EDGE_CURVE ( 'NONE', #69909, #58148, #73714, .T. ) ;
#36202=FACE_OUTER_BOUND ( 'NONE', #82256, .T. ) ;
#36223=EDGE_CURVE ( 'NONE', #87922, #52641, #85884, .T. ) ;
#36241=EDGE_CURVE ( 'NONE', #70755, #59129, #46228, .T. ) ;
#36253=VERTEX_POINT ( 'NONE', #72358 ) ;
#36257=LINE ( 'NONE', #22723, #6024 ) ;
#36265=VECTOR ( 'NONE', #57301, 1000.000000000000000 ) ;
#36268=FACE_OUTER_BOUND ( 'NONE', #35450, .T. ) ;
#36283=ORIENTED_EDGE ( 'NONE', *, *, #49314, .T. ) ;
#36323=CARTESIAN_POINT ( 'NONE',  ( 6.416666666666664298, -11.00000000000000000, 29.75000000000000355 ) ) ;
#36342=LINE ( 'NONE', #83204, #104 ) ;
#36345=CARTESIAN_POINT ( 'NONE',  ( -19.50000000000000000, -11.50000000000000000, 29.75000000000000355 ) ) ;
#36358=DIRECTION ( 'NONE',  ( 1.000000000000000000, 0.000000000000000000, 0.000000000000000000 ) ) ;
#36373=CARTESIAN_POINT ( 'NONE',  ( 11.00641025641025550, -3.499999999999999556, 29.75000000000000355 ) ) ;
#36383=ORIENTED_EDGE ( 'NONE', *, *, #83803, .F. ) ;
#36386=DIRECTION ( 'NONE',  ( -1.000000000000000000, -0.000000000000000000, -0.000000000000000000 ) ) ;
#36393=LINE ( 'NONE', #43581, #46108 ) ;
#36434=AXIS2_PLACEMENT_3D ( 'NONE', #46944, #66786, #5087 ) ;
#36445=EDGE_CURVE ( 'NONE', #35739, #69118, #77101, .T. ) ;
#36447=CIRCLE ( 'NONE', #9142, 4.000000000000000000 ) ;
#36456=DIRECTION ( 'NONE',  ( -1.000000000000000000, -0.000000000000000000, 0.000000000000000000 ) ) ;
#36464=LINE ( 'NONE', #9429, #8733 ) ;
#36480=VECTOR ( 'NONE', #76772, 1000.000000000000000 ) ;
#36488=ORIENTED_EDGE ( 'NONE', *, *, #41010, .F. ) ;
#36494=ORIENTED_EDGE ( 'NONE', *, *, #30551, .F. ) ;
#36495=LINE ( 'NONE', #43680, #965 ) ;
#36497=CARTESIAN_POINT ( 'NONE',  ( -13.19230769230769162, -3.499999999999999556, 29.75000000000000355 ) ) ;
#36508=DIRECTION ( 'NONE',  ( -0.000000000000000000, 1.000000000000000000, -0.000000000000000000 ) ) ;
#36526=ORIENTED_EDGE ( 'NONE', *, *, #12586, .T. ) ;
#36534=ORIENTED_EDGE ( 'NONE', *, *, #40988, .F. ) ;
#36536=VERTEX_POINT ( 'NONE', #58747 ) ;
#36548=ORIENTED_EDGE ( 'NONE', *, *, #25178, .T. ) ;
#36552=FACE_OUTER_BOUND ( 'NONE', #11786, .T. ) ;
#36565=ORIENTED_EDGE ( 'NONE', *, *, #15907, .F. ) ;
#36574=ORIENTED_EDGE ( 'NONE', *, *, #61964, .F. ) ;
#36576=VECTOR ( 'NONE', #69155, 1000.000000000000000 ) ;
#36587=EDGE_CURVE ( 'NONE', #47272, #71093, #81256, .T. ) ;
#36591=ORIENTED_EDGE ( 'NONE', *, *, #72421, .F. ) ;
#36593=CARTESIAN_POINT ( 'NONE',  ( -19.50000000000000000, -11.50000000000000000, 29.75000000000000355 ) ) ;
#36604=DIRECTION ( 'NONE',  ( 0.000000000000000000, 0.000000000000000000, -1.000000000000000000 ) ) ;
#36611=AXIS2_PLACEMENT_3D ( 'NONE', #67596, #5005, #19402 ) ;
#36612=DIRECTION ( 'NONE',  ( 0.000000000000000000, 0.000000000000000000, -1.000000000000000000 ) ) ;
#36613=EDGE_CURVE ( 'NONE', #49704, #71861, #19542, .T. ) ;
#36619=DIRECTION ( 'NONE',  ( -0.000000000000000000, 1.000000000000000000, -0.000000000000000000 ) ) ;
#36633=ORIENTED_EDGE ( 'NONE', *, *, #75691, .F. ) ;
#36634=LINE ( 'NONE', #43388, #33388 ) ;
#36635=DIRECTION ( 'NONE',  ( 1.000000000000000000, 0.000000000000000000, 0.000000000000000000 ) ) ;
#36647=VECTOR ( 'NONE', #5816, 1000.000000000000000 ) ;
#36648=FACE_OUTER_BOUND ( 'NONE', #35178, .T. ) ;
#36653=EDGE_CURVE ( 'NONE', #84875, #83291, #67294, .T. ) ;
#36666=CIRCLE ( 'NONE', #72659, 4.000000000000000000 ) ;
#36677=EDGE_CURVE ( 'NONE', #53825, #52479, #40717, .T. ) ;
#36688=ORIENTED_EDGE ( 'NONE', *, *, #36445, .F. ) ;
#36702=DIRECTION ( 'NONE',  ( 1.000000000000000000, 0.000000000000000000, 0.000000000000000000 ) ) ;
#36703=DIRECTION ( 'NONE',  ( -1.000000000000000000, 0.000000000000000000, -0.000000000000000000 ) ) ;
#36704=CARTESIAN_POINT ( 'NONE',  ( 5.448717948717947124, -7.500000000000000000, 29.75000000000000355 ) ) ;
#36709=CARTESIAN_POINT ( 'NONE',  ( -17.78205128205128105, -4.000000000000000000, 29.75000000000000355 ) ) ;
#36733=VECTOR ( 'NONE', #49653, 1000.000000000000000 ) ;
#36743=LINE ( 'NONE', #22777, #33936 ) ;
#36745=FACE_OUTER_BOUND ( 'NONE', #14481, .T. ) ;
#36759=DIRECTION ( 'NONE',  ( -1.000000000000000000, -0.000000000000000000, -0.000000000000000000 ) ) ;
#36768=DIRECTION ( 'NONE',  ( -1.000000000000000000, -0.000000000000000000, -0.000000000000000000 ) ) ;
#36801=CARTESIAN_POINT ( 'NONE',  ( 5.448717948717947124, -11.50000000000000000, 29.75000000000000355 ) ) ;
#36812=LINE ( 'NONE', #35042, #88090 ) ;
#36816=EDGE_CURVE ( 'NONE', #85269, #5298, #16765, .T. ) ;
#36817=ORIENTED_EDGE ( 'NONE', *, *, #36241, .T. ) ;
#36823=DIRECTION ( 'NONE',  ( -1.000000000000000000, -0.000000000000000000, 0.000000000000000000 ) ) ;
#36853=AXIS2_PLACEMENT_3D ( 'NONE', #5036, #60421, #20766 ) ;
#36855=DIRECTION ( 'NONE',  ( 0.000000000000000000, 0.000000000000000000, -1.000000000000000000 ) ) ;
#36857=ORIENTED_EDGE ( 'NONE', *, *, #59364, .F. ) ;
#36874=EDGE_LOOP ( 'NONE', ( #81911, #24507, #85299, #2667 ) ) ;
#36875=AXIS2_PLACEMENT_3D ( 'NONE', #58397, #32284, #31844 ) ;
#36892=DIRECTION ( 'NONE',  ( 0.000000000000000000, 0.000000000000000000, -1.000000000000000000 ) ) ;
#36899=ORIENTED_EDGE ( 'NONE', *, *, #50264, .F. ) ;
#36918=ORIENTED_EDGE ( 'NONE', *, *, #83864, .T. ) ;
#36919=AXIS2_PLACEMENT_3D ( 'NONE', #528, #27993, #23442 ) ;
#36921=CARTESIAN_POINT ( 'NONE',  ( 0.000000000000000000, -4.000000000000000000, 29.25000000000000000 ) ) ;
#36925=LINE ( 'NONE', #77915, #87740 ) ;
#36936=DIRECTION ( 'NONE',  ( 1.000000000000000000, 0.000000000000000000, 0.000000000000000000 ) ) ;
#36953=AXIS2_PLACEMENT_3D ( 'NONE', #66984, #5719, #81833 ) ;
#36958=EDGE_CURVE ( 'NONE', #52415, #1493, #80260, .T. ) ;
#36971=ADVANCED_FACE ( 'NONE', ( #81154 ), #48230, .T. ) ;
#36982=ORIENTED_EDGE ( 'NONE', *, *, #13527, .T. ) ;
#36986=EDGE_CURVE ( 'NONE', #23542, #1333, #80718, .T. ) ;
#36994=AXIS2_PLACEMENT_3D ( 'NONE', #85090, #57607, #15306 ) ;
#36995=ADVANCED_FACE ( 'NONE', ( #32957 ), #20331, .F. ) ;
#37001=DIRECTION ( 'NONE',  ( 0.000000000000000000, 0.000000000000000000, 1.000000000000000000 ) ) ;
#37011=DIRECTION ( 'NONE',  ( -1.000000000000000000, -0.000000000000000000, -0.000000000000000000 ) ) ;
#37012=CARTESIAN_POINT ( 'NONE',  ( 6.166666666666664298, -7.500000000000000000, 29.75000000000000355 ) ) ;
#37015=EDGE_LOOP ( 'NONE', ( #16298, #85581, #231, #18051 ) ) ;
#37025=ORIENTED_EDGE ( 'NONE', *, *, #39848, .T. ) ;
#37029=ORIENTED_EDGE ( 'NONE', *, *, #61153, .F. ) ;
#37039=ORIENTED_EDGE ( 'NONE', *, *, #34870, .F. ) ;
#37042=LINE ( 'NONE', #23099, #35217 ) ;
#37046=CARTESIAN_POINT ( 'NONE',  ( -19.50000000000000000, -3.499999999999999556, 29.75000000000000355 ) ) ;
#37056=VERTEX_POINT ( 'NONE', #41047 ) ;
#37057=CARTESIAN_POINT ( 'NONE',  ( -1.576923076923076872, -7.500000000000000000, 29.75000000000000355 ) ) ;
#37073=CARTESIAN_POINT ( 'NONE',  ( -4.230769230769230838, -3.499999999999999556, 29.75000000000000355 ) ) ;
#37084=EDGE_CURVE ( 'NONE', #53391, #59157, #9795, .T. ) ;
#37102=ADVANCED_FACE ( 'NONE', ( #49572 ), #940, .T. ) ;
#37108=ORIENTED_EDGE ( 'NONE', *, *, #33742, .T. ) ;
#37109=DIRECTION ( 'NONE',  ( -1.000000000000000000, -0.000000000000000000, 0.000000000000000000 ) ) ;
#37114=ADVANCED_FACE ( 'NONE', ( #55879 ), #58409, .F. ) ;
#37120=VECTOR ( 'NONE', #80013, 1000.000000000000000 ) ;
#37131=AXIS2_PLACEMENT_3D ( 'NONE', #52370, #72199, #72647 ) ;
#37135=FACE_OUTER_BOUND ( 'NONE', #5490, .T. ) ;
#37146=DIRECTION ( 'NONE',  ( 1.000000000000000000, 0.000000000000000000, 0.000000000000000000 ) ) ;
#37148=EDGE_LOOP ( 'NONE', ( #26477, #63893, #76861, #3294 ) ) ;
#37184=ORIENTED_EDGE ( 'NONE', *, *, #59065, .T. ) ;
#37185=DIRECTION ( 'NONE',  ( -1.000000000000000000, -0.000000000000000000, -0.000000000000000000 ) ) ;
#37188=EDGE_LOOP ( 'NONE', ( #63640, #68292, #2194, #11074 ) ) ;
#37200=AXIS2_PLACEMENT_3D ( 'NONE', #62059, #56193, #27394 ) ;
#37225=PLANE ( 'NONE',  #84076 ) ;
#37229=FACE_OUTER_BOUND ( 'NONE', #64649, .T. ) ;
#37234=DIRECTION ( 'NONE',  ( 0.000000000000000000, 0.000000000000000000, -1.000000000000000000 ) ) ;
#37238=LINE ( 'NONE', #52087, #42971 ) ;
#37265=DIRECTION ( 'NONE',  ( 1.000000000000000000, 0.000000000000000000, 0.000000000000000000 ) ) ;
#37271=DIRECTION ( 'NONE',  ( -1.000000000000000000, 0.000000000000000000, -0.000000000000000000 ) ) ;
#37281=EDGE_LOOP ( 'NONE', ( #26364, #78753, #37558, #12161 ) ) ;
#37290=ADVANCED_FACE ( 'NONE', ( #27747 ), #54326, .F. ) ;
#37291=CARTESIAN_POINT ( 'NONE',  ( -15.84615384615384670, -11.00000000000000000, 29.75000000000000355 ) ) ;
#37318=CARTESIAN_POINT ( 'NONE',  ( -14.16025641025641058, -11.00000000000000000, 29.75000000000000355 ) ) ;
#37347=CARTESIAN_POINT ( 'NONE',  ( 0.000000000000000000, -11.00000000000000000, 29.75000000000000355 ) ) ;
#37352=ORIENTED_EDGE ( 'NONE', *, *, #5682, .F. ) ;
#37353=EDGE_CURVE ( 'NONE', #71459, #48865, #55654, .T. ) ;
#37363=LINE ( 'NONE', #77043, #7217 ) ;
#37382=VECTOR ( 'NONE', #80471, 1000.000000000000000 ) ;
#37389=VECTOR ( 'NONE', #28308, 1000.000000000000000 ) ;
#37401=VERTEX_POINT ( 'NONE', #43920 ) ;
#37420=AXIS2_PLACEMENT_3D ( 'NONE', #27437, #54904, #88716 ) ;
#37431=DIRECTION ( 'NONE',  ( 0.000000000000000000, 0.000000000000000000, 1.000000000000000000 ) ) ;
#37436=CIRCLE ( 'NONE', #43180, 4.000000000000000000 ) ;
#37449=MECHANICAL_DESIGN_GEOMETRIC_PRESENTATION_REPRESENTATION('',(#31686),#50373);
#37452=DIRECTION ( 'NONE',  ( -0.000000000000000000, 0.000000000000000000, 1.000000000000000000 ) ) ;
#37470=DIRECTION ( 'NONE',  ( -1.000000000000000000, 0.000000000000000000, -0.000000000000000000 ) ) ;
#37474=ORIENTED_EDGE ( 'NONE', *, *, #3834, .T. ) ;
#37481=DIRECTION ( 'NONE',  ( 0.000000000000000000, 0.000000000000000000, 1.000000000000000000 ) ) ;
#37493=LINE ( 'NONE', #64962, #84966 ) ;
#37497=LINE ( 'NONE', #65856, #77299 ) ;
#37502=DIRECTION ( 'NONE',  ( -0.000000000000000000, 1.000000000000000000, -0.000000000000000000 ) ) ;
#37503=ADVANCED_FACE ( 'NONE', ( #50667 ), #30411, .T. ) ;
#37508=DIRECTION ( 'NONE',  ( 1.000000000000000000, 0.000000000000000000, 0.000000000000000000 ) ) ;
#37509=VECTOR ( 'NONE', #58709, 1000.000000000000000 ) ;
#37510=VECTOR ( 'NONE', #77350, 1000.000000000000000 ) ;
#37519=AXIS2_PLACEMENT_3D ( 'NONE', #87125, #32597, #80809 ) ;
#37547=ORIENTED_EDGE ( 'NONE', *, *, #67265, .F. ) ;
#37549=EDGE_CURVE ( 'NONE', #56816, #83848, #59655, .T. ) ;
#37558=ORIENTED_EDGE ( 'NONE', *, *, #88848, .F. ) ;
#37583=DIRECTION ( 'NONE',  ( 1.000000000000000000, 0.000000000000000000, 0.000000000000000000 ) ) ;
#37599=EDGE_CURVE ( 'NONE', #11498, #34673, #38506, .T. ) ;
#37649=FACE_OUTER_BOUND ( 'NONE', #46749, .T. ) ;
#37651=CARTESIAN_POINT ( 'NONE',  ( -19.50000000000000000, -11.50000000000000000, 29.75000000000000355 ) ) ;
#37657=VERTEX_POINT ( 'NONE', #40290 ) ;
#37662=DIRECTION ( 'NONE',  ( -0.000000000000000000, 1.000000000000000000, -0.000000000000000000 ) ) ;
#37665=DIRECTION ( 'NONE',  ( 1.000000000000000000, 0.000000000000000000, 0.000000000000000000 ) ) ;
#37670=VECTOR ( 'NONE', #60110, 1000.000000000000000 ) ;
#37679=CARTESIAN_POINT ( 'NONE',  ( -19.50000000000000000, -3.499999999999999556, 29.75000000000000355 ) ) ;
#37681=DIRECTION ( 'NONE',  ( 1.000000000000000000, 0.000000000000000000, 0.000000000000000000 ) ) ;
#37683=EDGE_CURVE ( 'NONE', #27696, #22240, #2382, .T. ) ;
#37699=CIRCLE ( 'NONE', #30500, 4.000000000000000000 ) ;
#37704=CARTESIAN_POINT ( 'NONE',  ( 0.000000000000000000, -4.000000000000000000, 29.25000000000000000 ) ) ;
#37709=AXIS2_PLACEMENT_3D ( 'NONE', #2070, #70086, #35869 ) ;
#37716=CARTESIAN_POINT ( 'NONE',  ( -16.81410256410256565, -3.499999999999999556, 29.75000000000000355 ) ) ;
#37754=EDGE_LOOP ( 'NONE', ( #28235, #77423, #5656, #36494 ) ) ;
#37798=ORIENTED_EDGE ( 'NONE', *, *, #282, .F. ) ;
#37799=LINE ( 'NONE', #85110, #58779 ) ;
#37804=DIRECTION ( 'NONE',  ( 1.000000000000000000, 0.000000000000000000, 0.000000000000000000 ) ) ;
#37817=ORIENTED_EDGE ( 'NONE', *, *, #47841, .T. ) ;
#37820=EDGE_LOOP ( 'NONE', ( #32501, #68132, #66, #78926, #61814 ) ) ;
#37827=PLANE ( 'NONE',  #48487 ) ;
#37829=ORIENTED_EDGE ( 'NONE', *, *, #67680, .T. ) ;
#37830=CARTESIAN_POINT ( 'NONE',  ( -13.91025641025641058, -7.500000000000000000, 29.75000000000000355 ) ) ;
#37834=VECTOR ( 'NONE', #10558, 1000.000000000000000 ) ;
#37835=EDGE_CURVE ( 'NONE', #48938, #31226, #49252, .T. ) ;
#37843=VECTOR ( 'NONE', #42095, 1000.000000000000000 ) ;
#37853=VERTEX_POINT ( 'NONE', #72168 ) ;
#37854=DIRECTION ( 'NONE',  ( -0.000000000000000000, 1.000000000000000000, -0.000000000000000000 ) ) ;
#37856=EDGE_CURVE ( 'NONE', #36253, #72492, #73521, .T. ) ;
#37862=ORIENTED_EDGE ( 'NONE', *, *, #39053, .F. ) ;
#37871=ORIENTED_EDGE ( 'NONE', *, *, #59448, .T. ) ;
#37881=ORIENTED_EDGE ( 'NONE', *, *, #73070, .F. ) ;
#37896=FACE_OUTER_BOUND ( 'NONE', #40619, .T. ) ;
#37909=DIRECTION ( 'NONE',  ( 1.000000000000000000, 0.000000000000000000, 0.000000000000000000 ) ) ;
#37917=ORIENTED_EDGE ( 'NONE', *, *, #23479, .T. ) ;
#37956=ORIENTED_EDGE ( 'NONE', *, *, #22708, .F. ) ;
#37959=AXIS2_PLACEMENT_3D ( 'NONE', #2092, #29580, #44391 ) ;
#37972=ORIENTED_EDGE ( 'NONE', *, *, #81264, .F. ) ;
#37974=DIRECTION ( 'NONE',  ( 0.000000000000000000, 0.000000000000000000, -1.000000000000000000 ) ) ;
#37985=ADVANCED_FACE ( 'NONE', ( #34295 ), #34741, .T. ) ;
#37988=ORIENTED_EDGE ( 'NONE', *, *, #38274, .T. ) ;
#37989=VECTOR ( 'NONE', #57752, 1000.000000000000000 ) ;
#37990=ORIENTED_EDGE ( 'NONE', *, *, #55597, .F. ) ;
#37991=ORIENTED_EDGE ( 'NONE', *, *, #39848, .F. ) ;
#38012=CARTESIAN_POINT ( 'NONE',  ( 4.230769230769229061, -3.499999999999999556, 29.75000000000000355 ) ) ;
#38076=LINE ( 'NONE', #23228, #88097 ) ;
#38092=DIRECTION ( 'NONE',  ( 0.000000000000000000, 0.000000000000000000, -1.000000000000000000 ) ) ;
#38094=ORIENTED_EDGE ( 'NONE', *, *, #6529, .F. ) ;
#38096=EDGE_CURVE ( 'NONE', #31128, #43735, #41952, .T. ) ;
#38128=EDGE_CURVE ( 'NONE', #3529, #84875, #42717, .T. ) ;
#38132=CARTESIAN_POINT ( 'NONE',  ( -7.384615384615385025, -11.50000000000000000, 29.75000000000000355 ) ) ;
#38140=LINE ( 'NONE', #22411, #71903 ) ;
#38179=CARTESIAN_POINT ( 'NONE',  ( 11.97435897435897267, -7.500000000000000000, 29.75000000000000355 ) ) ;
#38183=ORIENTED_EDGE ( 'NONE', *, *, #30402, .F. ) ;
#38204=FACE_OUTER_BOUND ( 'NONE', #13274, .T. ) ;
#38209=EDGE_CURVE ( 'NONE', #72149, #47713, #83726, .T. ) ;
#38211=ORIENTED_EDGE ( 'NONE', *, *, #36653, .T. ) ;
#38212=ORIENTED_EDGE ( 'NONE', *, *, #35651, .F. ) ;
#38238=ORIENTED_EDGE ( 'NONE', *, *, #14828, .T. ) ;
#38246=DIRECTION ( 'NONE',  ( -0.000000000000000000, 1.000000000000000000, -0.000000000000000000 ) ) ;
#38248=DIRECTION ( 'NONE',  ( 1.000000000000000000, 0.000000000000000000, 0.000000000000000000 ) ) ;
#38252=( NAMED_UNIT ( * ) PLANE_ANGLE_UNIT ( ) SI_UNIT ( $, .RADIAN. ) );
#38262=DIRECTION ( 'NONE',  ( 0.000000000000000000, 0.000000000000000000, 1.000000000000000000 ) ) ;
#38268=VERTEX_POINT ( 'NONE', #31879 ) ;
#38274=EDGE_CURVE ( 'NONE', #70465, #81224, #71496, .T. ) ;
#38280=EDGE_LOOP ( 'NONE', ( #51242, #12670, #66306, #80171 ) ) ;
#38287=EDGE_CURVE ( 'NONE', #79996, #3529, #58496, .T. ) ;
#38288=CARTESIAN_POINT ( 'NONE',  ( -19.50000000000000000, -11.50000000000000000, 29.75000000000000355 ) ) ;
#38303=CARTESIAN_POINT ( 'NONE',  ( 20.00000000000000000, -4.000000000000000000, 29.75000000000000355 ) ) ;
#38319=ORIENTED_EDGE ( 'NONE', *, *, #64830, .F. ) ;
#38332=DIRECTION ( 'NONE',  ( 0.000000000000000000, 0.000000000000000000, -1.000000000000000000 ) ) ;
#38335=ORIENTED_EDGE ( 'NONE', *, *, #54353, .T. ) ;
#38348=ORIENTED_EDGE ( 'NONE', *, *, #82525, .F. ) ;
#38412=CARTESIAN_POINT ( 'NONE',  ( 16.09615384615384670, -7.500000000000000000, 29.75000000000000355 ) ) ;
#38421=LINE ( 'NONE', #72194, #20978 ) ;
#38432=VECTOR ( 'NONE', #10312, 1000.000000000000000 ) ;
#38447=EDGE_CURVE ( 'NONE', #88550, #70465, #22670, .T. ) ;
#38451=LINE ( 'NONE', #80337, #37509 ) ;
#38460=EDGE_CURVE ( 'NONE', #61394, #27134, #77219, .T. ) ;
#38463=CARTESIAN_POINT ( 'NONE',  ( -16.81410256410256565, -3.499999999999999556, 29.75000000000000355 ) ) ;
#38476=DIRECTION ( 'NONE',  ( -1.000000000000000000, 0.000000000000000000, -0.000000000000000000 ) ) ;
#38494=LINE ( 'NONE', #33067, #51109 ) ;
#38506=LINE ( 'NONE', #38961, #88707 ) ;
#38524=DIRECTION ( 'NONE',  ( -1.000000000000000000, -0.000000000000000000, 0.000000000000000000 ) ) ;
#38534=ADVANCED_FACE ( 'NONE', ( #85712 ), #8285, .F. ) ;
#38538=VECTOR ( 'NONE', #77335, 1000.000000000000000 ) ;
#38548=CARTESIAN_POINT ( 'NONE',  ( 1.576923076923075762, -3.499999999999999556, 29.75000000000000355 ) ) ;
#38562=ORIENTED_EDGE ( 'NONE', *, *, #31910, .T. ) ;
#38563=CARTESIAN_POINT ( 'NONE',  ( -7.134615384615385025, -3.499999999999999556, 29.75000000000000355 ) ) ;
#38566=VERTEX_POINT ( 'NONE', #70427 ) ;
#38585=CARTESIAN_POINT ( 'NONE',  ( -19.50000000000000000, -3.499999999999999556, 29.75000000000000355 ) ) ;
#38586=DIRECTION ( 'NONE',  ( -1.000000000000000000, -0.000000000000000000, -0.000000000000000000 ) ) ;
#38594=CARTESIAN_POINT ( 'NONE',  ( 13.19230769230769340, -11.00000000000000000, 29.75000000000000355 ) ) ;
#38599=EDGE_CURVE ( 'NONE', #18170, #77088, #29447, .T. ) ;
#38600=CARTESIAN_POINT ( 'NONE',  ( 9.320512820512821150, -1.926643599941765039, 28.25000000000000000 ) ) ;
#38614=EDGE_CURVE ( 'NONE', #5068, #30150, #84391, .T. ) ;
#38623=CARTESIAN_POINT ( 'NONE',  ( 7.134615384615385025, -7.500000000000000000, 29.75000000000000355 ) ) ;
#38648=VERTEX_POINT ( 'NONE', #12265 ) ;
#38653=LINE ( 'NONE', #52152, #30680 ) ;
#38656=ORIENTED_EDGE ( 'NONE', *, *, #39042, .T. ) ;
#38660=EDGE_LOOP ( 'NONE', ( #43826, #65894, #65700, #49539, #78800 ) ) ;
#38665=ORIENTED_EDGE ( 'NONE', *, *, #8635, .T. ) ;
#38666=CARTESIAN_POINT ( 'NONE',  ( -9.320512820512821150, -3.499999999999999556, 29.75000000000000355 ) ) ;
#38688=FACE_OUTER_BOUND ( 'NONE', #83410, .T. ) ;
#38691=FACE_OUTER_BOUND ( 'NONE', #37148, .T. ) ;
#38715=CARTESIAN_POINT ( 'NONE',  ( 7.384615384615385025, -7.500000000000000000, 29.75000000000000355 ) ) ;
#38725=VECTOR ( 'NONE', #16745, 1000.000000000000000 ) ;
#38748=VERTEX_POINT ( 'NONE', #85 ) ;
#38755=EDGE_LOOP ( 'NONE', ( #83654, #54533, #52599, #12712 ) ) ;
#38758=CARTESIAN_POINT ( 'NONE',  ( -11.00641025641025550, -11.50000000000000000, 29.75000000000000355 ) ) ;
#38772=CARTESIAN_POINT ( 'NONE',  ( -10.28846153846153832, -11.00000000000000000, 29.75000000000000355 ) ) ;
#38776=VERTEX_POINT ( 'NONE', #76179 ) ;
#38778=EDGE_CURVE ( 'NONE', #88550, #35014, #68981, .T. ) ;
#38780=EDGE_CURVE ( 'NONE', #30410, #5644, #7287, .T. ) ;
#38783=ADVANCED_FACE ( 'NONE', ( #19467 ), #34751, .T. ) ;
#38788=PLANE ( 'NONE',  #42414 ) ;
#38803=LINE ( 'NONE', #32041, #77463 ) ;
#38829=VECTOR ( 'NONE', #48373, 1000.000000000000000 ) ;
#38835=CARTESIAN_POINT ( 'NONE',  ( -2.294871794871794712, -11.50000000000000000, 29.75000000000000355 ) ) ;
#38880=AXIS2_PLACEMENT_3D ( 'NONE', #6916, #54210, #34832 ) ;
#38885=CARTESIAN_POINT ( 'NONE',  ( -8.102564102564102200, -7.500000000000000000, 33.75000000000000000 ) ) ;
#38886=CYLINDRICAL_SURFACE ( 'NONE', #35197, 4.000000000000000000 ) ;
#38888=CIRCLE ( 'NONE', #35998, 4.000000000000000000 ) ;
#38896=PLANE ( 'NONE',  #1327 ) ;
#38911=ORIENTED_EDGE ( 'NONE', *, *, #45490, .T. ) ;
#38918=EDGE_CURVE ( 'NONE', #4960, #59157, #66665, .T. ) ;
#38944=CYLINDRICAL_SURFACE ( 'NONE', #63916, 4.000000000000000000 ) ;
#38954=FACE_OUTER_BOUND ( 'NONE', #58814, .T. ) ;
#38956=VECTOR ( 'NONE', #45589, 1000.000000000000000 ) ;
#38958=VERTEX_POINT ( 'NONE', #65761 ) ;
#38961=CARTESIAN_POINT ( 'NONE',  ( 20.00000000000000000, -4.000000000000000000, 29.75000000000000355 ) ) ;
#38967=VECTOR ( 'NONE', #66142, 1000.000000000000000 ) ;
#38968=DIRECTION ( 'NONE',  ( 1.000000000000000000, 0.000000000000000000, 0.000000000000000000 ) ) ;
#38976=ORIENTED_EDGE ( 'NONE', *, *, #60093, .T. ) ;
#38981=DIRECTION ( 'NONE',  ( 0.000000000000000000, 0.000000000000000000, -1.000000000000000000 ) ) ;
#38985=ADVANCED_FACE ( 'NONE', ( #25234 ), #59011, .T. ) ;
#38994=CARTESIAN_POINT ( 'NONE',  ( 10.03846153846153832, -7.500000000000000000, 29.75000000000000355 ) ) ;
#39001=ORIENTED_EDGE ( 'NONE', *, *, #67861, .T. ) ;
#39003=VECTOR ( 'NONE', #36508, 1000.000000000000000 ) ;
#39025=ORIENTED_EDGE ( 'NONE', *, *, #16353, .T. ) ;
#39041=DIRECTION ( 'NONE',  ( 0.000000000000000000, 0.000000000000000000, 1.000000000000000000 ) ) ;
#39042=EDGE_CURVE ( 'NONE', #38776, #15438, #77291, .T. ) ;
#39044=ADVANCED_FACE ( 'NONE', ( #80795 ), #27157, .F. ) ;
#39053=EDGE_CURVE ( 'NONE', #34461, #16936, #47870, .T. ) ;
#39061=PLANE ( 'NONE',  #11424 ) ;
#39071=LINE ( 'NONE', #74175, #12397 ) ;
#39084=CARTESIAN_POINT ( 'NONE',  ( 7.134615384615385025, -3.499999999999999556, 29.75000000000000355 ) ) ;
#39092=EDGE_LOOP ( 'NONE', ( #6261, #78009, #5964, #55847, #14091 ) ) ;
#39106=ORIENTED_EDGE ( 'NONE', *, *, #201, .T. ) ;
#39118=ORIENTED_EDGE ( 'NONE', *, *, #70213, .F. ) ;
#39119=ORIENTED_EDGE ( 'NONE', *, *, #56126, .T. ) ;
#39124=CARTESIAN_POINT ( 'NONE',  ( -19.50000000000000000, -3.499999999999999556, 29.75000000000000355 ) ) ;
#39138=CYLINDRICAL_SURFACE ( 'NONE', #36191, 4.000000000000000000 ) ;
#39153=EDGE_CURVE ( 'NONE', #55647, #54542, #54174, .T. ) ;
#39156=FACE_OUTER_BOUND ( 'NONE', #50170, .T. ) ;
#39160=LINE ( 'NONE', #73832, #54941 ) ;
#39197=ORIENTED_EDGE ( 'NONE', *, *, #23278, .F. ) ;
#39202=LINE ( 'NONE', #38303, #1926 ) ;
#39228=DIRECTION ( 'NONE',  ( 0.000000000000000000, 0.000000000000000000, -1.000000000000000000 ) ) ;
#39241=FACE_OUTER_BOUND ( 'NONE', #25163, .T. ) ;
#39247=EDGE_LOOP ( 'NONE', ( #77417, #69117, #66823, #28147 ) ) ;
#39253=DIRECTION ( 'NONE',  ( 1.000000000000000000, 0.000000000000000000, 0.000000000000000000 ) ) ;
#39256=EDGE_CURVE ( 'NONE', #6548, #27134, #36146, .T. ) ;
#39264=AXIS2_PLACEMENT_3D ( 'NONE', #40361, #41682, #60611 ) ;
#39278=ORIENTED_EDGE ( 'NONE', *, *, #1517, .T. ) ;
#39282=CARTESIAN_POINT ( 'NONE',  ( 0.000000000000000000, -2.085786437626902856, 29.25000000000000000 ) ) ;
#39301=CARTESIAN_POINT ( 'NONE',  ( 20.00000000000000000, -4.000000000000000000, 29.75000000000000355 ) ) ;
#39315=ORIENTED_EDGE ( 'NONE', *, *, #33339, .T. ) ;
#39329=CIRCLE ( 'NONE', #78142, 4.000000000000000000 ) ;
#39341=ORIENTED_EDGE ( 'NONE', *, *, #58025, .T. ) ;
#39344=DIRECTION ( 'NONE',  ( 0.000000000000000000, 0.000000000000000000, 1.000000000000000000 ) ) ;
#39345=EDGE_CURVE ( 'NONE', #75643, #24805, #23931, .T. ) ;
#39407=ORIENTED_EDGE ( 'NONE', *, *, #16155, .F. ) ;
#39419=CARTESIAN_POINT ( 'NONE',  ( 1.576923076923076428, -4.000000000000000000, 29.75000000000000355 ) ) ;
#39428=LINE ( 'NONE', #65539, #49811 ) ;
#39433=AXIS2_PLACEMENT_3D ( 'NONE', #24827, #52299, #73026 ) ;
#39436=DIRECTION ( 'NONE',  ( 1.000000000000000000, 0.000000000000000000, 0.000000000000000000 ) ) ;
#39449=VECTOR ( 'NONE', #12651, 1000.000000000000000 ) ;
#39484=VECTOR ( 'NONE', #62722, 1000.000000000000000 ) ;
#39491=DIRECTION ( 'NONE',  ( -0.000000000000000000, 0.000000000000000000, 1.000000000000000000 ) ) ;
#39500=PLANE ( 'NONE',  #85013 ) ;
#39504=DIRECTION ( 'NONE',  ( 1.000000000000000000, 0.000000000000000000, 0.000000000000000000 ) ) ;
#39533=CARTESIAN_POINT ( 'NONE',  ( 15.12820512820512953, -3.499999999999999556, 29.75000000000000355 ) ) ;
#39537=CARTESIAN_POINT ( 'NONE',  ( 4.480769230769229061, -7.500000000000000000, 29.75000000000000355 ) ) ;
#39552=DIRECTION ( 'NONE',  ( -1.000000000000000000, -0.000000000000000000, -0.000000000000000000 ) ) ;
#39560=ORIENTED_EDGE ( 'NONE', *, *, #24136, .T. ) ;
#39562=CYLINDRICAL_SURFACE ( 'NONE', #88985, 4.000000000000000000 ) ;
#39566=DIRECTION ( 'NONE',  ( 0.000000000000000000, 0.000000000000000000, -1.000000000000000000 ) ) ;
#39575=ORIENTED_EDGE ( 'NONE', *, *, #88791, .F. ) ;
#39585=VECTOR ( 'NONE', #27072, 1000.000000000000000 ) ;
#39596=DIRECTION ( 'NONE',  ( 0.000000000000000000, 0.000000000000000000, -1.000000000000000000 ) ) ;
#39602=LINE ( 'NONE', #31489, #81641 ) ;
#39607=CARTESIAN_POINT ( 'NONE',  ( -18.75000000000000000, -3.499999999999999556, 29.75000000000000355 ) ) ;
#39608=( LENGTH_UNIT ( ) NAMED_UNIT ( * ) SI_UNIT ( .MILLI., .METRE. ) );
#39627=CARTESIAN_POINT ( 'NONE',  ( -19.50000000000000000, -3.499999999999999556, 29.75000000000000355 ) ) ;
#39629=LINE ( 'NONE', #67087, #13167 ) ;
#39651=EDGE_CURVE ( 'NONE', #42406, #82638, #5425, .T. ) ;
#39672=EDGE_LOOP ( 'NONE', ( #28744, #7207, #54834, #24808, #39919 ) ) ;
#39678=CIRCLE ( 'NONE', #51133, 4.000000000000000000 ) ;
#39682=CARTESIAN_POINT ( 'NONE',  ( -5.448717948717948012, -11.00000000000000000, 29.75000000000000355 ) ) ;
#39702=CARTESIAN_POINT ( 'NONE',  ( 0.000000000000000000, -11.00000000000000000, 29.75000000000000355 ) ) ;
#39710=EDGE_LOOP ( 'NONE', ( #81024, #17707, #59081, #49778 ) ) ;
#39726=DIRECTION ( 'NONE',  ( 0.000000000000000000, -1.000000000000000000, 0.000000000000000000 ) ) ;
#39734=DIRECTION ( 'NONE',  ( 0.000000000000000000, 0.000000000000000000, -1.000000000000000000 ) ) ;
#39740=CARTESIAN_POINT ( 'NONE',  ( -18.75000000000000000, -7.500000000000000000, 29.75000000000000355 ) ) ;
#39744=AXIS2_PLACEMENT_3D ( 'NONE', #79615, #17914, #45368 ) ;
#39746=DIRECTION ( 'NONE',  ( 0.000000000000000000, 0.000000000000000000, -1.000000000000000000 ) ) ;
#39748=ORIENTED_EDGE ( 'NONE', *, *, #59833, .T. ) ;
#39762=CARTESIAN_POINT ( 'NONE',  ( 13.19230769230769340, -11.50000000000000000, 29.75000000000000355 ) ) ;
#39765=EDGE_CURVE ( 'NONE', #84875, #65515, #13759, .T. ) ;
#39773=CARTESIAN_POINT ( 'NONE',  ( 4.480769230769229061, -7.500000000000000000, 29.75000000000000355 ) ) ;
#39785=DIRECTION ( 'NONE',  ( 0.000000000000000000, 0.000000000000000000, -1.000000000000000000 ) ) ;
#39795=ORIENTED_EDGE ( 'NONE', *, *, #15711, .F. ) ;
#39812=LINE ( 'NONE', #33048, #31807 ) ;
#39841=EDGE_LOOP ( 'NONE', ( #27230, #34023, #7481, #19218 ) ) ;
#39848=EDGE_CURVE ( 'NONE', #53945, #79249, #55627, .T. ) ;
#39852=DIRECTION ( 'NONE',  ( -0.000000000000000000, 1.000000000000000000, -0.000000000000000000 ) ) ;
#39859=EDGE_CURVE ( 'NONE', #49704, #72244, #48609, .T. ) ;
#39868=ADVANCED_FACE ( 'NONE', ( #42138 ), #691, .F. ) ;
#39882=DIRECTION ( 'NONE',  ( 0.000000000000000000, 0.000000000000000000, 1.000000000000000000 ) ) ;
#39883=EDGE_CURVE ( 'NONE', #3633, #86305, #78828, .T. ) ;
#39885=LINE ( 'NONE', #81752, #76734 ) ;
#39888=AXIS2_PLACEMENT_3D ( 'NONE', #46976, #13641, #66819 ) ;
#39894=AXIS2_PLACEMENT_3D ( 'NONE', #48402, #39896, #41218 ) ;
#39896=DIRECTION ( 'NONE',  ( 1.000000000000000000, 0.000000000000000000, 0.000000000000000000 ) ) ;
#39901=VERTEX_POINT ( 'NONE', #84454 ) ;
#39910=CARTESIAN_POINT ( 'NONE',  ( -11.97435897435897623, -4.000000000000000000, 29.75000000000000355 ) ) ;
#39912=EDGE_CURVE ( 'NONE', #37056, #4960, #23181, .T. ) ;
#39915=DIRECTION ( 'NONE',  ( 1.000000000000000000, 0.000000000000000000, 0.000000000000000000 ) ) ;
#39919=ORIENTED_EDGE ( 'NONE', *, *, #82254, .T. ) ;
#39920=DIRECTION ( 'NONE',  ( -1.000000000000000000, -0.000000000000000000, -0.000000000000000000 ) ) ;
#39926=DIRECTION ( 'NONE',  ( -1.000000000000000000, -0.000000000000000000, -0.000000000000000000 ) ) ;
#39933=LINE ( 'NONE', #59745, #56101 ) ;
#39943=CARTESIAN_POINT ( 'NONE',  ( 16.09615384615384670, -4.000000000000000000, 29.75000000000000355 ) ) ;
#39962=ORIENTED_EDGE ( 'NONE', *, *, #63219, .F. ) ;
#39963=CARTESIAN_POINT ( 'NONE',  ( 4.480769230769229061, -11.50000000000000000, 29.75000000000000355 ) ) ;
#39967=CARTESIAN_POINT ( 'NONE',  ( -0.6089743589743593644, -7.500000000000000000, 29.75000000000000355 ) ) ;
#39971=DIRECTION ( 'NONE',  ( -1.000000000000000000, 0.000000000000000000, -0.000000000000000000 ) ) ;
#39975=VECTOR ( 'NONE', #26114, 1000.000000000000000 ) ;
#39988=AXIS2_PLACEMENT_3D ( 'NONE', #32826, #72917, #11223 ) ;
#39993=DIRECTION ( 'NONE',  ( 0.000000000000000000, 0.000000000000000000, -1.000000000000000000 ) ) ;
#40007=CARTESIAN_POINT ( 'NONE',  ( -5.448717948717948012, -7.500000000000000000, 33.75000000000000000 ) ) ;
#40029=EDGE_CURVE ( 'NONE', #30874, #11346, #6902, .T. ) ;
#40041=CARTESIAN_POINT ( 'NONE',  ( 1.326923076923076206, -3.499999999999999556, 29.75000000000000355 ) ) ;
#40043=LINE ( 'NONE', #9550, #24134 ) ;
#40047=CARTESIAN_POINT ( 'NONE',  ( -9.070512820512819374, -3.499999999999999556, 29.75000000000000355 ) ) ;
#40057=DIRECTION ( 'NONE',  ( 1.000000000000000000, 0.000000000000000000, 0.000000000000000000 ) ) ;
#40059=DIRECTION ( 'NONE',  ( -1.000000000000000000, 0.000000000000000000, -0.000000000000000000 ) ) ;
#40067=EDGE_CURVE ( 'NONE', #15438, #48507, #5134, .T. ) ;
#40076=VECTOR ( 'NONE', #66783, 1000.000000000000000 ) ;
#40106=DIRECTION ( 'NONE',  ( -1.000000000000000000, -0.000000000000000000, -0.000000000000000000 ) ) ;
#40110=ORIENTED_EDGE ( 'NONE', *, *, #67265, .T. ) ;
#40122=VERTEX_POINT ( 'NONE', #68605 ) ;
#40135=CARTESIAN_POINT ( 'NONE',  ( -19.50000000000000000, -3.499999999999999556, 29.75000000000000355 ) ) ;
#40141=ORIENTED_EDGE ( 'NONE', *, *, #29120, .T. ) ;
#40184=AXIS2_PLACEMENT_3D ( 'NONE', #66789, #71758, #10064 ) ;
#40185=ORIENTED_EDGE ( 'NONE', *, *, #22837, .F. ) ;
#40214=VECTOR ( 'NONE', #9015, 1000.000000000000000 ) ;
#40223=DIRECTION ( 'NONE',  ( 1.000000000000000000, 0.000000000000000000, 0.000000000000000000 ) ) ;
#40230=VECTOR ( 'NONE', #79086, 1000.000000000000000 ) ;
#40239=ORIENTED_EDGE ( 'NONE', *, *, #53430, .T. ) ;
#40248=FACE_OUTER_BOUND ( 'NONE', #28469, .T. ) ;
#40252=ORIENTED_EDGE ( 'NONE', *, *, #79741, .F. ) ;
#40256=ORIENTED_EDGE ( 'NONE', *, *, #24576, .T. ) ;
#40257=DIRECTION ( 'NONE',  ( -1.000000000000000000, -0.000000000000000000, -0.000000000000000000 ) ) ;
#40272=DIRECTION ( 'NONE',  ( -0.000000000000000000, 1.000000000000000000, -0.000000000000000000 ) ) ;
#40290=CARTESIAN_POINT ( 'NONE',  ( -0.3589743589743593088, -7.500000000000000000, 33.75000000000000000 ) ) ;
#40309=LINE ( 'NONE', #641, #2291 ) ;
#40318=ORIENTED_EDGE ( 'NONE', *, *, #25018, .F. ) ;
#40335=CARTESIAN_POINT ( 'NONE',  ( 9.320512820512821150, -1.926643599941765039, 29.65000000000000213 ) ) ;
#40346=ORIENTED_EDGE ( 'NONE', *, *, #41092, .F. ) ;
#40355=AXIS2_PLACEMENT_3D ( 'NONE', #15680, #62084, #69730 ) ;
#40359=ORIENTED_EDGE ( 'NONE', *, *, #70151, .F. ) ;
#40361=CARTESIAN_POINT ( 'NONE',  ( -11.00641025641025550, -3.499999999999999556, 29.75000000000000355 ) ) ;
#40378=DIRECTION ( 'NONE',  ( -1.000000000000000000, -0.000000000000000000, 0.000000000000000000 ) ) ;
#40385=DIRECTION ( 'NONE',  ( -0.000000000000000000, 1.000000000000000000, -0.000000000000000000 ) ) ;
#40390=DIRECTION ( 'NONE',  ( 1.000000000000000000, 0.000000000000000000, 0.000000000000000000 ) ) ;
#40409=DIRECTION ( 'NONE',  ( 0.000000000000000000, 0.000000000000000000, -1.000000000000000000 ) ) ;
#40437=LINE ( 'NONE', #41757, #86982 ) ;
#40460=DIRECTION ( 'NONE',  ( 1.000000000000000000, 0.000000000000000000, 0.000000000000000000 ) ) ;
#40475=LINE ( 'NONE', #46774, #38967 ) ;
#40489=CIRCLE ( 'NONE', #28986, 4.000000000000000000 ) ;
#40490=CYLINDRICAL_SURFACE ( 'NONE', #85597, 4.000000000000000000 ) ;
#40494=EDGE_CURVE ( 'NONE', #73366, #61830, #32801, .T. ) ;
#40507=DIRECTION ( 'NONE',  ( -1.000000000000000000, 0.000000000000000000, -0.000000000000000000 ) ) ;
#40511=CARTESIAN_POINT ( 'NONE',  ( -17.78205128205128105, -11.50000000000000000, 29.75000000000000355 ) ) ;
#40514=EDGE_CURVE ( 'NONE', #62375, #48447, #44276, .T. ) ;
#40517=PLANE ( 'NONE',  #87765 ) ;
#40554=VERTEX_POINT ( 'NONE', #63059 ) ;
#40572=DIRECTION ( 'NONE',  ( 1.000000000000000000, 0.000000000000000000, 0.000000000000000000 ) ) ;
#40576=CARTESIAN_POINT ( 'NONE',  ( -19.50000000000000000, -3.499999999999999556, 29.75000000000000355 ) ) ;
#40583=DIRECTION ( 'NONE',  ( 0.000000000000000000, 0.000000000000000000, 1.000000000000000000 ) ) ;
#40590=CARTESIAN_POINT ( 'NONE',  ( -19.50000000000000000, -11.50000000000000000, 29.75000000000000355 ) ) ;
#40595=VERTEX_POINT ( 'NONE', #50432 ) ;
#40604=PLANE ( 'NONE',  #27344 ) ;
#40605=ORIENTED_EDGE ( 'NONE', *, *, #2360, .T. ) ;
#40619=EDGE_LOOP ( 'NONE', ( #74407, #40239, #45486, #3638, #40847 ) ) ;
#40622=VECTOR ( 'NONE', #69822, 1000.000000000000000 ) ;
#40626=VERTEX_POINT ( 'NONE', #65280 ) ;
#40643=ORIENTED_EDGE ( 'NONE', *, *, #82132, .T. ) ;
#40647=AXIS2_PLACEMENT_3D ( 'NONE', #14790, #29631, #42266 ) ;
#40650=EDGE_CURVE ( 'NONE', #40554, #15501, #47412, .T. ) ;
#40657=DIRECTION ( 'NONE',  ( -1.000000000000000000, -0.000000000000000000, -0.000000000000000000 ) ) ;
#40665=EDGE_CURVE ( 'NONE', #21924, #7139, #80489, .T. ) ;
#40672=ADVANCED_FACE ( 'NONE', ( #60750 ), #52655, .F. ) ;
#40693=ORIENTED_EDGE ( 'NONE', *, *, #21182, .F. ) ;
#40695=ORIENTED_EDGE ( 'NONE', *, *, #67606, .T. ) ;
#40702=DIRECTION ( 'NONE',  ( -1.000000000000000000, -0.000000000000000000, 0.000000000000000000 ) ) ;
#40704=ORIENTED_EDGE ( 'NONE', *, *, #64805, .T. ) ;
#40717=LINE ( 'NONE', #6481, #6637 ) ;
#40722=DIRECTION ( 'NONE',  ( 1.000000000000000000, 0.000000000000000000, 0.000000000000000000 ) ) ;
#40740=EDGE_CURVE ( 'NONE', #83471, #48416, #18883, .T. ) ;
#40748=ORIENTED_EDGE ( 'NONE', *, *, #54458, .F. ) ;
#40751=CARTESIAN_POINT ( 'NONE',  ( -19.50000000000000000, -11.50000000000000000, 29.75000000000000355 ) ) ;
#40764=DIRECTION ( 'NONE',  ( -1.000000000000000000, -0.000000000000000000, -0.000000000000000000 ) ) ;
#40773=EDGE_CURVE ( 'NONE', #68727, #4543, #11236, .T. ) ;
#40790=ORIENTED_EDGE ( 'NONE', *, *, #41534, .F. ) ;
#40793=ORIENTED_EDGE ( 'NONE', *, *, #60356, .F. ) ;
#40794=DIRECTION ( 'NONE',  ( 1.000000000000000000, 0.000000000000000000, 0.000000000000000000 ) ) ;
#40802=DIRECTION ( 'NONE',  ( -0.000000000000000000, 1.000000000000000000, -0.000000000000000000 ) ) ;
#40822=CARTESIAN_POINT ( 'NONE',  ( 20.00000000000000000, -4.000000000000000000, 29.75000000000000355 ) ) ;
#40847=ORIENTED_EDGE ( 'NONE', *, *, #2502, .T. ) ;
#40866=AXIS2_PLACEMENT_3D ( 'NONE', #7558, #26946, #14759 ) ;
#40899=DIRECTION ( 'NONE',  ( -1.000000000000000000, -0.000000000000000000, -0.000000000000000000 ) ) ;
#40919=CARTESIAN_POINT ( 'NONE',  ( 1.326923076923075762, -3.499999999999999556, 29.75000000000000355 ) ) ;
#40925=ORIENTED_EDGE ( 'NONE', *, *, #54155, .T. ) ;
#40927=ORIENTED_EDGE ( 'NONE', *, *, #89074, .T. ) ;
#40939=CARTESIAN_POINT ( 'NONE',  ( -19.50000000000000000, -3.499999999999999556, 29.75000000000000355 ) ) ;
#40945=DIRECTION ( 'NONE',  ( 0.000000000000000000, 0.000000000000000000, -1.000000000000000000 ) ) ;
#40946=VERTEX_POINT ( 'NONE', #2579 ) ;
#40955=ORIENTED_EDGE ( 'NONE', *, *, #32130, .T. ) ;
#40984=ORIENTED_EDGE ( 'NONE', *, *, #8813, .T. ) ;
#40988=EDGE_CURVE ( 'NONE', #15501, #40554, #63237, .T. ) ;
#41006=DIRECTION ( 'NONE',  ( -0.000000000000000000, 1.000000000000000000, -0.000000000000000000 ) ) ;
#41009=DIRECTION ( 'NONE',  ( -1.000000000000000000, -0.000000000000000000, -0.000000000000000000 ) ) ;
#41010=EDGE_CURVE ( 'NONE', #71780, #65753, #8613, .T. ) ;
#41021=CARTESIAN_POINT ( 'NONE',  ( 12.22435897435897267, -3.499999999999999556, 29.75000000000000355 ) ) ;
#41038=CARTESIAN_POINT ( 'NONE',  ( 10.03846153846153832, -4.000000000000000000, 29.75000000000000355 ) ) ;
#41041=EDGE_CURVE ( 'NONE', #81906, #29384, #45345, .T. ) ;
#41043=ORIENTED_EDGE ( 'NONE', *, *, #9325, .F. ) ;
#41044=CARTESIAN_POINT ( 'NONE',  ( 1.576923076923075762, -3.499999999999999556, 29.75000000000000355 ) ) ;
#41047=CARTESIAN_POINT ( 'NONE',  ( 13.91025641025641235, -11.00000000000000000, 29.75000000000000355 ) ) ;
#41052=VECTOR ( 'NONE', #16983, 1000.000000000000000 ) ;
#41062=DIRECTION ( 'NONE',  ( -1.000000000000000000, -0.000000000000000000, 0.000000000000000000 ) ) ;
#41063=VECTOR ( 'NONE', #24921, 1000.000000000000000 ) ;
#41066=LINE ( 'NONE', #39301, #49967 ) ;
#41068=ORIENTED_EDGE ( 'NONE', *, *, #37084, .T. ) ;
#41072=ORIENTED_EDGE ( 'NONE', *, *, #60991, .F. ) ;
#41075=ORIENTED_EDGE ( 'NONE', *, *, #23642, .T. ) ;
#41078=DIRECTION ( 'NONE',  ( -0.000000000000000000, 0.000000000000000000, 1.000000000000000000 ) ) ;
#41087=ADVANCED_FACE ( 'NONE', ( #11579 ), #39061, .F. ) ;
#41091=CARTESIAN_POINT ( 'NONE',  ( 17.78205128205128105, -7.500000000000000000, 29.75000000000000355 ) ) ;
#41092=EDGE_CURVE ( 'NONE', #59157, #60898, #80484, .T. ) ;
#41094=EDGE_CURVE ( 'NONE', #24532, #29384, #18633, .T. ) ;
#41099=ORIENTED_EDGE ( 'NONE', *, *, #7551, .F. ) ;
#41100=EDGE_CURVE ( 'NONE', #81906, #30233, #25083, .T. ) ;
#41103=ORIENTED_EDGE ( 'NONE', *, *, #9819, .T. ) ;
#41115=AXIS2_PLACEMENT_3D ( 'NONE', #22595, #50064, #37431 ) ;
#41126=DIRECTION ( 'NONE',  ( 0.000000000000000000, 0.000000000000000000, -1.000000000000000000 ) ) ;
#41137=CARTESIAN_POINT ( 'NONE',  ( 20.00000000000000000, -7.500000000000000000, 33.75000000000000000 ) ) ;
#41145=VECTOR ( 'NONE', #12824, 1000.000000000000000 ) ;
#41148=DIRECTION ( 'NONE',  ( -0.000000000000000000, 1.000000000000000000, -0.000000000000000000 ) ) ;
#41157=PLANE ( 'NONE',  #38880 ) ;
#41171=FACE_OUTER_BOUND ( 'NONE', #39092, .T. ) ;
#41204=CARTESIAN_POINT ( 'NONE',  ( 2.294871794871793824, -3.499999999999999556, 29.75000000000000355 ) ) ;
#41206=VECTOR ( 'NONE', #15491, 1000.000000000000000 ) ;
#41211=ORIENTED_EDGE ( 'NONE', *, *, #84948, .T. ) ;
#41217=CARTESIAN_POINT ( 'NONE',  ( 4.480769230769229061, -7.500000000000000000, 29.75000000000000355 ) ) ;
#41218=DIRECTION ( 'NONE',  ( 0.000000000000000000, 0.000000000000000000, -1.000000000000000000 ) ) ;
#41222=ORIENTED_EDGE ( 'NONE', *, *, #14727, .F. ) ;
#41259=CARTESIAN_POINT ( 'NONE',  ( 10.03846153846153832, -3.499999999999999556, 29.75000000000000355 ) ) ;
#41262=ORIENTED_EDGE ( 'NONE', *, *, #26894, .T. ) ;
#41277=VECTOR ( 'NONE', #76248, 1000.000000000000000 ) ;
#41278=PLANE ( 'NONE',  #30261 ) ;
#41288=ORIENTED_EDGE ( 'NONE', *, *, #87197, .T. ) ;
#41297=ORIENTED_EDGE ( 'NONE', *, *, #72421, .T. ) ;
#41310=CARTESIAN_POINT ( 'NONE',  ( -15.12820512820512953, -3.499999999999999556, 29.75000000000000355 ) ) ;
#41316=CARTESIAN_POINT ( 'NONE',  ( -13.91025641025641058, -7.500000000000000000, 29.75000000000000355 ) ) ;
#41317=EDGE_LOOP ( 'NONE', ( #64936, #86505, #64860, #88353 ) ) ;
#41319=DIRECTION ( 'NONE',  ( -1.000000000000000000, -0.000000000000000000, -0.000000000000000000 ) ) ;
#41323=ORIENTED_EDGE ( 'NONE', *, *, #66680, .T. ) ;
#41326=LINE ( 'NONE', #68795, #23119 ) ;
#41344=LINE ( 'NONE', #69258, #49786 ) ;
#41350=SURFACE_SIDE_STYLE ('',( #47209 ) ) ;
#41353=CYLINDRICAL_SURFACE ( 'NONE', #2972, 4.000000000000000000 ) ;
#41367=AXIS2_PLACEMENT_3D ( 'NONE', #35465, #75558, #15641 ) ;
#41372=VECTOR ( 'NONE', #70180, 1000.000000000000000 ) ;
#41381=DIRECTION ( 'NONE',  ( -0.000000000000000000, 0.000000000000000000, 1.000000000000000000 ) ) ;
#41390=CARTESIAN_POINT ( 'NONE',  ( -19.50000000000000000, -3.499999999999999556, 29.75000000000000355 ) ) ;
#41402=ORIENTED_EDGE ( 'NONE', *, *, #72354, .T. ) ;
#41420=DIRECTION ( 'NONE',  ( 1.000000000000000000, 0.000000000000000000, 0.000000000000000000 ) ) ;
#41428=VECTOR ( 'NONE', #76127, 1000.000000000000000 ) ;
#41467=ADVANCED_FACE ( 'NONE', ( #19008 ), #67644, .F. ) ;
#41472=ORIENTED_EDGE ( 'NONE', *, *, #84530, .T. ) ;
#41479=DIRECTION ( 'NONE',  ( -1.000000000000000000, -0.000000000000000000, -0.000000000000000000 ) ) ;
#41487=CARTESIAN_POINT ( 'NONE',  ( -19.00000000000000000, -7.500000000000000000, 29.75000000000000355 ) ) ;
#41489=DIRECTION ( 'NONE',  ( 1.000000000000000000, 0.000000000000000000, 0.000000000000000000 ) ) ;
#41490=EDGE_CURVE ( 'NONE', #85035, #75229, #47805, .T. ) ;
#41499=ADVANCED_FACE ( 'NONE', ( #54108 ), #6815, .F. ) ;
#41508=CARTESIAN_POINT ( 'NONE',  ( -11.97435897435897267, -3.499999999999999556, 29.75000000000000355 ) ) ;
#41519=ORIENTED_EDGE ( 'NONE', *, *, #83803, .T. ) ;
#41534=EDGE_CURVE ( 'NONE', #26475, #38566, #28422, .T. ) ;
#41549=CARTESIAN_POINT ( 'NONE',  ( 0.000000000000000000, -11.00000000000000000, 29.75000000000000355 ) ) ;
#41557=DIRECTION ( 'NONE',  ( 0.000000000000000000, -1.000000000000000000, 0.000000000000000000 ) ) ;
#41567=CARTESIAN_POINT ( 'NONE',  ( 9.070512820512819374, -3.499999999999999556, 29.75000000000000355 ) ) ;
#41570=ORIENTED_EDGE ( 'NONE', *, *, #80, .T. ) ;
#41596=CYLINDRICAL_SURFACE ( 'NONE', #61879, 4.000000000000000000 ) ;
#41626=ORIENTED_EDGE ( 'NONE', *, *, #74615, .F. ) ;
#41629=PLANE ( 'NONE',  #61244 ) ;
#41652=ORIENTED_EDGE ( 'NONE', *, *, #88791, .T. ) ;
#41678=LINE ( 'NONE', #77227, #82020 ) ;
#41682=DIRECTION ( 'NONE',  ( -0.000000000000000000, 0.000000000000000000, 1.000000000000000000 ) ) ;
#41683=DIRECTION ( 'NONE',  ( 1.000000000000000000, 0.000000000000000000, 0.000000000000000000 ) ) ;
#41697=PLANE ( 'NONE',  #75136 ) ;
#41704=VECTOR ( 'NONE', #71999, 1000.000000000000000 ) ;
#41726=CARTESIAN_POINT ( 'NONE',  ( -17.06410256410256565, -11.50000000000000000, 29.75000000000000355 ) ) ;
#41750=EDGE_LOOP ( 'NONE', ( #75143, #10293, #77976, #2678 ) ) ;
#41757=CARTESIAN_POINT ( 'NONE',  ( -19.50000000000000000, -11.50000000000000000, 29.75000000000000355 ) ) ;
#41768=VECTOR ( 'NONE', #51542, 1000.000000000000000 ) ;
#41780=ADVANCED_FACE ( 'NONE', ( #88712 ), #40517, .T. ) ;
#41803=EDGE_LOOP ( 'NONE', ( #6849, #49355, #23465, #3992 ) ) ;
#41805=CARTESIAN_POINT ( 'NONE',  ( -7.134615384615385025, -7.500000000000000000, 29.75000000000000355 ) ) ;
#41810=CARTESIAN_POINT ( 'NONE',  ( 2.294871794871793380, -7.500000000000000000, 29.75000000000000355 ) ) ;
#41816=CARTESIAN_POINT ( 'NONE',  ( 20.00000000000000000, -4.000000000000000000, 29.75000000000000355 ) ) ;
#41827=DIRECTION ( 'NONE',  ( 0.000000000000000000, 1.000000000000000000, 0.000000000000000000 ) ) ;
#41831=CYLINDRICAL_SURFACE ( 'NONE', #32514, 4.000000000000000000 ) ;
#41835=AXIS2_PLACEMENT_3D ( 'NONE', #57844, #65029, #3340 ) ;
#41874=EDGE_CURVE ( 'NONE', #64241, #78478, #42286, .T. ) ;
#41893=DIRECTION ( 'NONE',  ( 0.000000000000000000, 0.000000000000000000, -1.000000000000000000 ) ) ;
#41897=AXIS2_PLACEMENT_3D ( 'NONE', #10762, #59392, #58483 ) ;
#41899=LINE ( 'NONE', #69366, #78389 ) ;
#41901=CARTESIAN_POINT ( 'NONE',  ( -19.50000000000000000, -11.50000000000000000, 29.75000000000000355 ) ) ;
#41903=ORIENTED_EDGE ( 'NONE', *, *, #76194, .F. ) ;
#41907=CIRCLE ( 'NONE', #56297, 4.000000000000000000 ) ;
#41922=ORIENTED_EDGE ( 'NONE', *, *, #52615, .F. ) ;
#41951=ORIENTED_EDGE ( 'NONE', *, *, #63439, .F. ) ;
#41952=LINE ( 'NONE', #9054, #78632 ) ;
#41962=DIRECTION ( 'NONE',  ( -0.000000000000000000, 1.000000000000000000, -0.000000000000000000 ) ) ;
#41967=VECTOR ( 'NONE', #42679, 1000.000000000000000 ) ;
#41969=ORIENTED_EDGE ( 'NONE', *, *, #23529, .T. ) ;
#41970=CARTESIAN_POINT ( 'NONE',  ( 10.28846153846153832, -3.499999999999999556, 29.75000000000000355 ) ) ;
#41977=VECTOR ( 'NONE', #51001, 1000.000000000000000 ) ;
#41982=ADVANCED_FACE ( 'NONE', ( #48134 ), #75604, .F. ) ;
#42009=ORIENTED_EDGE ( 'NONE', *, *, #78124, .T. ) ;
#42018=VERTEX_POINT ( 'NONE', #44029 ) ;
#42021=CARTESIAN_POINT ( 'NONE',  ( 10.03846153846153832, -1.926643599941765039, 28.25000000000000000 ) ) ;
#42023=EDGE_LOOP ( 'NONE', ( #23263, #17529, #48776, #6369, #30480 ) ) ;
#42025=EDGE_LOOP ( 'NONE', ( #64810, #87013, #6789, #31000 ) ) ;
#42027=DIRECTION ( 'NONE',  ( -1.000000000000000000, -0.000000000000000000, -0.000000000000000000 ) ) ;
#42031=DIRECTION ( 'NONE',  ( -1.000000000000000000, -0.000000000000000000, 0.000000000000000000 ) ) ;
#42050=DIRECTION ( 'NONE',  ( 0.000000000000000000, 0.000000000000000000, 1.000000000000000000 ) ) ;
#42055=DIRECTION ( 'NONE',  ( 1.000000000000000000, 0.000000000000000000, 0.000000000000000000 ) ) ;
#42056=ORIENTED_EDGE ( 'NONE', *, *, #34944, .F. ) ;
#42087=CARTESIAN_POINT ( 'NONE',  ( -13.19230769230769162, -11.00000000000000000, 29.75000000000000355 ) ) ;
#42090=EDGE_CURVE ( 'NONE', #6115, #60613, #85919, .T. ) ;
#42094=VECTOR ( 'NONE', #28530, 1000.000000000000000 ) ;
#42095=DIRECTION ( 'NONE',  ( -1.000000000000000000, -0.000000000000000000, -0.000000000000000000 ) ) ;
#42099=CARTESIAN_POINT ( 'NONE',  ( 17.78205128205128105, -4.000000000000000000, 29.75000000000000355 ) ) ;
#42138=FACE_OUTER_BOUND ( 'NONE', #75084, .T. ) ;
#42153=CARTESIAN_POINT ( 'NONE',  ( -10.28846153846153832, -3.499999999999999556, 29.75000000000000355 ) ) ;
#42182=CARTESIAN_POINT ( 'NONE',  ( 10.03846153846153832, -7.500000000000000000, 33.75000000000000000 ) ) ;
#42189=ADVANCED_FACE ( 'NONE', ( #4838 ), #59326, .F. ) ;
#42190=LINE ( 'NONE', #72301, #49230 ) ;
#42207=ORIENTED_EDGE ( 'NONE', *, *, #73130, .F. ) ;
#42208=AXIS2_PLACEMENT_3D ( 'NONE', #17499, #59365, #39566 ) ;
#42210=LINE ( 'NONE', #69665, #83255 ) ;
#42254=CARTESIAN_POINT ( 'NONE',  ( 1.326923076923075762, -7.500000000000000000, 33.75000000000000000 ) ) ;
#42263=EDGE_CURVE ( 'NONE', #16936, #71861, #24536, .T. ) ;
#42266=DIRECTION ( 'NONE',  ( 0.000000000000000000, 0.000000000000000000, -1.000000000000000000 ) ) ;
#42278=DIRECTION ( 'NONE',  ( -0.000000000000000000, 1.000000000000000000, -0.000000000000000000 ) ) ;
#42286=LINE ( 'NONE', #49026, #37389 ) ;
#42296=EDGE_CURVE ( 'NONE', #52150, #73790, #45654, .T. ) ;
#42297=ORIENTED_EDGE ( 'NONE', *, *, #4011, .T. ) ;
#42298=CARTESIAN_POINT ( 'NONE',  ( 10.03846153846153832, -11.00000000000000000, 29.75000000000000355 ) ) ;
#42303=EDGE_CURVE ( 'NONE', #15714, #53825, #30365, .T. ) ;
#42308=ORIENTED_EDGE ( 'NONE', *, *, #42296, .T. ) ;
#42319=ORIENTED_EDGE ( 'NONE', *, *, #39256, .F. ) ;
#42340=APPLICATION_CONTEXT ( 'automotive_design' ) ;
#42346=CARTESIAN_POINT ( 'NONE',  ( 20.00000000000000000, -4.000000000000000000, 29.75000000000000355 ) ) ;
#42362=DIRECTION ( 'NONE',  ( -1.000000000000000000, 0.000000000000000000, -0.000000000000000000 ) ) ;
#42363=CARTESIAN_POINT ( 'NONE',  ( -19.50000000000000000, -11.50000000000000000, 29.75000000000000355 ) ) ;
#42406=VERTEX_POINT ( 'NONE', #832 ) ;
#42409=AXIS2_PLACEMENT_3D ( 'NONE', #53965, #73809, #11205 ) ;
#42414=AXIS2_PLACEMENT_3D ( 'NONE', #33800, #12648, #52729 ) ;
#42415=ORIENTED_EDGE ( 'NONE', *, *, #41094, .F. ) ;
#42416=PLANE ( 'NONE',  #19860 ) ;
#42446=ORIENTED_EDGE ( 'NONE', *, *, #13527, .F. ) ;
#42461=CARTESIAN_POINT ( 'NONE',  ( 15.12820512820512953, -7.500000000000000000, 29.75000000000000355 ) ) ;
#42478=LINE ( 'NONE', #50098, #39484 ) ;
#42480=ORIENTED_EDGE ( 'NONE', *, *, #69845, .F. ) ;
#42486=LINE ( 'NONE', #56436, #51323 ) ;
#42489=CARTESIAN_POINT ( 'NONE',  ( -7.134615384615385025, -3.499999999999999556, 29.75000000000000355 ) ) ;
#42507=DIRECTION ( 'NONE',  ( -1.000000000000000000, 0.000000000000000000, -0.000000000000000000 ) ) ;
#42521=LINE ( 'NONE', #64531, #63313 ) ;
#42527=DIRECTION ( 'NONE',  ( 0.000000000000000000, 0.000000000000000000, -1.000000000000000000 ) ) ;
#42531=VERTEX_POINT ( 'NONE', #3029 ) ;
#42533=PLANE ( 'NONE',  #21162 ) ;
#42546=CARTESIAN_POINT ( 'NONE',  ( 1.576923076923075762, -7.500000000000000000, 33.75000000000000000 ) ) ;
#42556=EDGE_LOOP ( 'NONE', ( #26463, #16644, #55534, #38212 ) ) ;
#42568=EDGE_CURVE ( 'NONE', #56977, #7644, #32300, .T. ) ;
#42569=LINE ( 'NONE', #22289, #3099 ) ;
#42575=DIRECTION ( 'NONE',  ( -1.000000000000000000, -0.000000000000000000, 0.000000000000000000 ) ) ;
#42608=DIRECTION ( 'NONE',  ( -1.000000000000000000, -0.000000000000000000, -0.000000000000000000 ) ) ;
#42628=VECTOR ( 'NONE', #66440, 1000.000000000000000 ) ;
#42632=ORIENTED_EDGE ( 'NONE', *, *, #76266, .T. ) ;
#42659=ADVANCED_FACE ( 'NONE', ( #62410 ), #61529, .T. ) ;
#42670=ORIENTED_EDGE ( 'NONE', *, *, #41041, .T. ) ;
#42676=DIRECTION ( 'NONE',  ( -1.000000000000000000, -0.000000000000000000, -0.000000000000000000 ) ) ;
#42679=DIRECTION ( 'NONE',  ( -1.000000000000000000, -0.000000000000000000, -0.000000000000000000 ) ) ;
#42686=ADVANCED_FACE ( 'NONE', ( #20985 ), #41278, .F. ) ;
#42691=DIRECTION ( 'NONE',  ( -0.000000000000000000, 1.000000000000000000, -0.000000000000000000 ) ) ;
#42693=DIRECTION ( 'NONE',  ( -1.000000000000000000, -0.000000000000000000, -0.000000000000000000 ) ) ;
#42717=CIRCLE ( 'NONE', #45595, 4.000000000000000000 ) ;
#42726=EDGE_CURVE ( 'NONE', #48943, #55647, #35851, .T. ) ;
#42735=EDGE_CURVE ( 'NONE', #85269, #72492, #71390, .T. ) ;
#42736=VECTOR ( 'NONE', #54200, 1000.000000000000000 ) ;
#42739=CARTESIAN_POINT ( 'NONE',  ( -19.50000000000000000, -3.499999999999999556, 29.75000000000000355 ) ) ;
#42746=EDGE_LOOP ( 'NONE', ( #8326, #10491, #69452, #40955 ) ) ;
#42760=ORIENTED_EDGE ( 'NONE', *, *, #55353, .T. ) ;
#42779=LINE ( 'NONE', #3095, #82789 ) ;
#42805=FACE_OUTER_BOUND ( 'NONE', #59374, .T. ) ;
#42806=DIRECTION ( 'NONE',  ( -1.000000000000000000, -0.000000000000000000, 0.000000000000000000 ) ) ;
#42808=DIRECTION ( 'NONE',  ( 0.000000000000000000, 0.000000000000000000, -1.000000000000000000 ) ) ;
#42835=CARTESIAN_POINT ( 'NONE',  ( 14.87820512820512953, -7.500000000000000000, 29.75000000000000355 ) ) ;
#42839=ORIENTED_EDGE ( 'NONE', *, *, #60581, .T. ) ;
#42845=DIRECTION ( 'NONE',  ( -1.000000000000000000, -0.000000000000000000, -0.000000000000000000 ) ) ;
#42861=EDGE_CURVE ( 'NONE', #73366, #31226, #59663, .T. ) ;
#42863=CARTESIAN_POINT ( 'NONE',  ( 8.352564102564102200, -11.50000000000000000, 29.75000000000000355 ) ) ;
#42871=EDGE_CURVE ( 'NONE', #50717, #72564, #60550, .T. ) ;
#42876=AXIS2_PLACEMENT_3D ( 'NONE', #18624, #19063, #74013 ) ;
#42881=EDGE_CURVE ( 'NONE', #77088, #61773, #24989, .T. ) ;
#42888=FACE_OUTER_BOUND ( 'NONE', #6985, .T. ) ;
#42897=CARTESIAN_POINT ( 'NONE',  ( -19.50000000000000000, -3.499999999999999556, 29.75000000000000355 ) ) ;
#42908=CARTESIAN_POINT ( 'NONE',  ( 10.03846153846153832, -11.00000000000000000, 29.65000000000000213 ) ) ;
#42926=ORIENTED_EDGE ( 'NONE', *, *, #37835, .F. ) ;
#42939=PLANE ( 'NONE',  #76884 ) ;
#42941=AXIS2_PLACEMENT_3D ( 'NONE', #25513, #66946, #39041 ) ;
#42955=VECTOR ( 'NONE', #27059, 1000.000000000000000 ) ;
#42959=VERTEX_POINT ( 'NONE', #35294 ) ;
#42962=CARTESIAN_POINT ( 'NONE',  ( 19.00000000000000000, -7.500000000000000000, 29.75000000000000355 ) ) ;
#42971=VECTOR ( 'NONE', #38586, 1000.000000000000000 ) ;
#42990=ORIENTED_EDGE ( 'NONE', *, *, #29265, .F. ) ;
#43011=PLANE ( 'NONE',  #27736 ) ;
#43016=DIRECTION ( 'NONE',  ( 1.000000000000000000, 0.000000000000000000, 0.000000000000000000 ) ) ;
#43034=LINE ( 'NONE', #71829, #30586 ) ;
#43045=DIRECTION ( 'NONE',  ( 1.000000000000000000, 0.000000000000000000, 0.000000000000000000 ) ) ;
#43049=DIRECTION ( 'NONE',  ( 0.000000000000000000, 0.000000000000000000, -1.000000000000000000 ) ) ;
#43057=DIRECTION ( 'NONE',  ( 1.000000000000000000, 0.000000000000000000, 0.000000000000000000 ) ) ;
#43060=CARTESIAN_POINT ( 'NONE',  ( -0.3589743589743593088, -3.499999999999999556, 29.75000000000000355 ) ) ;
#43064=AXIS2_PLACEMENT_3D ( 'NONE', #62312, #81284, #19566 ) ;
#43080=ORIENTED_EDGE ( 'NONE', *, *, #88585, .F. ) ;
#43102=VERTEX_POINT ( 'NONE', #50126 ) ;
#43103=ADVANCED_FACE ( 'NONE', ( #9164 ), #84829, .T. ) ;
#43109=FACE_OUTER_BOUND ( 'NONE', #71499, .T. ) ;
#43111=DIRECTION ( 'NONE',  ( -1.000000000000000000, -0.000000000000000000, -0.000000000000000000 ) ) ;
#43118=EDGE_CURVE ( 'NONE', #42531, #15081, #43816, .T. ) ;
#43121=AXIS2_PLACEMENT_3D ( 'NONE', #36921, #72483, #38262 ) ;
#43124=VECTOR ( 'NONE', #87616, 1000.000000000000000 ) ;
#43126=CARTESIAN_POINT ( 'NONE',  ( -12.22435897435897267, -3.499999999999999556, 29.75000000000000355 ) ) ;
#43153=EDGE_CURVE ( 'NONE', #25462, #21400, #78047, .T. ) ;
#43170=DIRECTION ( 'NONE',  ( 1.000000000000000000, 0.000000000000000000, 0.000000000000000000 ) ) ;
#43172=DIRECTION ( 'NONE',  ( -1.000000000000000000, -0.000000000000000000, 0.000000000000000000 ) ) ;
#43180=AXIS2_PLACEMENT_3D ( 'NONE', #63307, #723, #28187 ) ;
#43188=AXIS2_PLACEMENT_3D ( 'NONE', #14637, #83102, #20062 ) ;
#43194=ORIENTED_EDGE ( 'NONE', *, *, #9819, .F. ) ;
#43213=FACE_OUTER_BOUND ( 'NONE', #56753, .T. ) ;
#43225=CARTESIAN_POINT ( 'NONE',  ( -7.134615384615385025, -4.000000000000000000, 29.75000000000000355 ) ) ;
#43236=CIRCLE ( 'NONE', #21694, 4.000000000000000000 ) ;
#43242=VECTOR ( 'NONE', #47641, 1000.000000000000000 ) ;
#43244=ORIENTED_EDGE ( 'NONE', *, *, #86968, .F. ) ;
#43264=DIRECTION ( 'NONE',  ( 0.000000000000000000, 0.000000000000000000, -1.000000000000000000 ) ) ;
#43292=CARTESIAN_POINT ( 'NONE',  ( -3.512820512820513663, -3.499999999999999556, 29.75000000000000355 ) ) ;
#43313=AXIS2_PLACEMENT_3D ( 'NONE', #82129, #48325, #68164 ) ;
#43327=ORIENTED_EDGE ( 'NONE', *, *, #26522, .T. ) ;
#43335=CARTESIAN_POINT ( 'NONE',  ( 1.576923076923075762, -11.50000000000000000, 29.75000000000000355 ) ) ;
#43343=AXIS2_PLACEMENT_3D ( 'NONE', #3701, #23970, #10477 ) ;
#43350=LINE ( 'NONE', #14546, #13259 ) ;
#43353=DIRECTION ( 'NONE',  ( 1.000000000000000000, 0.000000000000000000, 0.000000000000000000 ) ) ;
#43360=PLANE ( 'NONE',  #10797 ) ;
#43385=DIRECTION ( 'NONE',  ( 0.000000000000000000, 0.000000000000000000, -1.000000000000000000 ) ) ;
#43388=CARTESIAN_POINT ( 'NONE',  ( 11.25641025641025550, -3.499999999999999556, 29.75000000000000355 ) ) ;
#43390=EDGE_CURVE ( 'NONE', #47437, #20712, #64329, .T. ) ;
#43408=EDGE_LOOP ( 'NONE', ( #31278, #66746, #30871, #89025 ) ) ;
#43426=CARTESIAN_POINT ( 'NONE',  ( -12.94230769230769162, -7.500000000000000000, 33.75000000000000000 ) ) ;
#43428=VECTOR ( 'NONE', #49554, 1000.000000000000000 ) ;
#43430=VECTOR ( 'NONE', #6425, 1000.000000000000000 ) ;
#43452=CARTESIAN_POINT ( 'NONE',  ( -10.28846153846153832, -11.50000000000000000, 29.75000000000000355 ) ) ;
#43457=CYLINDRICAL_SURFACE ( 'NONE', #89063, 4.000000000000000000 ) ;
#43493=CARTESIAN_POINT ( 'NONE',  ( 15.84615384615384670, -3.499999999999999556, 29.75000000000000355 ) ) ;
#43499=VECTOR ( 'NONE', #28340, 1000.000000000000000 ) ;
#43510=ORIENTED_EDGE ( 'NONE', *, *, #65273, .F. ) ;
#43522=LINE ( 'NONE', #66464, #63231 ) ;
#43524=FACE_OUTER_BOUND ( 'NONE', #48613, .T. ) ;
#43530=EDGE_LOOP ( 'NONE', ( #71010, #57815, #5348, #73885 ) ) ;
#43532=ORIENTED_EDGE ( 'NONE', *, *, #50296, .T. ) ;
#43533=LINE ( 'NONE', #31812, #52188 ) ;
#43542=CARTESIAN_POINT ( 'NONE',  ( -19.50000000000000000, -11.50000000000000000, 29.75000000000000355 ) ) ;
#43556=LINE ( 'NONE', #36801, #12036 ) ;
#43566=CARTESIAN_POINT ( 'NONE',  ( -11.00641025641025550, -4.000000000000000000, 29.75000000000000355 ) ) ;
#43572=ADVANCED_FACE ( 'NONE', ( #23323 ), #50781, .F. ) ;
#43578=LINE ( 'NONE', #17445, #5461 ) ;
#43581=CARTESIAN_POINT ( 'NONE',  ( -19.50000000000000000, -3.499999999999999556, 29.75000000000000355 ) ) ;
#43582=AXIS2_PLACEMENT_3D ( 'NONE', #51438, #10495, #22669 ) ;
#43585=DIRECTION ( 'NONE',  ( 0.000000000000000000, 0.000000000000000000, -1.000000000000000000 ) ) ;
#43587=VECTOR ( 'NONE', #23698, 1000.000000000000000 ) ;
#43591=ORIENTED_EDGE ( 'NONE', *, *, #21788, .F. ) ;
#43607=ORIENTED_EDGE ( 'NONE', *, *, #33206, .F. ) ;
#43612=ORIENTED_EDGE ( 'NONE', *, *, #40067, .T. ) ;
#43618=ADVANCED_FACE ( 'NONE', ( #12054 ), #61108, .T. ) ;
#43622=CARTESIAN_POINT ( 'NONE',  ( 10.28846153846153832, -7.500000000000000000, 29.75000000000000355 ) ) ;
#43638=VECTOR ( 'NONE', #46523, 1000.000000000000000 ) ;
#43641=DIRECTION ( 'NONE',  ( 0.000000000000000000, 0.000000000000000000, -1.000000000000000000 ) ) ;
#43644=CARTESIAN_POINT ( 'NONE',  ( -19.50000000000000000, -3.499999999999999556, 29.75000000000000355 ) ) ;
#43680=CARTESIAN_POINT ( 'NONE',  ( -1.326923076923076872, -3.499999999999999556, 29.75000000000000355 ) ) ;
#43682=LINE ( 'NONE', #70724, #6379 ) ;
#43683=EDGE_CURVE ( 'NONE', #70465, #23070, #87724, .T. ) ;
#43695=EDGE_CURVE ( 'NONE', #65515, #50542, #74634, .T. ) ;
#43725=ORIENTED_EDGE ( 'NONE', *, *, #823, .T. ) ;
#43727=LINE ( 'NONE', #12176, #18843 ) ;
#43735=VERTEX_POINT ( 'NONE', #20566 ) ;
#43743=EDGE_CURVE ( 'NONE', #26475, #21434, #84545, .T. ) ;
#43749=VERTEX_POINT ( 'NONE', #13810 ) ;
#43759=DIRECTION ( 'NONE',  ( -1.000000000000000000, -0.000000000000000000, -0.000000000000000000 ) ) ;
#43796=VERTEX_POINT ( 'NONE', #49805 ) ;
#43803=DIRECTION ( 'NONE',  ( -0.000000000000000000, 0.000000000000000000, 1.000000000000000000 ) ) ;
#43806=VECTOR ( 'NONE', #40106, 1000.000000000000000 ) ;
#43808=LINE ( 'NONE', #71270, #75465 ) ;
#43815=DIRECTION ( 'NONE',  ( -0.000000000000000000, 1.000000000000000000, -0.000000000000000000 ) ) ;
#43816=LINE ( 'NONE', #71724, #8298 ) ;
#43826=ORIENTED_EDGE ( 'NONE', *, *, #70345, .F. ) ;
#43829=ORIENTED_EDGE ( 'NONE', *, *, #29929, .F. ) ;
#43832=DIRECTION ( 'NONE',  ( -1.000000000000000000, -0.000000000000000000, -0.000000000000000000 ) ) ;
#43835=EDGE_CURVE ( 'NONE', #74179, #37853, #23663, .T. ) ;
#43836=CARTESIAN_POINT ( 'NONE',  ( 19.00000000000000000, -3.499999999999999556, 29.75000000000000355 ) ) ;
#43846=ADVANCED_FACE ( 'NONE', ( #58331 ), #16913, .F. ) ;
#43857=DIRECTION ( 'NONE',  ( -0.000000000000000000, 1.000000000000000000, -0.000000000000000000 ) ) ;
#43861=AXIS2_PLACEMENT_3D ( 'NONE', #75267, #11794, #66729 ) ;
#43867=AXIS2_PLACEMENT_3D ( 'NONE', #8199, #35673, #64005 ) ;
#43901=CARTESIAN_POINT ( 'NONE',  ( 9.320512820512821150, -11.00000000000000000, 29.65000000000000213 ) ) ;
#43920=CARTESIAN_POINT ( 'NONE',  ( 17.06410256410256565, -11.50000000000000000, 29.75000000000000355 ) ) ;
#43927=DIRECTION ( 'NONE',  ( -1.000000000000000000, 0.000000000000000000, -0.000000000000000000 ) ) ;
#43930=VECTOR ( 'NONE', #48435, 1000.000000000000000 ) ;
#43936=ORIENTED_EDGE ( 'NONE', *, *, #36201, .F. ) ;
#43955=ORIENTED_EDGE ( 'NONE', *, *, #72534, .F. ) ;
#43956=EDGE_CURVE ( 'NONE', #20735, #87881, #33094, .T. ) ;
#44029=CARTESIAN_POINT ( 'NONE',  ( -4.230769230769230838, -7.500000000000000000, 33.75000000000000000 ) ) ;
#44053=ORIENTED_EDGE ( 'NONE', *, *, #7105, .F. ) ;
#44058=AXIS2_PLACEMENT_3D ( 'NONE', #54015, #81509, #32422 ) ;
#44067=CARTESIAN_POINT ( 'NONE',  ( -2.294871794871794712, -7.500000000000000000, 29.75000000000000355 ) ) ;
#44082=DIRECTION ( 'NONE',  ( 0.000000000000000000, 0.000000000000000000, -1.000000000000000000 ) ) ;
#44094=EDGE_LOOP ( 'NONE', ( #4889, #12567, #86237, #62724, #53890 ) ) ;
#44100=LINE ( 'NONE', #71579, #65462 ) ;
#44103=ORIENTED_EDGE ( 'NONE', *, *, #3332, .T. ) ;
#44114=DIRECTION ( 'NONE',  ( -1.000000000000000000, -0.000000000000000000, -0.000000000000000000 ) ) ;
#44128=DIRECTION ( 'NONE',  ( 1.000000000000000000, 0.000000000000000000, 0.000000000000000000 ) ) ;
#44163=DIRECTION ( 'NONE',  ( -1.000000000000000000, -0.000000000000000000, 0.000000000000000000 ) ) ;
#44167=DIRECTION ( 'NONE',  ( -1.000000000000000000, -0.000000000000000000, -0.000000000000000000 ) ) ;
#44170=ORIENTED_EDGE ( 'NONE', *, *, #61909, .T. ) ;
#44173=ORIENTED_EDGE ( 'NONE', *, *, #41874, .F. ) ;
#44179=ORIENTED_EDGE ( 'NONE', *, *, #1970, .F. ) ;
#44183=DIRECTION ( 'NONE',  ( -1.000000000000000000, 0.000000000000000000, -0.000000000000000000 ) ) ;
#44198=AXIS2_PLACEMENT_3D ( 'NONE', #32317, #73760, #59779 ) ;
#44209=EDGE_CURVE ( 'NONE', #66098, #33822, #60009, .T. ) ;
#44217=EDGE_LOOP ( 'NONE', ( #50515, #23533, #780, #30170, #55794, #13705, #5559, #26927, #16261, #52962, #46280, #72749, #61289, #18394, #46003, #56492, #26856, #25925, #23946, #17656, #64761, #66765, #38319, #55463, #39118, #66391, #7026, #16484, #25999, #7690, #72770, #77230, #66773, #79487, #87290, #14292, #26704, #56605, #59238, #28974, #54908, #8768, #14063, #86579, #24691, #48486, #86198, #31439, #44934, #68133, #81459, #12637, #80552, #2125, #64389, #62491, #63042, #12675, #48548, #3128, #68001, #32272, #51668, #59393, #17622, #65260, #27849, #76267, #12080, #8299, #37991, #28037, #28356, #87551, #51407, #10475, #56268, #32658, #44231, #13575, #55166, #83214, #77309, #17493, #73992, #42446, #66961, #54655, #14302, #88299, #31438, #67339, #85774, #17595, #85016 ) ) ;
#44231=ORIENTED_EDGE ( 'NONE', *, *, #88396, .F. ) ;
#44251=ORIENTED_EDGE ( 'NONE', *, *, #37683, .T. ) ;
#44264=PLANE ( 'NONE',  #85407 ) ;
#44273=ADVANCED_FACE ( 'NONE', ( #52802 ), #67223, .F. ) ;
#44276=CIRCLE ( 'NONE', #81670, 4.000000000000000000 ) ;
#44289=ORIENTED_EDGE ( 'NONE', *, *, #52601, .F. ) ;
#44291=CARTESIAN_POINT ( 'NONE',  ( 0.6089743589743582541, -3.499999999999999556, 29.75000000000000355 ) ) ;
#44295=CARTESIAN_POINT ( 'NONE',  ( -10.28846153846153832, -7.500000000000000000, 29.75000000000000355 ) ) ;
#44296=DIRECTION ( 'NONE',  ( -0.000000000000000000, 1.000000000000000000, -0.000000000000000000 ) ) ;
#44302=ORIENTED_EDGE ( 'NONE', *, *, #56829, .T. ) ;
#44317=AXIS2_PLACEMENT_3D ( 'NONE', #22788, #48491, #21915 ) ;
#44319=DIRECTION ( 'NONE',  ( 1.000000000000000000, 0.000000000000000000, 0.000000000000000000 ) ) ;
#44335=ADVANCED_FACE ( 'NONE', ( #33867 ), #42416, .F. ) ;
#44345=ORIENTED_EDGE ( 'NONE', *, *, #25056, .T. ) ;
#44361=EDGE_CURVE ( 'NONE', #32571, #22055, #62224, .T. ) ;
#44364=DIRECTION ( 'NONE',  ( 0.000000000000000000, 0.000000000000000000, -1.000000000000000000 ) ) ;
#44367=DIRECTION ( 'NONE',  ( -1.000000000000000000, -0.000000000000000000, -0.000000000000000000 ) ) ;
#44371=EDGE_CURVE ( 'NONE', #66098, #27341, #88840, .T. ) ;
#44382=ADVANCED_FACE ( 'NONE', ( #14041 ), #82072, .F. ) ;
#44388=VECTOR ( 'NONE', #32273, 1000.000000000000000 ) ;
#44391=DIRECTION ( 'NONE',  ( 0.000000000000000000, 0.000000000000000000, -1.000000000000000000 ) ) ;
#44420=EDGE_CURVE ( 'NONE', #5961, #7880, #20798, .T. ) ;
#44464=ADVANCED_FACE ( 'NONE', ( #65324 ), #85165, .F. ) ;
#44472=ORIENTED_EDGE ( 'NONE', *, *, #4103, .T. ) ;
#44474=EDGE_CURVE ( 'NONE', #11720, #57615, #1856, .T. ) ;
#44486=ORIENTED_EDGE ( 'NONE', *, *, #26751, .T. ) ;
#44492=EDGE_CURVE ( 'NONE', #35283, #35014, #64425, .T. ) ;
#44505=VERTEX_POINT ( 'NONE', #30651 ) ;
#44513=FACE_OUTER_BOUND ( 'NONE', #50624, .T. ) ;
#44538=VERTEX_POINT ( 'NONE', #46835 ) ;
#44543=CARTESIAN_POINT ( 'NONE',  ( -19.50000000000000000, -3.499999999999999556, 29.75000000000000355 ) ) ;
#44569=ORIENTED_EDGE ( 'NONE', *, *, #25797, .F. ) ;
#44574=VECTOR ( 'NONE', #23193, 1000.000000000000000 ) ;
#44575=VECTOR ( 'NONE', #60499, 1000.000000000000000 ) ;
#44586=ORIENTED_EDGE ( 'NONE', *, *, #75699, .T. ) ;
#44592=CARTESIAN_POINT ( 'NONE',  ( 1.576923076923075762, -3.499999999999999556, 29.75000000000000355 ) ) ;
#44616=EDGE_LOOP ( 'NONE', ( #84196, #28706, #26136, #85044 ) ) ;
#44633=DIRECTION ( 'NONE',  ( -1.000000000000000000, -0.000000000000000000, -0.000000000000000000 ) ) ;
#44640=COLOUR_RGB ( '', 0.72549020, 0.75294118, 0.79215686) ;
#44650=ORIENTED_EDGE ( 'NONE', *, *, #7715, .F. ) ;
#44669=ADVANCED_FACE ( 'NONE', ( #74315 ), #59013, .F. ) ;
#44673=FACE_OUTER_BOUND ( 'NONE', #87649, .T. ) ;
#44677=ORIENTED_EDGE ( 'NONE', *, *, #85121, .F. ) ;
#44680=DIRECTION ( 'NONE',  ( -1.000000000000000000, -0.000000000000000000, 0.000000000000000000 ) ) ;
#44691=DIRECTION ( 'NONE',  ( -1.000000000000000000, -0.000000000000000000, -0.000000000000000000 ) ) ;
#44694=CARTESIAN_POINT ( 'NONE',  ( -4.230769230769230838, -3.499999999999999556, 29.75000000000000355 ) ) ;
#44699=ORIENTED_EDGE ( 'NONE', *, *, #72434, .F. ) ;
#44702=VECTOR ( 'NONE', #27947, 1000.000000000000000 ) ;
#44710=AXIS2_PLACEMENT_3D ( 'NONE', #59625, #11004, #38476 ) ;
#44719=ORIENTED_EDGE ( 'NONE', *, *, #43153, .T. ) ;
#44728=VERTEX_POINT ( 'NONE', #82853 ) ;
#44729=ORIENTED_EDGE ( 'NONE', *, *, #36223, .T. ) ;
#44736=AXIS2_PLACEMENT_3D ( 'NONE', #80385, #60091, #65956 ) ;
#44740=CARTESIAN_POINT ( 'NONE',  ( -1.576923076923076428, -4.000000000000000000, 29.75000000000000355 ) ) ;
#44744=DIRECTION ( 'NONE',  ( 1.000000000000000000, 0.000000000000000000, 0.000000000000000000 ) ) ;
#44746=EDGE_LOOP ( 'NONE', ( #76592, #73336, #29472, #71779, #32766 ) ) ;
#44779=LINE ( 'NONE', #3356, #14129 ) ;
#44811=AXIS2_PLACEMENT_3D ( 'NONE', #81176, #87503, #87960 ) ;
#44827=EDGE_CURVE ( 'NONE', #14132, #87104, #30435, .T. ) ;
#44833=EDGE_CURVE ( 'NONE', #34232, #11498, #71410, .T. ) ;
#44837=ORIENTED_EDGE ( 'NONE', *, *, #32354, .T. ) ;
#44846=EDGE_CURVE ( 'NONE', #67618, #67129, #5631, .T. ) ;
#44850=ORIENTED_EDGE ( 'NONE', *, *, #3712, .F. ) ;
#44854=ORIENTED_EDGE ( 'NONE', *, *, #42303, .F. ) ;
#44855=CARTESIAN_POINT ( 'NONE',  ( 6.416666666666664298, -11.50000000000000000, 29.75000000000000355 ) ) ;
#44858=VECTOR ( 'NONE', #52860, 1000.000000000000000 ) ;
#44860=CARTESIAN_POINT ( 'NONE',  ( 10.28846153846153832, -3.499999999999999556, 29.75000000000000355 ) ) ;
#44875=PLANE ( 'NONE',  #39264 ) ;
#44882=DIRECTION ( 'NONE',  ( 0.000000000000000000, 0.000000000000000000, -1.000000000000000000 ) ) ;
#44898=DIRECTION ( 'NONE',  ( 0.000000000000000000, 0.000000000000000000, 1.000000000000000000 ) ) ;
#44900=CARTESIAN_POINT ( 'NONE',  ( 0.000000000000000000, -11.00000000000000000, 29.75000000000000355 ) ) ;
#44903=EDGE_CURVE ( 'NONE', #48041, #61963, #2616, .T. ) ;
#44934=ORIENTED_EDGE ( 'NONE', *, *, #16294, .F. ) ;
#44951=DIRECTION ( 'NONE',  ( -1.000000000000000000, -0.000000000000000000, -0.000000000000000000 ) ) ;
#44972=LINE ( 'NONE', #16618, #26016 ) ;
#44991=DIRECTION ( 'NONE',  ( 1.000000000000000000, 0.000000000000000000, 0.000000000000000000 ) ) ;
#45006=CARTESIAN_POINT ( 'NONE',  ( 3.262820512820511443, -4.000000000000000000, 29.75000000000000355 ) ) ;
#45027=CIRCLE ( 'NONE', #68065, 4.000000000000000000 ) ;
#45036=DIRECTION ( 'NONE',  ( 0.000000000000000000, 0.000000000000000000, -1.000000000000000000 ) ) ;
#45042=DIRECTION ( 'NONE',  ( 1.000000000000000000, 0.000000000000000000, 0.000000000000000000 ) ) ;
#45062=VERTEX_POINT ( 'NONE', #64541 ) ;
#45065=ORIENTED_EDGE ( 'NONE', *, *, #20037, .T. ) ;
#45069=ORIENTED_EDGE ( 'NONE', *, *, #32069, .F. ) ;
#45079=CARTESIAN_POINT ( 'NONE',  ( -18.03205128205128105, -3.499999999999999556, 29.75000000000000355 ) ) ;
#45089=ORIENTED_EDGE ( 'NONE', *, *, #50557, .F. ) ;
#45118=DIRECTION ( 'NONE',  ( -0.000000000000000000, 1.000000000000000000, -0.000000000000000000 ) ) ;
#45119=DIRECTION ( 'NONE',  ( 1.000000000000000000, 0.000000000000000000, 0.000000000000000000 ) ) ;
#45120=VECTOR ( 'NONE', #85652, 1000.000000000000000 ) ;
#45136=CYLINDRICAL_SURFACE ( 'NONE', #4517, 4.000000000000000000 ) ;
#45140=CARTESIAN_POINT ( 'NONE',  ( -19.00000000000000000, -3.499999999999999556, 29.75000000000000355 ) ) ;
#45150=AXIS2_PLACEMENT_3D ( 'NONE', #66005, #11976, #32673 ) ;
#45155=VECTOR ( 'NONE', #85281, 1000.000000000000000 ) ;
#45166=LINE ( 'NONE', #65443, #10959 ) ;
#45168=VERTEX_POINT ( 'NONE', #45618 ) ;
#45188=CARTESIAN_POINT ( 'NONE',  ( 1.576923076923075762, -3.499999999999999556, 29.75000000000000355 ) ) ;
#45216=FACE_OUTER_BOUND ( 'NONE', #74365, .T. ) ;
#45217=FACE_OUTER_BOUND ( 'NONE', #37188, .T. ) ;
#45222=VERTEX_POINT ( 'NONE', #80758 ) ;
#45225=CARTESIAN_POINT ( 'NONE',  ( -19.50000000000000000, -3.499999999999999556, 29.75000000000000355 ) ) ;
#45232=EDGE_CURVE ( 'NONE', #50514, #79802, #5082, .T. ) ;
#45241=EDGE_CURVE ( 'NONE', #21562, #22635, #18155, .T. ) ;
#45266=DIRECTION ( 'NONE',  ( -1.000000000000000000, 0.000000000000000000, -0.000000000000000000 ) ) ;
#45275=EDGE_LOOP ( 'NONE', ( #15825, #3519, #32049, #50705 ) ) ;
#45279=DIRECTION ( 'NONE',  ( 0.000000000000000000, 0.000000000000000000, -1.000000000000000000 ) ) ;
#45285=ORIENTED_EDGE ( 'NONE', *, *, #42871, .T. ) ;
#45288=DIRECTION ( 'NONE',  ( -1.000000000000000000, -0.000000000000000000, 0.000000000000000000 ) ) ;
#45319=ORIENTED_EDGE ( 'NONE', *, *, #32259, .F. ) ;
#45345=LINE ( 'NONE', #81374, #58920 ) ;
#45356=CARTESIAN_POINT ( 'NONE',  ( 0.3589743589743582541, -7.500000000000000000, 33.75000000000000000 ) ) ;
#45368=DIRECTION ( 'NONE',  ( 0.000000000000000000, 0.000000000000000000, -1.000000000000000000 ) ) ;
#45378=ADVANCED_FACE ( 'NONE', ( #4566 ), #66262, .F. ) ;
#45383=ADVANCED_FACE ( 'NONE', ( #86558 ), #24828, .F. ) ;
#45384=VERTEX_POINT ( 'NONE', #73027 ) ;
#45385=EDGE_CURVE ( 'NONE', #51674, #30978, #38803, .T. ) ;
#45397=DIRECTION ( 'NONE',  ( -0.000000000000000000, -0.000000000000000000, 1.000000000000000000 ) ) ;
#45403=ORIENTED_EDGE ( 'NONE', *, *, #51180, .F. ) ;
#45406=DIRECTION ( 'NONE',  ( 0.000000000000000000, 0.000000000000000000, -1.000000000000000000 ) ) ;
#45409=CARTESIAN_POINT ( 'NONE',  ( -7.134615384615385025, -7.500000000000000000, 29.75000000000000355 ) ) ;
#45416=DIRECTION ( 'NONE',  ( -1.000000000000000000, 0.000000000000000000, -0.000000000000000000 ) ) ;
#45424=ORIENTED_EDGE ( 'NONE', *, *, #83655, .T. ) ;
#45425=DIRECTION ( 'NONE',  ( 1.000000000000000000, 0.000000000000000000, 0.000000000000000000 ) ) ;
#45428=EDGE_LOOP ( 'NONE', ( #20233, #32018, #21144, #51147, #30654 ) ) ;
#45439=EDGE_CURVE ( 'NONE', #67446, #427, #5015, .T. ) ;
#45447=EDGE_CURVE ( 'NONE', #40122, #46874, #74574, .T. ) ;
#45451=EDGE_CURVE ( 'NONE', #78478, #34673, #26615, .T. ) ;
#45474=CARTESIAN_POINT ( 'NONE',  ( -7.384615384615385025, -7.500000000000000000, 29.75000000000000355 ) ) ;
#45486=ORIENTED_EDGE ( 'NONE', *, *, #67606, .F. ) ;
#45488=ORIENTED_EDGE ( 'NONE', *, *, #58420, .F. ) ;
#45490=EDGE_CURVE ( 'NONE', #72293, #21038, #45989, .T. ) ;
#45497=EDGE_CURVE ( 'NONE', #34333, #17369, #73923, .T. ) ;
#45517=ORIENTED_EDGE ( 'NONE', *, *, #38447, .T. ) ;
#45546=CARTESIAN_POINT ( 'NONE',  ( -11.00641025641025550, -7.500000000000000000, 29.75000000000000355 ) ) ;
#45547=DIRECTION ( 'NONE',  ( -1.000000000000000000, 0.000000000000000000, -0.000000000000000000 ) ) ;
#45566=CIRCLE ( 'NONE', #85880, 4.000000000000000000 ) ;
#45577=AXIS2_PLACEMENT_3D ( 'NONE', #77382, #15692, #8935 ) ;
#45589=DIRECTION ( 'NONE',  ( -1.000000000000000000, -0.000000000000000000, -0.000000000000000000 ) ) ;
#45595=AXIS2_PLACEMENT_3D ( 'NONE', #27881, #8502, #15702 ) ;
#45603=ORIENTED_EDGE ( 'NONE', *, *, #30030, .F. ) ;
#45618=CARTESIAN_POINT ( 'NONE',  ( 3.512820512820511443, -11.50000000000000000, 29.75000000000000355 ) ) ;
#45632=ADVANCED_FACE ( 'NONE', ( #38688 ), #85991, .T. ) ;
#45654=LINE ( 'NONE', #38012, #51837 ) ;
#45671=CARTESIAN_POINT ( 'NONE',  ( 10.03846153846153832, -4.000000000000000000, 29.25000000000000000 ) ) ;
#45672=DIRECTION ( 'NONE',  ( 0.000000000000000000, 0.000000000000000000, 1.000000000000000000 ) ) ;
#45684=CARTESIAN_POINT ( 'NONE',  ( 15.12820512820512953, -7.500000000000000000, 29.75000000000000355 ) ) ;
#45694=VECTOR ( 'NONE', #82122, 1000.000000000000000 ) ;
#45706=DIRECTION ( 'NONE',  ( -1.000000000000000000, -0.000000000000000000, -0.000000000000000000 ) ) ;
#45715=ORIENTED_EDGE ( 'NONE', *, *, #63569, .F. ) ;
#45744=DIRECTION ( 'NONE',  ( -1.000000000000000000, -0.000000000000000000, -0.000000000000000000 ) ) ;
#45765=LINE ( 'NONE', #52513, #85943 ) ;
#45766=CARTESIAN_POINT ( 'NONE',  ( -19.50000000000000000, -3.499999999999999556, 29.75000000000000355 ) ) ;
#45776=CARTESIAN_POINT ( 'NONE',  ( -9.320512820512821150, -3.499999999999999556, 29.75000000000000355 ) ) ;
#45778=DIRECTION ( 'NONE',  ( -1.000000000000000000, 0.000000000000000000, -0.000000000000000000 ) ) ;
#45793=DIRECTION ( 'NONE',  ( -0.000000000000000000, 1.000000000000000000, -0.000000000000000000 ) ) ;
#45812=EDGE_CURVE ( 'NONE', #20712, #77757, #54412, .T. ) ;
#45831=ORIENTED_EDGE ( 'NONE', *, *, #64306, .T. ) ;
#45839=CARTESIAN_POINT ( 'NONE',  ( 20.00000000000000000, -4.000000000000000000, 29.75000000000000355 ) ) ;
#45840=EDGE_CURVE ( 'NONE', #64311, #53642, #15655, .T. ) ;
#45847=AXIS2_PLACEMENT_3D ( 'NONE', #3118, #65261, #3563 ) ;
#45877=VECTOR ( 'NONE', #37662, 1000.000000000000000 ) ;
#45885=ADVANCED_FACE ( 'NONE', ( #62929 ), #28730, .T. ) ;
#45886=DIRECTION ( 'NONE',  ( -1.000000000000000000, 0.000000000000000000, -0.000000000000000000 ) ) ;
#45898=DIRECTION ( 'NONE',  ( -0.000000000000000000, 1.000000000000000000, -0.000000000000000000 ) ) ;
#45903=EDGE_CURVE ( 'NONE', #82221, #31128, #77348, .T. ) ;
#45921=DIRECTION ( 'NONE',  ( 1.000000000000000000, 0.000000000000000000, 0.000000000000000000 ) ) ;
#45924=EDGE_LOOP ( 'NONE', ( #50423, #69756, #32492, #19057, #71145 ) ) ;
#45939=ORIENTED_EDGE ( 'NONE', *, *, #15646, .T. ) ;
#45947=CARTESIAN_POINT ( 'NONE',  ( -7.134615384615385025, -3.499999999999999556, 29.75000000000000355 ) ) ;
#45948=VECTOR ( 'NONE', #63145, 1000.000000000000000 ) ;
#45949=CIRCLE ( 'NONE', #2796, 4.000000000000000000 ) ;
#45953=VERTEX_POINT ( 'NONE', #29615 ) ;
#45969=EDGE_CURVE ( 'NONE', #40626, #51674, #85437, .T. ) ;
#45974=FACE_OUTER_BOUND ( 'NONE', #22795, .T. ) ;
#45980=ORIENTED_EDGE ( 'NONE', *, *, #1553, .T. ) ;
#45989=LINE ( 'NONE', #41021, #86082 ) ;
#45998=ORIENTED_EDGE ( 'NONE', *, *, #15028, .T. ) ;
#46001=CIRCLE ( 'NONE', #87758, 4.000000000000000000 ) ;
#46003=ORIENTED_EDGE ( 'NONE', *, *, #82932, .F. ) ;
#46005=CARTESIAN_POINT ( 'NONE',  ( -11.25641025641025550, -11.00000000000000000, 29.75000000000000355 ) ) ;
#46011=DIRECTION ( 'NONE',  ( -1.000000000000000000, -0.000000000000000000, -0.000000000000000000 ) ) ;
#46012=VECTOR ( 'NONE', #87486, 1000.000000000000000 ) ;
#46018=CYLINDRICAL_SURFACE ( 'NONE', #26610, 4.000000000000000000 ) ;
#46020=CARTESIAN_POINT ( 'NONE',  ( -19.50000000000000000, -3.499999999999999556, 29.75000000000000355 ) ) ;
#46024=CYLINDRICAL_SURFACE ( 'NONE', #58136, 4.000000000000000000 ) ;
#46032=LINE ( 'NONE', #17680, #695 ) ;
#46033=EDGE_LOOP ( 'NONE', ( #12313, #62524, #75968, #53497 ) ) ;
#46037=EDGE_CURVE ( 'NONE', #60033, #80094, #19200, .T. ) ;
#46041=LINE ( 'NONE', #17691, #10582 ) ;
#46042=VERTEX_POINT ( 'NONE', #45776 ) ;
#46072=FACE_OUTER_BOUND ( 'NONE', #75291, .T. ) ;
#46076=LINE ( 'NONE', #38885, #43638 ) ;
#46082=ADVANCED_FACE ( 'NONE', ( #33154 ), #26843, .T. ) ;
#46086=ORIENTED_EDGE ( 'NONE', *, *, #79201, .T. ) ;
#46089=EDGE_CURVE ( 'NONE', #73852, #9873, #25950, .T. ) ;
#46090=CARTESIAN_POINT ( 'NONE',  ( -4.230769230769230838, -7.500000000000000000, 29.75000000000000355 ) ) ;
#46091=LINE ( 'NONE', #85156, #19257 ) ;
#46094=CARTESIAN_POINT ( 'NONE',  ( 20.00000000000000000, -7.500000000000000000, 33.75000000000000000 ) ) ;
#46108=VECTOR ( 'NONE', #71054, 1000.000000000000000 ) ;
#46114=CARTESIAN_POINT ( 'NONE',  ( 18.75000000000000000, -3.499999999999999556, 29.75000000000000355 ) ) ;
#46120=EDGE_LOOP ( 'NONE', ( #35762, #53011, #88354, #34569 ) ) ;
#46136=CARTESIAN_POINT ( 'NONE',  ( -12.22435897435897267, -3.499999999999999556, 29.75000000000000355 ) ) ;
#46140=AXIS2_PLACEMENT_3D ( 'NONE', #41810, #22846, #83690 ) ;
#46146=ORIENTED_EDGE ( 'NONE', *, *, #33556, .T. ) ;
#46149=ORIENTED_EDGE ( 'NONE', *, *, #61937, .T. ) ;
#46200=ORIENTED_EDGE ( 'NONE', *, *, #9062, .T. ) ;
#46216=DIRECTION ( 'NONE',  ( 1.000000000000000000, 0.000000000000000000, 0.000000000000000000 ) ) ;
#46218=FACE_OUTER_BOUND ( 'NONE', #78585, .T. ) ;
#46228=LINE ( 'NONE', #18314, #81423 ) ;
#46229=CARTESIAN_POINT ( 'NONE',  ( -19.50000000000000000, -11.50000000000000000, 29.75000000000000355 ) ) ;
#46272=DIRECTION ( 'NONE',  ( -1.000000000000000000, -0.000000000000000000, -0.000000000000000000 ) ) ;
#46280=ORIENTED_EDGE ( 'NONE', *, *, #3332, .F. ) ;
#46291=VECTOR ( 'NONE', #130, 1000.000000000000000 ) ;
#46296=CARTESIAN_POINT ( 'NONE',  ( -0.6089743589743593644, -7.500000000000000000, 33.75000000000000000 ) ) ;
#46309=CARTESIAN_POINT ( 'NONE',  ( 9.070512820512819374, -11.00000000000000000, 29.75000000000000355 ) ) ;
#46312=AXIS2_PLACEMENT_3D ( 'NONE', #42835, #1395, #82937 ) ;
#46329=CARTESIAN_POINT ( 'NONE',  ( 12.94230769230769340, -11.50000000000000000, 29.75000000000000355 ) ) ;
#46331=EDGE_LOOP ( 'NONE', ( #23231, #41211, #84247, #51069 ) ) ;
#46333=DIRECTION ( 'NONE',  ( 0.000000000000000000, 0.000000000000000000, -1.000000000000000000 ) ) ;
#46342=EDGE_CURVE ( 'NONE', #38566, #83848, #35809, .T. ) ;
#46344=SHAPE_REPRESENTATION_RELATIONSHIP ( 'NONE' , 'NONE' ,  #60984, #923 ) ;
#46347=EDGE_LOOP ( 'NONE', ( #12112, #47322, #72411, #50696, #32333 ) ) ;
#46360=DIRECTION ( 'NONE',  ( 0.000000000000000000, 0.000000000000000000, -1.000000000000000000 ) ) ;
#46361=CARTESIAN_POINT ( 'NONE',  ( 2.544871794871792936, -7.500000000000000000, 29.75000000000000355 ) ) ;
#46362=VECTOR ( 'NONE', #19528, 1000.000000000000000 ) ;
#46365=ADVANCED_FACE ( 'NONE', ( #79018 ), #43457, .T. ) ;
#46386=ORIENTED_EDGE ( 'NONE', *, *, #30271, .F. ) ;
#46392=ORIENTED_EDGE ( 'NONE', *, *, #2631, .T. ) ;
#46399=LINE ( 'NONE', #59468, #74984 ) ;
#46413=ORIENTED_EDGE ( 'NONE', *, *, #86511, .F. ) ;
#46426=DIRECTION ( 'NONE',  ( 0.000000000000000000, 0.000000000000000000, -1.000000000000000000 ) ) ;
#46433=ORIENTED_EDGE ( 'NONE', *, *, #25591, .T. ) ;
#46444=DIRECTION ( 'NONE',  ( 0.000000000000000000, 0.000000000000000000, -1.000000000000000000 ) ) ;
#46455=ORIENTED_EDGE ( 'NONE', *, *, #20111, .F. ) ;
#46473=DIRECTION ( 'NONE',  ( -1.000000000000000000, -0.000000000000000000, -0.000000000000000000 ) ) ;
#46484=VERTEX_POINT ( 'NONE', #49996 ) ;
#46489=FACE_OUTER_BOUND ( 'NONE', #34568, .T. ) ;
#46491=DIRECTION ( 'NONE',  ( 1.000000000000000000, 0.000000000000000000, 0.000000000000000000 ) ) ;
#46501=EDGE_CURVE ( 'NONE', #40626, #15955, #13235, .T. ) ;
#46509=EDGE_CURVE ( 'NONE', #48052, #50514, #4022, .T. ) ;
#46519=AXIS2_PLACEMENT_3D ( 'NONE', #43644, #57162, #64347 ) ;
#46523=DIRECTION ( 'NONE',  ( -1.000000000000000000, -0.000000000000000000, -0.000000000000000000 ) ) ;
#46528=ORIENTED_EDGE ( 'NONE', *, *, #76194, .T. ) ;
#46537=LINE ( 'NONE', #67697, #86910 ) ;
#46538=LINE ( 'NONE', #33025, #8851 ) ;
#46539=ORIENTED_EDGE ( 'NONE', *, *, #2904, .T. ) ;
#46552=CARTESIAN_POINT ( 'NONE',  ( 9.320512820512821150, -11.50000000000000000, 29.75000000000000355 ) ) ;
#46558=ORIENTED_EDGE ( 'NONE', *, *, #14850, .F. ) ;
#46561=DIRECTION ( 'NONE',  ( 1.000000000000000000, 0.000000000000000000, 0.000000000000000000 ) ) ;
#46566=ORIENTED_EDGE ( 'NONE', *, *, #12586, .F. ) ;
#46593=ORIENTED_EDGE ( 'NONE', *, *, #36677, .F. ) ;
#46608=LINE ( 'NONE', #73194, #50766 ) ;
#46609=EDGE_LOOP ( 'NONE', ( #19012, #10094, #12949, #6396, #37029 ) ) ;
#46631=ORIENTED_EDGE ( 'NONE', *, *, #76135, .F. ) ;
#46638=AXIS2_PLACEMENT_3D ( 'NONE', #27464, #49053, #83299 ) ;
#46642=ORIENTED_EDGE ( 'NONE', *, *, #43743, .F. ) ;
#46646=ORIENTED_EDGE ( 'NONE', *, *, #68789, .T. ) ;
#46661=CARTESIAN_POINT ( 'NONE',  ( -3.262820512820514107, -3.499999999999999556, 29.75000000000000355 ) ) ;
#46662=ORIENTED_EDGE ( 'NONE', *, *, #64306, .F. ) ;
#46665=ORIENTED_EDGE ( 'NONE', *, *, #80762, .T. ) ;
#46693=CARTESIAN_POINT ( 'NONE',  ( 0.000000000000000000, -11.00000000000000000, 29.75000000000000355 ) ) ;
#46694=DIRECTION ( 'NONE',  ( -1.000000000000000000, -0.000000000000000000, -0.000000000000000000 ) ) ;
#46695=DIRECTION ( 'NONE',  ( -1.000000000000000000, -0.000000000000000000, -0.000000000000000000 ) ) ;
#46712=DIRECTION ( 'NONE',  ( -1.000000000000000000, -0.000000000000000000, -0.000000000000000000 ) ) ;
#46733=CARTESIAN_POINT ( 'NONE',  ( 13.91025641025641235, -3.499999999999999556, 29.75000000000000355 ) ) ;
#46749=EDGE_LOOP ( 'NONE', ( #86331, #85618, #22147, #55278 ) ) ;
#46774=CARTESIAN_POINT ( 'NONE',  ( -11.97435897435897267, -3.499999999999999556, 29.75000000000000355 ) ) ;
#46798=LINE ( 'NONE', #47682, #36647 ) ;
#46823=ORIENTED_EDGE ( 'NONE', *, *, #43743, .T. ) ;
#46833=EDGE_CURVE ( 'NONE', #46874, #6628, #35950, .T. ) ;
#46835=CARTESIAN_POINT ( 'NONE',  ( 7.134615384615385025, -7.500000000000000000, 33.75000000000000000 ) ) ;
#46872=CARTESIAN_POINT ( 'NONE',  ( -8.102564102564102200, -11.50000000000000000, 29.75000000000000355 ) ) ;
#46874=VERTEX_POINT ( 'NONE', #83704 ) ;
#46881=ORIENTED_EDGE ( 'NONE', *, *, #18414, .T. ) ;
#46886=DIRECTION ( 'NONE',  ( 1.000000000000000000, 0.000000000000000000, 0.000000000000000000 ) ) ;
#46892=ORIENTED_EDGE ( 'NONE', *, *, #9810, .T. ) ;
#46896=CARTESIAN_POINT ( 'NONE',  ( -18.75000000000000000, -7.500000000000000000, 33.75000000000000000 ) ) ;
#46924=DIRECTION ( 'NONE',  ( -1.000000000000000000, -0.000000000000000000, -0.000000000000000000 ) ) ;
#46939=ORIENTED_EDGE ( 'NONE', *, *, #35665, .F. ) ;
#46944=CARTESIAN_POINT ( 'NONE',  ( 0.6089743589743582541, -7.500000000000000000, 29.75000000000000355 ) ) ;
#46953=VERTEX_POINT ( 'NONE', #10688 ) ;
#46962=EDGE_CURVE ( 'NONE', #57615, #59590, #43578, .T. ) ;
#46965=EDGE_CURVE ( 'NONE', #60579, #17730, #30940, .T. ) ;
#46968=ORIENTED_EDGE ( 'NONE', *, *, #68716, .T. ) ;
#46970=AXIS2_PLACEMENT_3D ( 'NONE', #62225, #41078, #34755 ) ;
#46976=CARTESIAN_POINT ( 'NONE',  ( -13.19230769230769162, -7.500000000000000000, 29.75000000000000355 ) ) ;
#47010=CARTESIAN_POINT ( 'NONE',  ( 15.12820512820512953, -3.499999999999999556, 29.75000000000000355 ) ) ;
#47014=VECTOR ( 'NONE', #75418, 1000.000000000000000 ) ;
#47041=FACE_OUTER_BOUND ( 'NONE', #75646, .T. ) ;
#47044=CARTESIAN_POINT ( 'NONE',  ( 0.000000000000000000, -11.00000000000000000, 29.75000000000000355 ) ) ;
#47057=DIRECTION ( 'NONE',  ( 0.000000000000000000, 0.000000000000000000, 1.000000000000000000 ) ) ;
#47060=AXIS2_PLACEMENT_3D ( 'NONE', #85105, #65697, #9008 ) ;
#47061=ORIENTED_EDGE ( 'NONE', *, *, #38780, .T. ) ;
#47074=ORIENTED_EDGE ( 'NONE', *, *, #60093, .F. ) ;
#47099=DIRECTION ( 'NONE',  ( -0.000000000000000000, 1.000000000000000000, -0.000000000000000000 ) ) ;
#47108=DIRECTION ( 'NONE',  ( 1.000000000000000000, 0.000000000000000000, 0.000000000000000000 ) ) ;
#47127=EDGE_CURVE ( 'NONE', #49729, #71435, #68709, .T. ) ;
#47161=ORIENTED_EDGE ( 'NONE', *, *, #69552, .F. ) ;
#47163=CIRCLE ( 'NONE', #14056, 4.000000000000000000 ) ;
#47172=ORIENTED_EDGE ( 'NONE', *, *, #56571, .F. ) ;
#47175=DIRECTION ( 'NONE',  ( 1.000000000000000000, 0.000000000000000000, 0.000000000000000000 ) ) ;
#47178=CARTESIAN_POINT ( 'NONE',  ( -19.50000000000000000, -3.499999999999999556, 29.75000000000000355 ) ) ;
#47195=VECTOR ( 'NONE', #5667, 1000.000000000000000 ) ;
#47209=SURFACE_STYLE_FILL_AREA ( #19746 ) ;
#47228=EDGE_LOOP ( 'NONE', ( #46939, #38348, #44345, #56276 ) ) ;
#47248=EDGE_CURVE ( 'NONE', #17957, #34265, #58678, .T. ) ;
#47272=VERTEX_POINT ( 'NONE', #1006 ) ;
#47273=AXIS2_PLACEMENT_3D ( 'NONE', #34042, #13328, #18764 ) ;
#47284=ORIENTED_EDGE ( 'NONE', *, *, #10844, .F. ) ;
#47299=VECTOR ( 'NONE', #26873, 1000.000000000000000 ) ;
#47307=PLANE ( 'NONE',  #57245 ) ;
#47311=LINE ( 'NONE', #40576, #62009 ) ;
#47322=ORIENTED_EDGE ( 'NONE', *, *, #55597, .T. ) ;
#47326=FACE_OUTER_BOUND ( 'NONE', #82583, .T. ) ;
#47341=DIRECTION ( 'NONE',  ( 0.000000000000000000, 0.000000000000000000, -1.000000000000000000 ) ) ;
#47356=CARTESIAN_POINT ( 'NONE',  ( -17.06410256410256565, -7.500000000000000000, 29.75000000000000355 ) ) ;
#47371=EDGE_CURVE ( 'NONE', #49175, #9891, #84322, .T. ) ;
#47376=CARTESIAN_POINT ( 'NONE',  ( 20.00000000000000000, -4.000000000000000000, 29.75000000000000355 ) ) ;
#47384=CARTESIAN_POINT ( 'NONE',  ( 5.448717948717947124, -3.499999999999999556, 29.75000000000000355 ) ) ;
#47396=ORIENTED_EDGE ( 'NONE', *, *, #9810, .F. ) ;
#47399=ORIENTED_EDGE ( 'NONE', *, *, #55807, .T. ) ;
#47412=CIRCLE ( 'NONE', #43121, 0.5000000000000004441 ) ;
#47420=CARTESIAN_POINT ( 'NONE',  ( -15.12820512820512953, -3.499999999999999556, 29.75000000000000355 ) ) ;
#47433=VERTEX_POINT ( 'NONE', #5419 ) ;
#47435=LINE ( 'NONE', #67723, #5900 ) ;
#47437=VERTEX_POINT ( 'NONE', #12620 ) ;
#47454=FACE_OUTER_BOUND ( 'NONE', #61055, .T. ) ;
#47467=DIRECTION ( 'NONE',  ( -0.000000000000000000, 1.000000000000000000, -0.000000000000000000 ) ) ;
#47481=VECTOR ( 'NONE', #22326, 1000.000000000000000 ) ;
#47503=CARTESIAN_POINT ( 'NONE',  ( 19.50000000000000000, -7.500000000000000000, 29.75000000000000355 ) ) ;
#47512=VECTOR ( 'NONE', #45921, 1000.000000000000000 ) ;
#47519=ADVANCED_FACE ( 'NONE', ( #62992 ), #9400, .T. ) ;
#47528=DIRECTION ( 'NONE',  ( 1.000000000000000000, 0.000000000000000000, 0.000000000000000000 ) ) ;
#47533=CARTESIAN_POINT ( 'NONE',  ( -19.50000000000000000, -3.499999999999999556, 29.75000000000000355 ) ) ;
#47534=CIRCLE ( 'NONE', #86467, 4.000000000000000000 ) ;
#47537=DIRECTION ( 'NONE',  ( 0.000000000000000000, 0.000000000000000000, 1.000000000000000000 ) ) ;
#47541=ADVANCED_FACE ( 'NONE', ( #2623 ), #1752, .F. ) ;
#47545=ORIENTED_EDGE ( 'NONE', *, *, #19058, .T. ) ;
#47546=VECTOR ( 'NONE', #1582, 1000.000000000000000 ) ;
#47562=CARTESIAN_POINT ( 'NONE',  ( 2.544871794871792936, -7.500000000000000000, 29.75000000000000355 ) ) ;
#47565=LINE ( 'NONE', #26859, #33443 ) ;
#47572=DIRECTION ( 'NONE',  ( 0.000000000000000000, 0.000000000000000000, -1.000000000000000000 ) ) ;
#47589=CARTESIAN_POINT ( 'NONE',  ( -1.326923076923076872, -3.499999999999999556, 29.75000000000000355 ) ) ;
#47597=LINE ( 'NONE', #67873, #83391 ) ;
#47607=CARTESIAN_POINT ( 'NONE',  ( 0.000000000000000000, -11.00000000000000000, 29.75000000000000355 ) ) ;
#47612=ORIENTED_EDGE ( 'NONE', *, *, #10951, .F. ) ;
#47614=VECTOR ( 'NONE', #32824, 1000.000000000000000 ) ;
#47616=CARTESIAN_POINT ( 'NONE',  ( 19.50000000000000000, -3.499999999999999556, 29.75000000000000355 ) ) ;
#47619=DIRECTION ( 'NONE',  ( 1.000000000000000000, 0.000000000000000000, 0.000000000000000000 ) ) ;
#47628=DIRECTION ( 'NONE',  ( 0.000000000000000000, 0.000000000000000000, 1.000000000000000000 ) ) ;
#47631=EDGE_CURVE ( 'NONE', #29384, #4984, #85065, .T. ) ;
#47632=DIRECTION ( 'NONE',  ( -1.000000000000000000, 0.000000000000000000, -0.000000000000000000 ) ) ;
#47635=LINE ( 'NONE', #60252, #33544 ) ;
#47641=DIRECTION ( 'NONE',  ( -1.000000000000000000, -0.000000000000000000, -0.000000000000000000 ) ) ;
#47670=DIRECTION ( 'NONE',  ( 0.000000000000000000, 0.000000000000000000, -1.000000000000000000 ) ) ;
#47673=CARTESIAN_POINT ( 'NONE',  ( 0.000000000000000000, -11.00000000000000000, 29.65000000000000213 ) ) ;
#47682=CARTESIAN_POINT ( 'NONE',  ( 0.000000000000000000, -11.00000000000000000, 29.75000000000000355 ) ) ;
#47713=VERTEX_POINT ( 'NONE', #47616 ) ;
#47758=LINE ( 'NONE', #40135, #50278 ) ;
#47763=EDGE_CURVE ( 'NONE', #955, #45222, #53028, .T. ) ;
#47805=LINE ( 'NONE', #88379, #46012 ) ;
#47807=EDGE_CURVE ( 'NONE', #88674, #44538, #52941, .T. ) ;
#47808=AXIS2_PLACEMENT_3D ( 'NONE', #70049, #2467, #15116 ) ;
#47813=DIRECTION ( 'NONE',  ( 1.000000000000000000, 0.000000000000000000, 0.000000000000000000 ) ) ;
#47841=EDGE_CURVE ( 'NONE', #75643, #12463, #756, .T. ) ;
#47848=VERTEX_POINT ( 'NONE', #36323 ) ;
#47850=ADVANCED_FACE ( 'NONE', ( #55691 ), #7072, .F. ) ;
#47854=VECTOR ( 'NONE', #56874, 1000.000000000000000 ) ;
#47858=DIRECTION ( 'NONE',  ( -1.000000000000000000, -0.000000000000000000, 0.000000000000000000 ) ) ;
#47870=LINE ( 'NONE', #74913, #64343 ) ;
#47877=LINE ( 'NONE', #42021, #76391 ) ;
#47879=ORIENTED_EDGE ( 'NONE', *, *, #70151, .T. ) ;
#47890=CARTESIAN_POINT ( 'NONE',  ( -20.00000000000000000, -11.50000000000000000, 28.25000000000000000 ) ) ;
#47903=LINE ( 'NONE', #42489, #73531 ) ;
#47960=DIRECTION ( 'NONE',  ( 0.000000000000000000, -1.000000000000000000, 0.000000000000000000 ) ) ;
#47968=FACE_OUTER_BOUND ( 'NONE', #83862, .T. ) ;
#47970=ADVANCED_FACE ( 'NONE', ( #12284 ), #32113, .F. ) ;
#47972=DIRECTION ( 'NONE',  ( 0.000000000000000000, 0.000000000000000000, -1.000000000000000000 ) ) ;
#47978=VECTOR ( 'NONE', #55061, 1000.000000000000000 ) ;
#48014=DIRECTION ( 'NONE',  ( -1.000000000000000000, -0.000000000000000000, 0.000000000000000000 ) ) ;
#48028=DIRECTION ( 'NONE',  ( -0.000000000000000000, 1.000000000000000000, -0.000000000000000000 ) ) ;
#48029=VERTEX_POINT ( 'NONE', #87985 ) ;
#48041=VERTEX_POINT ( 'NONE', #27129 ) ;
#48050=CARTESIAN_POINT ( 'NONE',  ( 1.576923076923075762, -7.500000000000000000, 29.75000000000000355 ) ) ;
#48052=VERTEX_POINT ( 'NONE', #62672 ) ;
#48058=DIRECTION ( 'NONE',  ( 0.000000000000000000, 0.000000000000000000, -1.000000000000000000 ) ) ;
#48059=CARTESIAN_POINT ( 'NONE',  ( -11.97435897435897267, -3.499999999999999556, 29.75000000000000355 ) ) ;
#48061=CARTESIAN_POINT ( 'NONE',  ( -13.19230769230769162, -3.499999999999999556, 29.75000000000000355 ) ) ;
#48069=CARTESIAN_POINT ( 'NONE',  ( 6.166666666666664298, -3.499999999999999556, 29.75000000000000355 ) ) ;
#48077=CARTESIAN_POINT ( 'NONE',  ( 14.16025641025641235, -7.500000000000000000, 29.75000000000000355 ) ) ;
#48078=CYLINDRICAL_SURFACE ( 'NONE', #35322, 4.000000000000000000 ) ;
#48086=EDGE_CURVE ( 'NONE', #44728, #73862, #63034, .T. ) ;
#48099=CIRCLE ( 'NONE', #17955, 4.000000000000000000 ) ;
#48110=AXIS2_PLACEMENT_3D ( 'NONE', #48050, #34546, #68335 ) ;
#48123=PLANE ( 'NONE',  #53074 ) ;
#48134=FACE_OUTER_BOUND ( 'NONE', #82850, .T. ) ;
#48136=EDGE_CURVE ( 'NONE', #29630, #32571, #54141, .T. ) ;
#48149=EDGE_LOOP ( 'NONE', ( #72976, #24579, #75015, #75221 ) ) ;
#48161=DIRECTION ( 'NONE',  ( 1.000000000000000000, -0.000000000000000000, 0.000000000000000000 ) ) ;
#48162=DIRECTION ( 'NONE',  ( 1.000000000000000000, 0.000000000000000000, 0.000000000000000000 ) ) ;
#48165=CARTESIAN_POINT ( 'NONE',  ( -20.00000000000000000, -3.499999999999999556, 28.25000000000000000 ) ) ;
#48183=ORIENTED_EDGE ( 'NONE', *, *, #88510, .T. ) ;
#48185=EDGE_CURVE ( 'NONE', #1012, #40626, #23027, .T. ) ;
#48204=ADVANCED_FACE ( 'NONE', ( #9084 ), #77972, .T. ) ;
#48209=ORIENTED_EDGE ( 'NONE', *, *, #32259, .T. ) ;
#48227=CARTESIAN_POINT ( 'NONE',  ( -17.78205128205128105, -3.499999999999999556, 29.75000000000000355 ) ) ;
#48230=PLANE ( 'NONE',  #58367 ) ;
#48233=CARTESIAN_POINT ( 'NONE',  ( -18.03205128205128105, -4.000000000000000000, 29.75000000000000355 ) ) ;
#48235=FACE_OUTER_BOUND ( 'NONE', #80325, .T. ) ;
#48246=VERTEX_POINT ( 'NONE', #3634 ) ;
#48263=CARTESIAN_POINT ( 'NONE',  ( 13.91025641025641235, -7.500000000000000000, 29.75000000000000355 ) ) ;
#48265=AXIS2_PLACEMENT_3D ( 'NONE', #39282, #39726, #80719 ) ;
#48267=LINE ( 'NONE', #8183, #13132 ) ;
#48277=EDGE_LOOP ( 'NONE', ( #619, #34556, #31909, #54620 ) ) ;
#48305=FACE_OUTER_BOUND ( 'NONE', #42023, .T. ) ;
#48311=CARTESIAN_POINT ( 'NONE',  ( 12.22435897435897623, -11.50000000000000000, 29.75000000000000355 ) ) ;
#48320=ORIENTED_EDGE ( 'NONE', *, *, #11768, .T. ) ;
#48323=CIRCLE ( 'NONE', #35409, 4.000000000000000000 ) ;
#48324=DIRECTION ( 'NONE',  ( 0.000000000000000000, 0.000000000000000000, -1.000000000000000000 ) ) ;
#48325=DIRECTION ( 'NONE',  ( 1.000000000000000000, 0.000000000000000000, 0.000000000000000000 ) ) ;
#48338=CARTESIAN_POINT ( 'NONE',  ( -19.00000000000000000, -3.499999999999999556, 29.75000000000000355 ) ) ;
#48364=VECTOR ( 'NONE', #24167, 1000.000000000000000 ) ;
#48373=DIRECTION ( 'NONE',  ( 0.000000000000000000, 0.000000000000000000, -1.000000000000000000 ) ) ;
#48378=ADVANCED_FACE ( 'NONE', ( #75220 ), #12630, .T. ) ;
#48402=CARTESIAN_POINT ( 'NONE',  ( 16.81410256410256565, -7.500000000000000000, 29.75000000000000355 ) ) ;
#48406=ORIENTED_EDGE ( 'NONE', *, *, #83652, .T. ) ;
#48416=VERTEX_POINT ( 'NONE', #13946 ) ;
#48421=DIRECTION ( 'NONE',  ( 1.000000000000000000, 0.000000000000000000, 0.000000000000000000 ) ) ;
#48431=CYLINDRICAL_SURFACE ( 'NONE', #64476, 4.000000000000000000 ) ;
#48435=DIRECTION ( 'NONE',  ( -1.000000000000000000, -0.000000000000000000, -0.000000000000000000 ) ) ;
#48447=VERTEX_POINT ( 'NONE', #13066 ) ;
#48455=AXIS2_PLACEMENT_3D ( 'NONE', #65503, #37583, #31281 ) ;
#48457=LINE ( 'NONE', #67415, #47299 ) ;
#48459=DIRECTION ( 'NONE',  ( -0.000000000000000000, 0.000000000000000000, 1.000000000000000000 ) ) ;
#48464=AXIS2_PLACEMENT_3D ( 'NONE', #75503, #28197, #55231 ) ;
#48486=ORIENTED_EDGE ( 'NONE', *, *, #53430, .F. ) ;
#48487=AXIS2_PLACEMENT_3D ( 'NONE', #65296, #9912, #51765 ) ;
#48491=DIRECTION ( 'NONE',  ( 1.000000000000000000, 0.000000000000000000, 0.000000000000000000 ) ) ;
#48492=VECTOR ( 'NONE', #63881, 1000.000000000000000 ) ;
#48500=CARTESIAN_POINT ( 'NONE',  ( -12.94230769230769162, -3.499999999999999556, 29.75000000000000355 ) ) ;
#48504=AXIS2_PLACEMENT_3D ( 'NONE', #51716, #10756, #45416 ) ;
#48507=VERTEX_POINT ( 'NONE', #28806 ) ;
#48519=ORIENTED_EDGE ( 'NONE', *, *, #7479, .T. ) ;
#48529=CARTESIAN_POINT ( 'NONE',  ( -4.230769230769230838, -7.500000000000000000, 29.75000000000000355 ) ) ;
#48530=SURFACE_STYLE_USAGE ( .BOTH. , #41350 ) ;
#48537=LINE ( 'NONE', #36373, #52980 ) ;
#48548=ORIENTED_EDGE ( 'NONE', *, *, #59065, .F. ) ;
#48553=DIRECTION ( 'NONE',  ( -0.000000000000000000, 1.000000000000000000, -0.000000000000000000 ) ) ;
#48566=LINE ( 'NONE', #19341, #10704 ) ;
#48569=FACE_OUTER_BOUND ( 'NONE', #27069, .T. ) ;
#48576=VECTOR ( 'NONE', #60058, 1000.000000000000000 ) ;
#48589=ORIENTED_EDGE ( 'NONE', *, *, #17456, .F. ) ;
#48591=DIRECTION ( 'NONE',  ( 1.000000000000000000, 0.000000000000000000, 0.000000000000000000 ) ) ;
#48595=ORIENTED_EDGE ( 'NONE', *, *, #33748, .F. ) ;
#48609=CIRCLE ( 'NONE', #5494, 4.000000000000000000 ) ;
#48613=EDGE_LOOP ( 'NONE', ( #74675, #66662, #70858, #28805 ) ) ;
#48617=ORIENTED_EDGE ( 'NONE', *, *, #61153, .T. ) ;
#48621=ORIENTED_EDGE ( 'NONE', *, *, #1829, .T. ) ;
#48625=CARTESIAN_POINT ( 'NONE',  ( 4.480769230769229061, -3.499999999999999556, 29.75000000000000355 ) ) ;
#48646=FACE_OUTER_BOUND ( 'NONE', #15739, .T. ) ;
#48658=VERTEX_POINT ( 'NONE', #46296 ) ;
#48679=CARTESIAN_POINT ( 'NONE',  ( -0.3589743589743593088, -11.50000000000000000, 29.75000000000000355 ) ) ;
#48701=CARTESIAN_POINT ( 'NONE',  ( -19.00000000000000000, -11.00000000000000000, 29.75000000000000355 ) ) ;
#48705=ADVANCED_FACE ( 'NONE', ( #62021 ), #39562, .T. ) ;
#48716=VECTOR ( 'NONE', #55640, 1000.000000000000000 ) ;
#48718=DIRECTION ( 'NONE',  ( 1.000000000000000000, 0.000000000000000000, 0.000000000000000000 ) ) ;
#48719=ORIENTED_EDGE ( 'NONE', *, *, #6773, .F. ) ;
#48727=LINE ( 'NONE', #61345, #50683 ) ;
#48743=PLANE ( 'NONE',  #7177 ) ;
#48752=LINE ( 'NONE', #42897, #86555 ) ;
#48757=ORIENTED_EDGE ( 'NONE', *, *, #26033, .T. ) ;
#48759=CARTESIAN_POINT ( 'NONE',  ( -7.134615384615385025, -3.499999999999999556, 29.75000000000000355 ) ) ;
#48770=ORIENTED_EDGE ( 'NONE', *, *, #32008, .F. ) ;
#48775=DIRECTION ( 'NONE',  ( -1.000000000000000000, -0.000000000000000000, 0.000000000000000000 ) ) ;
#48776=ORIENTED_EDGE ( 'NONE', *, *, #15674, .F. ) ;
#48792=ORIENTED_EDGE ( 'NONE', *, *, #16437, .T. ) ;
#48793=PLANE ( 'NONE',  #3077 ) ;
#48799=UNCERTAINTY_MEASURE_WITH_UNIT (LENGTH_MEASURE( 1.000000000000000082E-05 ), #88673, 'distance_accuracy_value', 'NONE');
#48805=CARTESIAN_POINT ( 'NONE',  ( 20.00000000000000000, -4.000000000000000000, 29.75000000000000355 ) ) ;
#48822=LINE ( 'NONE', #55140, #47014 ) ;
#48836=VECTOR ( 'NONE', #87814, 1000.000000000000000 ) ;
#48846=CARTESIAN_POINT ( 'NONE',  ( -14.87820512820512953, -7.500000000000000000, 33.75000000000000000 ) ) ;
#48848=CARTESIAN_POINT ( 'NONE',  ( 2.544871794871792936, -7.500000000000000000, 29.75000000000000355 ) ) ;
#48851=ORIENTED_EDGE ( 'NONE', *, *, #82278, .F. ) ;
#48865=VERTEX_POINT ( 'NONE', #48500 ) ;
#48870=CARTESIAN_POINT ( 'NONE',  ( -13.91025641025641058, -7.500000000000000000, 33.75000000000000000 ) ) ;
#48871=ORIENTED_EDGE ( 'NONE', *, *, #51244, .T. ) ;
#48877=EDGE_CURVE ( 'NONE', #55049, #9891, #42210, .T. ) ;
#48884=CARTESIAN_POINT ( 'NONE',  ( 12.22435897435897267, -7.500000000000000000, 29.75000000000000355 ) ) ;
#48907=AXIS2_PLACEMENT_3D ( 'NONE', #41390, #68855, #55336 ) ;
#48910=VECTOR ( 'NONE', #18966, 1000.000000000000000 ) ;
#48917=DIRECTION ( 'NONE',  ( -1.000000000000000000, -0.000000000000000000, -0.000000000000000000 ) ) ;
#48938=VERTEX_POINT ( 'NONE', #38548 ) ;
#48942=CARTESIAN_POINT ( 'NONE',  ( -19.50000000000000000, -3.499999999999999556, 29.75000000000000355 ) ) ;
#48943=VERTEX_POINT ( 'NONE', #66002 ) ;
#48944=EDGE_CURVE ( 'NONE', #73852, #5633, #79977, .T. ) ;
#48974=DIRECTION ( 'NONE',  ( -1.000000000000000000, -0.000000000000000000, -0.000000000000000000 ) ) ;
#48980=PLANE ( 'NONE',  #40866 ) ;
#49018=DIRECTION ( 'NONE',  ( -1.000000000000000000, -0.000000000000000000, 0.000000000000000000 ) ) ;
#49026=CARTESIAN_POINT ( 'NONE',  ( 6.166666666666664298, -3.499999999999999556, 29.75000000000000355 ) ) ;
#49034=ORIENTED_EDGE ( 'NONE', *, *, #12405, .T. ) ;
#49040=ORIENTED_EDGE ( 'NONE', *, *, #10635, .F. ) ;
#49041=CARTESIAN_POINT ( 'NONE',  ( 7.384615384615385025, -7.500000000000000000, 33.75000000000000000 ) ) ;
#49044=ORIENTED_EDGE ( 'NONE', *, *, #24899, .F. ) ;
#49045=ORIENTED_EDGE ( 'NONE', *, *, #36587, .T. ) ;
#49047=ORIENTED_EDGE ( 'NONE', *, *, #65645, .T. ) ;
#49053=DIRECTION ( 'NONE',  ( 0.000000000000000000, 0.000000000000000000, -1.000000000000000000 ) ) ;
#49056=ORIENTED_EDGE ( 'NONE', *, *, #40773, .T. ) ;
#49061=EDGE_CURVE ( 'NONE', #18312, #47848, #19604, .T. ) ;
#49083=DIRECTION ( 'NONE',  ( 1.000000000000000000, 0.000000000000000000, 0.000000000000000000 ) ) ;
#49087=CARTESIAN_POINT ( 'NONE',  ( -19.50000000000000000, -11.00000000000000000, 28.25000000000000000 ) ) ;
#49125=FACE_OUTER_BOUND ( 'NONE', #50934, .T. ) ;
#49175=VERTEX_POINT ( 'NONE', #56495 ) ;
#49179=VECTOR ( 'NONE', #76344, 1000.000000000000000 ) ;
#49189=CARTESIAN_POINT ( 'NONE',  ( 20.00000000000000000, -7.500000000000000000, 29.75000000000000355 ) ) ;
#49200=UNCERTAINTY_MEASURE_WITH_UNIT (LENGTH_MEASURE( 1.000000000000000082E-05 ), #55033, 'distance_accuracy_value', 'NONE');
#49210=LINE ( 'NONE', #48759, #33021 ) ;
#49215=ORIENTED_EDGE ( 'NONE', *, *, #34417, .T. ) ;
#49228=CARTESIAN_POINT ( 'NONE',  ( 0.000000000000000000, -11.00000000000000000, 29.75000000000000355 ) ) ;
#49230=VECTOR ( 'NONE', #44367, 1000.000000000000000 ) ;
#49232=ORIENTED_EDGE ( 'NONE', *, *, #55161, .T. ) ;
#49234=ORIENTED_EDGE ( 'NONE', *, *, #44474, .F. ) ;
#49242=CARTESIAN_POINT ( 'NONE',  ( -11.25641025641025550, -3.499999999999999556, 29.75000000000000355 ) ) ;
#49246=DIRECTION ( 'NONE',  ( 0.000000000000000000, 0.000000000000000000, -1.000000000000000000 ) ) ;
#49251=ORIENTED_EDGE ( 'NONE', *, *, #75539, .T. ) ;
#49252=LINE ( 'NONE', #37046, #77171 ) ;
#49265=EDGE_CURVE ( 'NONE', #8287, #20476, #64119, .T. ) ;
#49271=DIRECTION ( 'NONE',  ( -1.000000000000000000, -0.000000000000000000, -0.000000000000000000 ) ) ;
#49280=ORIENTED_EDGE ( 'NONE', *, *, #61175, .F. ) ;
#49281=DIRECTION ( 'NONE',  ( 0.000000000000000000, 0.000000000000000000, -1.000000000000000000 ) ) ;
#49299=DIRECTION ( 'NONE',  ( -1.000000000000000000, -0.000000000000000000, 0.000000000000000000 ) ) ;
#49308=DIRECTION ( 'NONE',  ( 1.000000000000000000, 0.000000000000000000, 0.000000000000000000 ) ) ;
#49314=EDGE_CURVE ( 'NONE', #75229, #13394, #73112, .T. ) ;
#49321=CARTESIAN_POINT ( 'NONE',  ( 5.198717948717946236, -3.499999999999999556, 29.75000000000000355 ) ) ;
#49339=CARTESIAN_POINT ( 'NONE',  ( -11.25641025641025550, -7.500000000000000000, 29.75000000000000355 ) ) ;
#49341=CARTESIAN_POINT ( 'NONE',  ( 11.25641025641025550, -3.499999999999999556, 29.75000000000000355 ) ) ;
#49347=STYLED_ITEM ( 'NONE', ( #76013 ), #28293 ) ;
#49355=ORIENTED_EDGE ( 'NONE', *, *, #26942, .T. ) ;
#49363=DIRECTION ( 'NONE',  ( -1.000000000000000000, -0.000000000000000000, -0.000000000000000000 ) ) ;
#49365=LINE ( 'NONE', #49798, #5998 ) ;
#49369=ADVANCED_FACE ( 'NONE', ( #33459 ), #38896, .F. ) ;
#49380=ADVANCED_FACE ( 'NONE', ( #35114 ), #73574, .T. ) ;
#49385=VERTEX_POINT ( 'NONE', #74898 ) ;
#49387=ORIENTED_EDGE ( 'NONE', *, *, #52737, .T. ) ;
#49392=DIRECTION ( 'NONE',  ( 0.000000000000000000, -1.000000000000000000, 0.000000000000000000 ) ) ;
#49418=DIRECTION ( 'NONE',  ( 1.000000000000000000, 0.000000000000000000, 0.000000000000000000 ) ) ;
#49453=ORIENTED_EDGE ( 'NONE', *, *, #16391, .T. ) ;
#49466=DIRECTION ( 'NONE',  ( 0.000000000000000000, 0.000000000000000000, -1.000000000000000000 ) ) ;
#49494=DIRECTION ( 'NONE',  ( 1.000000000000000000, 0.000000000000000000, 0.000000000000000000 ) ) ;
#49497=LINE ( 'NONE', #70650, #88774 ) ;
#49507=LINE ( 'NONE', #29679, #66518 ) ;
#49508=ADVANCED_FACE ( 'NONE', ( #52610 ), #31457, .F. ) ;
#49509=EDGE_CURVE ( 'NONE', #22240, #75095, #72437, .T. ) ;
#49521=ORIENTED_EDGE ( 'NONE', *, *, #76637, .F. ) ;
#49523=ORIENTED_EDGE ( 'NONE', *, *, #33188, .T. ) ;
#49534=VECTOR ( 'NONE', #81050, 1000.000000000000000 ) ;
#49536=DIRECTION ( 'NONE',  ( -1.000000000000000000, -0.000000000000000000, -0.000000000000000000 ) ) ;
#49539=ORIENTED_EDGE ( 'NONE', *, *, #18578, .F. ) ;
#49554=DIRECTION ( 'NONE',  ( 1.000000000000000000, 0.000000000000000000, 0.000000000000000000 ) ) ;
#49572=FACE_OUTER_BOUND ( 'NONE', #79034, .T. ) ;
#49577=DIRECTION ( 'NONE',  ( 1.000000000000000000, 0.000000000000000000, 0.000000000000000000 ) ) ;
#49583=EDGE_CURVE ( 'NONE', #79249, #55049, #59819, .T. ) ;
#49586=ORIENTED_EDGE ( 'NONE', *, *, #23328, .T. ) ;
#49641=LINE ( 'NONE', #78436, #50426 ) ;
#49649=VECTOR ( 'NONE', #61622, 1000.000000000000000 ) ;
#49653=DIRECTION ( 'NONE',  ( -1.000000000000000000, -0.000000000000000000, 0.000000000000000000 ) ) ;
#49670=ORIENTED_EDGE ( 'NONE', *, *, #24074, .T. ) ;
#49678=CARTESIAN_POINT ( 'NONE',  ( -20.00000000000000000, -7.500000000000000000, 29.75000000000000355 ) ) ;
#49700=EDGE_CURVE ( 'NONE', #15714, #27642, #75993, .T. ) ;
#49702=CARTESIAN_POINT ( 'NONE',  ( -3.262820512820514107, -3.499999999999999556, 29.75000000000000355 ) ) ;
#49704=VERTEX_POINT ( 'NONE', #61141 ) ;
#49710=FACE_OUTER_BOUND ( 'NONE', #86172, .T. ) ;
#49724=VECTOR ( 'NONE', #62472, 1000.000000000000000 ) ;
#49729=VERTEX_POINT ( 'NONE', #13407 ) ;
#49737=EDGE_LOOP ( 'NONE', ( #21021, #58735, #78607, #86146 ) ) ;
#49748=ORIENTED_EDGE ( 'NONE', *, *, #39859, .T. ) ;
#49758=DIRECTION ( 'NONE',  ( 0.000000000000000000, 0.000000000000000000, -1.000000000000000000 ) ) ;
#49766=DIRECTION ( 'NONE',  ( 0.000000000000000000, 1.000000000000000000, 0.000000000000000000 ) ) ;
#49774=FACE_OUTER_BOUND ( 'NONE', #82793, .T. ) ;
#49778=ORIENTED_EDGE ( 'NONE', *, *, #79517, .F. ) ;
#49786=VECTOR ( 'NONE', #75561, 1000.000000000000000 ) ;
#49787=ORIENTED_EDGE ( 'NONE', *, *, #29265, .T. ) ;
#49798=CARTESIAN_POINT ( 'NONE',  ( -9.320512820512821150, -3.499999999999999556, 29.75000000000000355 ) ) ;
#49804=AXIS2_PLACEMENT_3D ( 'NONE', #31639, #16782, #59099 ) ;
#49805=CARTESIAN_POINT ( 'NONE',  ( -11.00641025641025550, -11.50000000000000000, 29.75000000000000355 ) ) ;
#49811=VECTOR ( 'NONE', #10607, 1000.000000000000000 ) ;
#49813=LINE ( 'NONE', #64203, #31972 ) ;
#49819=ORIENTED_EDGE ( 'NONE', *, *, #29160, .F. ) ;
#49834=FACE_OUTER_BOUND ( 'NONE', #44094, .T. ) ;
#49855=LINE ( 'NONE', #20617, #38538 ) ;
#49858=DIRECTION ( 'NONE',  ( -1.000000000000000000, -0.000000000000000000, -0.000000000000000000 ) ) ;
#49866=AXIS2_PLACEMENT_3D ( 'NONE', #38412, #80296, #87069 ) ;
#49871=DIRECTION ( 'NONE',  ( 1.000000000000000000, 0.000000000000000000, 0.000000000000000000 ) ) ;
#49873=LINE ( 'NONE', #56198, #61667 ) ;
#49877=DIRECTION ( 'NONE',  ( 1.000000000000000000, 0.000000000000000000, 0.000000000000000000 ) ) ;
#49912=CARTESIAN_POINT ( 'NONE',  ( 1.576923076923075762, -7.500000000000000000, 29.75000000000000355 ) ) ;
#49913=ORIENTED_EDGE ( 'NONE', *, *, #66537, .F. ) ;
#49916=ORIENTED_EDGE ( 'NONE', *, *, #52677, .T. ) ;
#49926=EDGE_CURVE ( 'NONE', #18170, #35531, #18287, .T. ) ;
#49930=DIRECTION ( 'NONE',  ( 0.000000000000000000, 0.000000000000000000, -1.000000000000000000 ) ) ;
#49951=AXIS2_PLACEMENT_3D ( 'NONE', #85602, #23879, #10388 ) ;
#49964=DIRECTION ( 'NONE',  ( -1.000000000000000000, -0.000000000000000000, 0.000000000000000000 ) ) ;
#49967=VECTOR ( 'NONE', #5058, 1000.000000000000000 ) ;
#49986=LINE ( 'NONE', #84685, #53510 ) ;
#49996=CARTESIAN_POINT ( 'NONE',  ( -15.84615384615384670, -11.50000000000000000, 29.75000000000000355 ) ) ;
#50011=VECTOR ( 'NONE', #32751, 1000.000000000000000 ) ;
#50030=CARTESIAN_POINT ( 'NONE',  ( 7.384615384615385025, -7.500000000000000000, 33.75000000000000000 ) ) ;
#50033=FACE_OUTER_BOUND ( 'NONE', #46347, .T. ) ;
#50038=DIRECTION ( 'NONE',  ( -0.000000000000000000, 1.000000000000000000, -0.000000000000000000 ) ) ;
#50049=ORIENTED_EDGE ( 'NONE', *, *, #76854, .T. ) ;
#50055=FACE_OUTER_BOUND ( 'NONE', #62258, .T. ) ;
#50064=DIRECTION ( 'NONE',  ( -1.000000000000000000, -0.000000000000000000, -0.000000000000000000 ) ) ;
#50069=DIRECTION ( 'NONE',  ( -1.000000000000000000, -0.000000000000000000, -0.000000000000000000 ) ) ;
#50070=LINE ( 'NONE', #16296, #3044 ) ;
#50073=EDGE_LOOP ( 'NONE', ( #5476, #51537, #63361, #42839 ) ) ;
#50090=VERTEX_POINT ( 'NONE', #70012 ) ;
#50098=CARTESIAN_POINT ( 'NONE',  ( 12.22435897435897267, -7.500000000000000000, 33.75000000000000000 ) ) ;
#50109=EDGE_CURVE ( 'NONE', #21924, #34293, #69133, .T. ) ;
#50126=CARTESIAN_POINT ( 'NONE',  ( -5.448717948717947124, -4.000000000000000000, 29.75000000000000355 ) ) ;
#50164=CIRCLE ( 'NONE', #11360, 4.000000000000000000 ) ;
#50166=LINE ( 'NONE', #77209, #85467 ) ;
#50168=ADVANCED_FACE ( 'NONE', ( #29925 ), #57381, .F. ) ;
#50170=EDGE_LOOP ( 'NONE', ( #45319, #58141, #44103, #39119 ) ) ;
#50189=CARTESIAN_POINT ( 'NONE',  ( 15.12820512820512953, -7.500000000000000000, 33.75000000000000000 ) ) ;
#50195=PLANE ( 'NONE',  #22553 ) ;
#50226=DIRECTION ( 'NONE',  ( 1.000000000000000000, 0.000000000000000000, 0.000000000000000000 ) ) ;
#50235=VECTOR ( 'NONE', #2311, 1000.000000000000000 ) ;
#50240=CARTESIAN_POINT ( 'NONE',  ( 0.6089743589743582541, -3.499999999999999556, 29.75000000000000355 ) ) ;
#50243=VECTOR ( 'NONE', #71767, 1000.000000000000000 ) ;
#50245=VECTOR ( 'NONE', #63539, 1000.000000000000000 ) ;
#50249=ORIENTED_EDGE ( 'NONE', *, *, #68714, .F. ) ;
#50250=ORIENTED_EDGE ( 'NONE', *, *, #49314, .F. ) ;
#50256=EDGE_CURVE ( 'NONE', #60579, #18944, #23596, .T. ) ;
#50264=EDGE_CURVE ( 'NONE', #13929, #32893, #30361, .T. ) ;
#50273=ORIENTED_EDGE ( 'NONE', *, *, #27038, .T. ) ;
#50277=VERTEX_POINT ( 'NONE', #31703 ) ;
#50278=VECTOR ( 'NONE', #67595, 1000.000000000000000 ) ;
#50293=LINE ( 'NONE', #2121, #17519 ) ;
#50296=EDGE_CURVE ( 'NONE', #47433, #15714, #16845, .T. ) ;
#50301=AXIS2_PLACEMENT_3D ( 'NONE', #24555, #17360, #45266 ) ;
#50312=CARTESIAN_POINT ( 'NONE',  ( 0.000000000000000000, -11.00000000000000000, 29.75000000000000355 ) ) ;
#50319=EDGE_LOOP ( 'NONE', ( #13067, #76526, #33725, #37184 ) ) ;
#50323=DIRECTION ( 'NONE',  ( 0.000000000000000000, 1.000000000000000000, 0.000000000000000000 ) ) ;
#50357=EDGE_CURVE ( 'NONE', #58158, #345, #33475, .T. ) ;
#50358=DIRECTION ( 'NONE',  ( 0.000000000000000000, 0.000000000000000000, -1.000000000000000000 ) ) ;
#50366=VECTOR ( 'NONE', #25599, 1000.000000000000000 ) ;
#50373=( GEOMETRIC_REPRESENTATION_CONTEXT ( 3 ) GLOBAL_UNCERTAINTY_ASSIGNED_CONTEXT ( ( #62697 ) ) GLOBAL_UNIT_ASSIGNED_CONTEXT ( ( #39608, #38252, #52648 ) ) REPRESENTATION_CONTEXT ( 'NONE', 'WORKASPACE' ) );
#50383=ORIENTED_EDGE ( 'NONE', *, *, #5376, .F. ) ;
#50388=DIRECTION ( 'NONE',  ( 0.000000000000000000, 0.000000000000000000, -1.000000000000000000 ) ) ;
#50389=CARTESIAN_POINT ( 'NONE',  ( -4.230769230769230838, -7.500000000000000000, 29.75000000000000355 ) ) ;
#50419=LINE ( 'NONE', #7687, #15140 ) ;
#50423=ORIENTED_EDGE ( 'NONE', *, *, #79079, .F. ) ;
#50426=VECTOR ( 'NONE', #29387, 1000.000000000000000 ) ;
#50431=CARTESIAN_POINT ( 'NONE',  ( 11.97435897435897267, -4.000000000000000000, 29.75000000000000355 ) ) ;
#50432=CARTESIAN_POINT ( 'NONE',  ( -11.25641025641025195, -4.000000000000000000, 29.75000000000000355 ) ) ;
#50433=DIRECTION ( 'NONE',  ( -0.000000000000000000, 1.000000000000000000, -0.000000000000000000 ) ) ;
#50434=DIRECTION ( 'NONE',  ( -0.000000000000000000, -1.000000000000000000, -0.000000000000000000 ) ) ;
#50439=EDGE_CURVE ( 'NONE', #86419, #40595, #75778, .T. ) ;
#50446=CARTESIAN_POINT ( 'NONE',  ( -0.6089743589743593644, -3.499999999999999556, 29.75000000000000355 ) ) ;
#50448=PLANE ( 'NONE',  #71502 ) ;
#50488=ORIENTED_EDGE ( 'NONE', *, *, #4551, .T. ) ;
#50498=ORIENTED_EDGE ( 'NONE', *, *, #13927, .F. ) ;
#50514=VERTEX_POINT ( 'NONE', #32908 ) ;
#50515=ORIENTED_EDGE ( 'NONE', *, *, #35986, .F. ) ;
#50522=ORIENTED_EDGE ( 'NONE', *, *, #24074, .F. ) ;
#50537=ORIENTED_EDGE ( 'NONE', *, *, #46509, .F. ) ;
#50541=CARTESIAN_POINT ( 'NONE',  ( 10.28846153846153832, -3.499999999999999556, 29.75000000000000355 ) ) ;
#50542=VERTEX_POINT ( 'NONE', #39682 ) ;
#50557=EDGE_CURVE ( 'NONE', #11880, #14834, #52721, .T. ) ;
#50583=ORIENTED_EDGE ( 'NONE', *, *, #79306, .F. ) ;
#50587=ORIENTED_EDGE ( 'NONE', *, *, #24131, .T. ) ;
#50603=LINE ( 'NONE', #24012, #72994 ) ;
#50612=EDGE_CURVE ( 'NONE', #81234, #51205, #455, .T. ) ;
#50621=ORIENTED_EDGE ( 'NONE', *, *, #20527, .T. ) ;
#50624=EDGE_LOOP ( 'NONE', ( #39962, #69578, #44302, #38665 ) ) ;
#50625=DIRECTION ( 'NONE',  ( 0.000000000000000000, 0.000000000000000000, -1.000000000000000000 ) ) ;
#50633=EDGE_LOOP ( 'NONE', ( #78789, #35448, #38211, #88730, #41075 ) ) ;
#50643=CARTESIAN_POINT ( 'NONE',  ( 13.91025641025641235, -3.499999999999999556, 29.75000000000000355 ) ) ;
#50649=DIRECTION ( 'NONE',  ( -1.000000000000000000, -0.000000000000000000, -0.000000000000000000 ) ) ;
#50667=FACE_OUTER_BOUND ( 'NONE', #62203, .T. ) ;
#50683=VECTOR ( 'NONE', #28019, 1000.000000000000000 ) ;
#50689=DIRECTION ( 'NONE',  ( 1.000000000000000000, 0.000000000000000000, 0.000000000000000000 ) ) ;
#50696=ORIENTED_EDGE ( 'NONE', *, *, #75181, .T. ) ;
#50705=ORIENTED_EDGE ( 'NONE', *, *, #77670, .T. ) ;
#50709=CARTESIAN_POINT ( 'NONE',  ( 3.262820512820510999, -3.499999999999999556, 29.75000000000000355 ) ) ;
#50715=ORIENTED_EDGE ( 'NONE', *, *, #63468, .F. ) ;
#50717=VERTEX_POINT ( 'NONE', #82876 ) ;
#50719=ORIENTED_EDGE ( 'NONE', *, *, #83687, .T. ) ;
#50725=ORIENTED_EDGE ( 'NONE', *, *, #75539, .F. ) ;
#50737=( NAMED_UNIT ( * ) PLANE_ANGLE_UNIT ( ) SI_UNIT ( $, .RADIAN. ) );
#50754=DIRECTION ( 'NONE',  ( 0.000000000000000000, 0.000000000000000000, 1.000000000000000000 ) ) ;
#50765=LINE ( 'NONE', #64729, #1503 ) ;
#50766=VECTOR ( 'NONE', #33089, 1000.000000000000000 ) ;
#50768=CARTESIAN_POINT ( 'NONE',  ( 19.50000000000000000, -7.500000000000000000, 33.75000000000000000 ) ) ;
#50772=CARTESIAN_POINT ( 'NONE',  ( 20.00000000000000000, -4.000000000000000000, 29.75000000000000355 ) ) ;
#50781=PLANE ( 'NONE',  #22686 ) ;
#50783=ORIENTED_EDGE ( 'NONE', *, *, #64633, .T. ) ;
#50787=FACE_OUTER_BOUND ( 'NONE', #68420, .T. ) ;
#50795=EDGE_LOOP ( 'NONE', ( #84732, #82737, #49232, #89006 ) ) ;
#50803=DIRECTION ( 'NONE',  ( 1.000000000000000000, 0.000000000000000000, 0.000000000000000000 ) ) ;
#50805=LINE ( 'NONE', #45839, #298 ) ;
#50806=EDGE_CURVE ( 'NONE', #56977, #51043, #84806, .T. ) ;
#50808=ORIENTED_EDGE ( 'NONE', *, *, #63569, .T. ) ;
#50811=ORIENTED_EDGE ( 'NONE', *, *, #80705, .F. ) ;
#50813=EDGE_CURVE ( 'NONE', #5990, #5809, #57596, .T. ) ;
#50818=EDGE_LOOP ( 'NONE', ( #57583, #29923, #60420, #23732 ) ) ;
#50834=CARTESIAN_POINT ( 'NONE',  ( 10.28846153846153832, -7.500000000000000000, 29.75000000000000355 ) ) ;
#50848=AXIS2_PLACEMENT_3D ( 'NONE', #77751, #8865, #51140 ) ;
#50850=LINE ( 'NONE', #37347, #4260 ) ;
#50855=VERTEX_POINT ( 'NONE', #37318 ) ;
#50875=FACE_OUTER_BOUND ( 'NONE', #62593, .T. ) ;
#50913=ORIENTED_EDGE ( 'NONE', *, *, #21316, .T. ) ;
#50917=CARTESIAN_POINT ( 'NONE',  ( -0.3589743589743593088, -7.500000000000000000, 29.75000000000000355 ) ) ;
#50921=EDGE_CURVE ( 'NONE', #29864, #955, #38888, .T. ) ;
#50934=EDGE_LOOP ( 'NONE', ( #46646, #12158, #77146, #53936, #21181 ) ) ;
#50947=CARTESIAN_POINT ( 'NONE',  ( -18.75000000000000000, -3.499999999999999556, 29.75000000000000355 ) ) ;
#50953=DIRECTION ( 'NONE',  ( -0.000000000000000000, 0.000000000000000000, 1.000000000000000000 ) ) ;
#50957=VERTEX_POINT ( 'NONE', #46309 ) ;
#50984=VECTOR ( 'NONE', #49392, 1000.000000000000000 ) ;
#51001=DIRECTION ( 'NONE',  ( -0.000000000000000000, 1.000000000000000000, -0.000000000000000000 ) ) ;
#51003=FACE_OUTER_BOUND ( 'NONE', #4240, .T. ) ;
#51015=CIRCLE ( 'NONE', #30895, 4.000000000000000000 ) ;
#51033=VECTOR ( 'NONE', #17542, 1000.000000000000000 ) ;
#51034=DIRECTION ( 'NONE',  ( -0.000000000000000000, 1.000000000000000000, -0.000000000000000000 ) ) ;
#51035=CARTESIAN_POINT ( 'NONE',  ( 20.00000000000000000, -4.000000000000000000, 29.75000000000000355 ) ) ;
#51040=LINE ( 'NONE', #45188, #28361 ) ;
#51043=VERTEX_POINT ( 'NONE', #69243 ) ;
#51059=DIRECTION ( 'NONE',  ( 0.000000000000000000, 0.000000000000000000, -1.000000000000000000 ) ) ;
#51062=CARTESIAN_POINT ( 'NONE',  ( 9.320512820512821150, -7.500000000000000000, 29.75000000000000355 ) ) ;
#51069=ORIENTED_EDGE ( 'NONE', *, *, #73427, .F. ) ;
#51073=DIRECTION ( 'NONE',  ( 1.000000000000000000, 0.000000000000000000, 0.000000000000000000 ) ) ;
#51074=DIRECTION ( 'NONE',  ( 0.000000000000000000, 0.000000000000000000, -1.000000000000000000 ) ) ;
#51075=CARTESIAN_POINT ( 'NONE',  ( -14.16025641025641058, -7.500000000000000000, 29.75000000000000355 ) ) ;
#51089=ORIENTED_EDGE ( 'NONE', *, *, #87488, .F. ) ;
#51092=DIRECTION ( 'NONE',  ( 0.000000000000000000, 0.000000000000000000, -1.000000000000000000 ) ) ;
#51101=DIRECTION ( 'NONE',  ( 1.000000000000000000, 0.000000000000000000, 0.000000000000000000 ) ) ;
#51107=EDGE_CURVE ( 'NONE', #87423, #64241, #2853, .T. ) ;
#51109=VECTOR ( 'NONE', #26311, 1000.000000000000000 ) ;
#51111=CARTESIAN_POINT ( 'NONE',  ( -15.12820512820512953, -3.499999999999999556, 29.75000000000000355 ) ) ;
#51114=ADVANCED_FACE ( 'NONE', ( #57934 ), #29591, .T. ) ;
#51116=CARTESIAN_POINT ( 'NONE',  ( 0.000000000000000000, -11.00000000000000000, 29.75000000000000355 ) ) ;
#51120=VECTOR ( 'NONE', #23474, 1000.000000000000000 ) ;
#51133=AXIS2_PLACEMENT_3D ( 'NONE', #12157, #31531, #53121 ) ;
#51134=ORIENTED_EDGE ( 'NONE', *, *, #1103, .T. ) ;
#51140=DIRECTION ( 'NONE',  ( 0.000000000000000000, 0.000000000000000000, 1.000000000000000000 ) ) ;
#51147=ORIENTED_EDGE ( 'NONE', *, *, #84704, .F. ) ;
#51150=ORIENTED_EDGE ( 'NONE', *, *, #80913, .T. ) ;
#51166=EDGE_CURVE ( 'NONE', #51205, #85054, #31682, .T. ) ;
#51170=ORIENTED_EDGE ( 'NONE', *, *, #52585, .T. ) ;
#51180=EDGE_CURVE ( 'NONE', #57194, #29384, #84102, .T. ) ;
#51181=DIRECTION ( 'NONE',  ( 0.000000000000000000, 0.000000000000000000, -1.000000000000000000 ) ) ;
#51198=DIRECTION ( 'NONE',  ( 1.000000000000000000, 0.000000000000000000, 0.000000000000000000 ) ) ;
#51204=LINE ( 'NONE', #50772, #41372 ) ;
#51205=VERTEX_POINT ( 'NONE', #71012 ) ;
#51214=DIRECTION ( 'NONE',  ( 0.000000000000000000, 0.000000000000000000, 1.000000000000000000 ) ) ;
#51237=ORIENTED_EDGE ( 'NONE', *, *, #65645, .F. ) ;
#51239=AXIS2_PLACEMENT_3D ( 'NONE', #39537, #33203, #60667 ) ;
#51242=ORIENTED_EDGE ( 'NONE', *, *, #11303, .F. ) ;
#51244=EDGE_CURVE ( 'NONE', #49175, #8541, #64235, .T. ) ;
#51257=LINE ( 'NONE', #79662, #38432 ) ;
#51276=ORIENTED_EDGE ( 'NONE', *, *, #37856, .T. ) ;
#51296=CARTESIAN_POINT ( 'NONE',  ( -3.512820512820513663, -7.500000000000000000, 29.75000000000000355 ) ) ;
#51316=AXIS2_PLACEMENT_3D ( 'NONE', #70040, #50649, #78128 ) ;
#51318=EDGE_CURVE ( 'NONE', #48507, #21400, #56114, .T. ) ;
#51323=VECTOR ( 'NONE', #22206, 1000.000000000000000 ) ;
#51353=LINE ( 'NONE', #10412, #87052 ) ;
#51357=ADVANCED_FACE ( 'NONE', ( #58820 ), #24596, .F. ) ;
#51358=ORIENTED_EDGE ( 'NONE', *, *, #87174, .T. ) ;
#51371=DIRECTION ( 'NONE',  ( 0.000000000000000000, 0.000000000000000000, -1.000000000000000000 ) ) ;
#51375=ADVANCED_FACE ( 'NONE', ( #47968 ), #6112, .T. ) ;
#51381=CARTESIAN_POINT ( 'NONE',  ( -19.50000000000000000, -11.50000000000000000, 29.75000000000000355 ) ) ;
#51391=ORIENTED_EDGE ( 'NONE', *, *, #29547, .F. ) ;
#51407=ORIENTED_EDGE ( 'NONE', *, *, #87760, .F. ) ;
#51410=CARTESIAN_POINT ( 'NONE',  ( 4.480769230769229061, -11.50000000000000000, 29.75000000000000355 ) ) ;
#51413=DIRECTION ( 'NONE',  ( 0.000000000000000000, 0.000000000000000000, -1.000000000000000000 ) ) ;
#51423=ORIENTED_EDGE ( 'NONE', *, *, #30049, .T. ) ;
#51429=DIRECTION ( 'NONE',  ( 0.000000000000000000, 0.000000000000000000, 1.000000000000000000 ) ) ;
#51438=CARTESIAN_POINT ( 'NONE',  ( -6.166666666666667851, -7.500000000000000000, 29.75000000000000355 ) ) ;
#51458=AXIS2_PLACEMENT_3D ( 'NONE', #71851, #65981, #10160 ) ;
#51464=ADVANCED_FACE ( 'NONE', ( #31583 ), #15086, .T. ) ;
#51466=CARTESIAN_POINT ( 'NONE',  ( -9.070512820512819374, -7.500000000000000000, 29.75000000000000355 ) ) ;
#51470=EDGE_CURVE ( 'NONE', #13621, #43102, #86094, .T. ) ;
#51485=AXIS2_PLACEMENT_3D ( 'NONE', #73670, #59245, #26356 ) ;
#51486=ORIENTED_EDGE ( 'NONE', *, *, #36958, .T. ) ;
#51499=VERTEX_POINT ( 'NONE', #86550 ) ;
#51524=DIRECTION ( 'NONE',  ( 0.000000000000000000, 0.000000000000000000, -1.000000000000000000 ) ) ;
#51534=ORIENTED_EDGE ( 'NONE', *, *, #49583, .T. ) ;
#51536=EDGE_CURVE ( 'NONE', #47433, #74652, #72565, .T. ) ;
#51537=ORIENTED_EDGE ( 'NONE', *, *, #27806, .F. ) ;
#51542=DIRECTION ( 'NONE',  ( -0.000000000000000000, 1.000000000000000000, -0.000000000000000000 ) ) ;
#51565=EDGE_CURVE ( 'NONE', #13394, #14834, #83554, .T. ) ;
#51567=LINE ( 'NONE', #30439, #57956 ) ;
#51577=AXIS2_PLACEMENT_3D ( 'NONE', #16019, #64183, #43927 ) ;
#51581=VECTOR ( 'NONE', #68818, 1000.000000000000000 ) ;
#51597=DIRECTION ( 'NONE',  ( 1.000000000000000000, 0.000000000000000000, 0.000000000000000000 ) ) ;
#51615=VERTEX_POINT ( 'NONE', #46872 ) ;
#51627=PLANE ( 'NONE',  #77053 ) ;
#51633=EDGE_CURVE ( 'NONE', #15955, #21459, #88336, .T. ) ;
#51634=ORIENTED_EDGE ( 'NONE', *, *, #26498, .F. ) ;
#51637=LINE ( 'NONE', #38600, #82377 ) ;
#51656=DIRECTION ( 'NONE',  ( 0.000000000000000000, 0.000000000000000000, -1.000000000000000000 ) ) ;
#51667=CYLINDRICAL_SURFACE ( 'NONE', #72758, 4.000000000000000000 ) ;
#51668=ORIENTED_EDGE ( 'NONE', *, *, #32979, .F. ) ;
#51674=VERTEX_POINT ( 'NONE', #49087 ) ;
#51705=DIRECTION ( 'NONE',  ( -1.000000000000000000, 0.000000000000000000, -0.000000000000000000 ) ) ;
#51707=CIRCLE ( 'NONE', #43064, 4.000000000000000000 ) ;
#51716=CARTESIAN_POINT ( 'NONE',  ( -19.50000000000000000, -3.499999999999999556, 29.75000000000000355 ) ) ;
#51722=CARTESIAN_POINT ( 'NONE',  ( -19.50000000000000000, -3.499999999999999556, 29.75000000000000355 ) ) ;
#51738=DIRECTION ( 'NONE',  ( -0.000000000000000000, 1.000000000000000000, -0.000000000000000000 ) ) ;
#51744=DIRECTION ( 'NONE',  ( -0.000000000000000000, 0.000000000000000000, 1.000000000000000000 ) ) ;
#51746=DIRECTION ( 'NONE',  ( 1.000000000000000000, 0.000000000000000000, 0.000000000000000000 ) ) ;
#51755=ORIENTED_EDGE ( 'NONE', *, *, #82751, .F. ) ;
#51762=DIRECTION ( 'NONE',  ( 0.000000000000000000, 0.000000000000000000, -1.000000000000000000 ) ) ;
#51765=DIRECTION ( 'NONE',  ( -1.000000000000000000, 0.000000000000000000, -0.000000000000000000 ) ) ;
#51774=DIRECTION ( 'NONE',  ( 1.000000000000000000, 0.000000000000000000, 0.000000000000000000 ) ) ;
#51776=VERTEX_POINT ( 'NONE', #469 ) ;
#51782=ORIENTED_EDGE ( 'NONE', *, *, #86278, .T. ) ;
#51803=ORIENTED_EDGE ( 'NONE', *, *, #13142, .F. ) ;
#51813=ORIENTED_EDGE ( 'NONE', *, *, #21616, .T. ) ;
#51827=DIRECTION ( 'NONE',  ( 1.000000000000000000, 0.000000000000000000, 0.000000000000000000 ) ) ;
#51834=VERTEX_POINT ( 'NONE', #30581 ) ;
#51837=VECTOR ( 'NONE', #9643, 1000.000000000000000 ) ;
#51855=ORIENTED_EDGE ( 'NONE', *, *, #20804, .F. ) ;
#51875=AXIS2_PLACEMENT_3D ( 'NONE', #69197, #62421, #82279 ) ;
#51889=DIRECTION ( 'NONE',  ( 1.000000000000000000, 0.000000000000000000, 0.000000000000000000 ) ) ;
#51896=AXIS2_PLACEMENT_3D ( 'NONE', #83381, #83831, #71175 ) ;
#51898=ORIENTED_EDGE ( 'NONE', *, *, #13978, .T. ) ;
#51929=ORIENTED_EDGE ( 'NONE', *, *, #77180, .T. ) ;
#51936=CARTESIAN_POINT ( 'NONE',  ( -9.320512820512821150, -7.500000000000000000, 33.75000000000000000 ) ) ;
#51946=DIRECTION ( 'NONE',  ( 0.000000000000000000, 0.000000000000000000, -1.000000000000000000 ) ) ;
#51968=DIRECTION ( 'NONE',  ( 0.000000000000000000, 0.000000000000000000, -1.000000000000000000 ) ) ;
#51976=PLANE ( 'NONE',  #72932 ) ;
#51977=ORIENTED_EDGE ( 'NONE', *, *, #53523, .F. ) ;
#51983=ADVANCED_FACE ( 'NONE', ( #74249 ), #81014, .F. ) ;
#51993=EDGE_CURVE ( 'NONE', #54682, #88786, #40475, .T. ) ;
#52004=DIRECTION ( 'NONE',  ( -0.000000000000000000, 1.000000000000000000, -0.000000000000000000 ) ) ;
#52008=CARTESIAN_POINT ( 'NONE',  ( 20.00000000000000000, -4.000000000000000000, 29.75000000000000355 ) ) ;
#52023=CARTESIAN_POINT ( 'NONE',  ( 1.326923076923075762, -3.499999999999999556, 29.75000000000000355 ) ) ;
#52062=CARTESIAN_POINT ( 'NONE',  ( -19.50000000000000000, -3.499999999999999556, 29.75000000000000355 ) ) ;
#52066=ADVANCED_FACE ( 'NONE', ( #26953 ), #82788, .T. ) ;
#52070=CARTESIAN_POINT ( 'NONE',  ( 19.50000000000000000, -11.50000000000000000, 29.75000000000000355 ) ) ;
#52087=CARTESIAN_POINT ( 'NONE',  ( 20.00000000000000000, -4.000000000000000000, 29.75000000000000355 ) ) ;
#52092=DIRECTION ( 'NONE',  ( -1.000000000000000000, 0.000000000000000000, -0.000000000000000000 ) ) ;
#52103=CARTESIAN_POINT ( 'NONE',  ( -19.50000000000000000, -3.499999999999999556, 29.75000000000000355 ) ) ;
#52109=LINE ( 'NONE', #10252, #77734 ) ;
#52131=ADVANCED_FACE ( 'NONE', ( #35924 ), #71028, .T. ) ;
#52133=CARTESIAN_POINT ( 'NONE',  ( -6.166666666666667851, -7.500000000000000000, 33.75000000000000000 ) ) ;
#52136=AXIS2_PLACEMENT_3D ( 'NONE', #7586, #76486, #35047 ) ;
#52139=LINE ( 'NONE', #32330, #992 ) ;
#52144=CARTESIAN_POINT ( 'NONE',  ( 12.94230769230769340, -3.499999999999999556, 29.75000000000000355 ) ) ;
#52150=VERTEX_POINT ( 'NONE', #71460 ) ;
#52152=CARTESIAN_POINT ( 'NONE',  ( 20.00000000000000000, -4.000000000000000000, 29.75000000000000355 ) ) ;
#52183=ORIENTED_EDGE ( 'NONE', *, *, #29160, .T. ) ;
#52188=VECTOR ( 'NONE', #80446, 1000.000000000000000 ) ;
#52202=ORIENTED_EDGE ( 'NONE', *, *, #67452, .F. ) ;
#52213=DIRECTION ( 'NONE',  ( -1.000000000000000000, -0.000000000000000000, 0.000000000000000000 ) ) ;
#52238=ADVANCED_FACE ( 'NONE', ( #18756 ), #72794, .T. ) ;
#52263=AXIS2_PLACEMENT_3D ( 'NONE', #63981, #9490, #64866 ) ;
#52264=AXIS2_PLACEMENT_3D ( 'NONE', #47503, #83530, #81751 ) ;
#52281=DIRECTION ( 'NONE',  ( 1.000000000000000000, 0.000000000000000000, 0.000000000000000000 ) ) ;
#52285=AXIS2_PLACEMENT_3D ( 'NONE', #88829, #53685, #54566 ) ;
#52294=ORIENTED_EDGE ( 'NONE', *, *, #18193, .T. ) ;
#52299=DIRECTION ( 'NONE',  ( 1.000000000000000000, 0.000000000000000000, 0.000000000000000000 ) ) ;
#52300=DIRECTION ( 'NONE',  ( 0.000000000000000000, 0.000000000000000000, -1.000000000000000000 ) ) ;
#52303=CARTESIAN_POINT ( 'NONE',  ( 13.91025641025641235, -3.499999999999999556, 29.75000000000000355 ) ) ;
#52310=PRODUCT_CONTEXT ( 'NONE', #83770, 'mechanical' ) ;
#52341=LINE ( 'NONE', #64966, #63178 ) ;
#52342=CARTESIAN_POINT ( 'NONE',  ( 0.000000000000000000, -11.00000000000000000, 29.75000000000000355 ) ) ;
#52347=EDGE_CURVE ( 'NONE', #38268, #46042, #20517, .T. ) ;
#52353=AXIS2_PLACEMENT_3D ( 'NONE', #79852, #59122, #87074 ) ;
#52355=EDGE_LOOP ( 'NONE', ( #46642, #5302, #9292, #82342 ) ) ;
#52359=CARTESIAN_POINT ( 'NONE',  ( 13.91025641025641235, -11.50000000000000000, 29.75000000000000355 ) ) ;
#52370=CARTESIAN_POINT ( 'NONE',  ( -19.50000000000000000, -3.499999999999999556, 29.75000000000000355 ) ) ;
#52372=DIRECTION ( 'NONE',  ( 0.000000000000000000, 0.000000000000000000, 1.000000000000000000 ) ) ;
#52378=VECTOR ( 'NONE', #61499, 1000.000000000000000 ) ;
#52388=DIRECTION ( 'NONE',  ( -0.000000000000000000, 1.000000000000000000, -0.000000000000000000 ) ) ;
#52393=EDGE_LOOP ( 'NONE', ( #82808, #19993, #5128, #61439 ) ) ;
#52409=ORIENTED_EDGE ( 'NONE', *, *, #32354, .F. ) ;
#52415=VERTEX_POINT ( 'NONE', #26837 ) ;
#52436=ADVANCED_FACE ( 'NONE', ( #6566 ), #35360, .F. ) ;
#52456=LINE ( 'NONE', #80397, #9945 ) ;
#52457=PLANE ( 'NONE',  #10858 ) ;
#52463=EDGE_CURVE ( 'NONE', #7973, #3259, #35818, .T. ) ;
#52467=ORIENTED_EDGE ( 'NONE', *, *, #29772, .F. ) ;
#52479=VERTEX_POINT ( 'NONE', #70927 ) ;
#52498=ORIENTED_EDGE ( 'NONE', *, *, #85811, .T. ) ;
#52503=VECTOR ( 'NONE', #53502, 1000.000000000000000 ) ;
#52513=CARTESIAN_POINT ( 'NONE',  ( 13.19230769230769340, -7.500000000000000000, 33.75000000000000000 ) ) ;
#52529=CARTESIAN_POINT ( 'NONE',  ( -19.50000000000000000, -11.50000000000000000, 29.75000000000000355 ) ) ;
#52534=LINE ( 'NONE', #32280, #37382 ) ;
#52539=DIRECTION ( 'NONE',  ( -0.000000000000000000, 1.000000000000000000, -0.000000000000000000 ) ) ;
#52547=CARTESIAN_POINT ( 'NONE',  ( -19.50000000000000000, -11.50000000000000000, 29.75000000000000355 ) ) ;
#52560=LINE ( 'NONE', #4382, #24058 ) ;
#52570=PLANE ( 'NONE',  #66070 ) ;
#52585=EDGE_CURVE ( 'NONE', #70755, #75080, #60066, .T. ) ;
#52590=EDGE_CURVE ( 'NONE', #12230, #88550, #39812, .T. ) ;
#52599=ORIENTED_EDGE ( 'NONE', *, *, #86362, .T. ) ;
#52600=CARTESIAN_POINT ( 'NONE',  ( -4.230769230769230838, -3.499999999999999556, 29.75000000000000355 ) ) ;
#52601=EDGE_CURVE ( 'NONE', #82878, #57615, #65929, .T. ) ;
#52610=FACE_OUTER_BOUND ( 'NONE', #14935, .T. ) ;
#52613=DIRECTION ( 'NONE',  ( -1.000000000000000000, -0.000000000000000000, -0.000000000000000000 ) ) ;
#52615=EDGE_CURVE ( 'NONE', #59590, #13160, #60549, .T. ) ;
#52626=AXIS2_PLACEMENT_3D ( 'NONE', #53103, #32849, #31964 ) ;
#52636=CARTESIAN_POINT ( 'NONE',  ( -9.320512820512821150, -11.00000000000000000, 29.75000000000000355 ) ) ;
#52641=VERTEX_POINT ( 'NONE', #52861 ) ;
#52648=( NAMED_UNIT ( * ) SI_UNIT ( $, .STERADIAN. ) SOLID_ANGLE_UNIT ( ) );
#52655=PLANE ( 'NONE',  #79063 ) ;
#52677=EDGE_CURVE ( 'NONE', #30150, #51499, #80686, .T. ) ;
#52679=CARTESIAN_POINT ( 'NONE',  ( -3.512820512820513663, -7.500000000000000000, 33.75000000000000000 ) ) ;
#52684=ADVANCED_FACE ( 'NONE', ( #45217 ), #72694, .F. ) ;
#52685=CIRCLE ( 'NONE', #59814, 4.000000000000000000 ) ;
#52688=EDGE_CURVE ( 'NONE', #86305, #82221, #47435, .T. ) ;
#52712=EDGE_CURVE ( 'NONE', #71861, #28699, #56245, .T. ) ;
#52721=LINE ( 'NONE', #60373, #70452 ) ;
#52727=CARTESIAN_POINT ( 'NONE',  ( -9.070512820512819374, -3.499999999999999556, 29.75000000000000355 ) ) ;
#52729=DIRECTION ( 'NONE',  ( 1.000000000000000000, 0.000000000000000000, 0.000000000000000000 ) ) ;
#52737=EDGE_CURVE ( 'NONE', #496, #84195, #21705, .T. ) ;
#52740=DIRECTION ( 'NONE',  ( 1.000000000000000000, 0.000000000000000000, 0.000000000000000000 ) ) ;
#52746=EDGE_CURVE ( 'NONE', #50514, #3262, #17397, .T. ) ;
#52752=ORIENTED_EDGE ( 'NONE', *, *, #9513, .F. ) ;
#52760=FACE_OUTER_BOUND ( 'NONE', #32112, .T. ) ;
#52784=EDGE_CURVE ( 'NONE', #54472, #9433, #14104, .T. ) ;
#52789=DIRECTION ( 'NONE',  ( -1.000000000000000000, -0.000000000000000000, 0.000000000000000000 ) ) ;
#52791=CARTESIAN_POINT ( 'NONE',  ( -18.03205128205128105, -3.499999999999999556, 29.75000000000000355 ) ) ;
#52802=FACE_OUTER_BOUND ( 'NONE', #70806, .T. ) ;
#52809=EDGE_CURVE ( 'NONE', #63742, #52150, #62278, .T. ) ;
#52814=ORIENTED_EDGE ( 'NONE', *, *, #68538, .T. ) ;
#52818=VECTOR ( 'NONE', #40899, 1000.000000000000000 ) ;
#52819=CARTESIAN_POINT ( 'NONE',  ( -16.81410256410256565, -7.500000000000000000, 29.75000000000000355 ) ) ;
#52827=ORIENTED_EDGE ( 'NONE', *, *, #32008, .T. ) ;
#52847=CARTESIAN_POINT ( 'NONE',  ( 0.000000000000000000, -11.00000000000000000, 29.75000000000000355 ) ) ;
#52860=DIRECTION ( 'NONE',  ( -1.000000000000000000, -0.000000000000000000, 0.000000000000000000 ) ) ;
#52861=CARTESIAN_POINT ( 'NONE',  ( 11.97435897435897267, -11.00000000000000000, 29.75000000000000355 ) ) ;
#52880=CARTESIAN_POINT ( 'NONE',  ( -19.50000000000000000, -3.499999999999999556, 29.75000000000000355 ) ) ;
#52887=ORIENTED_EDGE ( 'NONE', *, *, #17513, .F. ) ;
#52895=DIRECTION ( 'NONE',  ( 0.000000000000000000, 0.000000000000000000, -1.000000000000000000 ) ) ;
#52904=PLANE ( 'NONE',  #66610 ) ;
#52917=AXIS2_PLACEMENT_3D ( 'NONE', #10776, #2668, #85994 ) ;
#52941=CIRCLE ( 'NONE', #44317, 4.000000000000000000 ) ;
#52942=CARTESIAN_POINT ( 'NONE',  ( -17.78205128205128105, -3.499999999999999556, 29.75000000000000355 ) ) ;
#52958=LINE ( 'NONE', #47533, #8730 ) ;
#52962=ORIENTED_EDGE ( 'NONE', *, *, #25012, .F. ) ;
#52980=VECTOR ( 'NONE', #42691, 1000.000000000000000 ) ;
#53009=DIRECTION ( 'NONE',  ( -0.000000000000000000, 1.000000000000000000, -0.000000000000000000 ) ) ;
#53011=ORIENTED_EDGE ( 'NONE', *, *, #53808, .T. ) ;
#53028=LINE ( 'NONE', #80531, #80303 ) ;
#53053=DIRECTION ( 'NONE',  ( 0.000000000000000000, 0.000000000000000000, -1.000000000000000000 ) ) ;
#53062=DIRECTION ( 'NONE',  ( -0.000000000000000000, 1.000000000000000000, -0.000000000000000000 ) ) ;
#53073=CARTESIAN_POINT ( 'NONE',  ( -19.50000000000000000, -3.499999999999999556, 29.75000000000000355 ) ) ;
#53074=AXIS2_PLACEMENT_3D ( 'NONE', #75596, #41381, #68846 ) ;
#53076=DIRECTION ( 'NONE',  ( -0.000000000000000000, 1.000000000000000000, -0.000000000000000000 ) ) ;
#53083=DIRECTION ( 'NONE',  ( -1.000000000000000000, -0.000000000000000000, -0.000000000000000000 ) ) ;
#53084=PRESENTATION_STYLE_ASSIGNMENT (( #87805 ) ) ;
#53096=DIRECTION ( 'NONE',  ( 1.000000000000000000, 0.000000000000000000, 0.000000000000000000 ) ) ;
#53103=CARTESIAN_POINT ( 'NONE',  ( 16.09615384615384670, -7.500000000000000000, 29.75000000000000355 ) ) ;
#53121=DIRECTION ( 'NONE',  ( 0.000000000000000000, 0.000000000000000000, -1.000000000000000000 ) ) ;
#53124=DIRECTION ( 'NONE',  ( 0.000000000000000000, 0.000000000000000000, -1.000000000000000000 ) ) ;
#53126=EDGE_CURVE ( 'NONE', #20882, #13118, #32947, .T. ) ;
#53150=ORIENTED_EDGE ( 'NONE', *, *, #73177, .T. ) ;
#53167=AXIS2_PLACEMENT_3D ( 'NONE', #29414, #85236, #16328 ) ;
#53187=CARTESIAN_POINT ( 'NONE',  ( 6.166666666666664298, -3.499999999999999556, 29.75000000000000355 ) ) ;
#53209=CARTESIAN_POINT ( 'NONE',  ( -6.166666666666667851, -11.00000000000000000, 29.75000000000000355 ) ) ;
#53219=LINE ( 'NONE', #38835, #12188 ) ;
#53251=ADVANCED_FACE ( 'NONE', ( #65163 ), #23294, .T. ) ;
#53280=FACE_OUTER_BOUND ( 'NONE', #34575, .T. ) ;
#53285=ORIENTED_EDGE ( 'NONE', *, *, #36201, .T. ) ;
#53292=CARTESIAN_POINT ( 'NONE',  ( 11.25641025641025550, -7.500000000000000000, 29.75000000000000355 ) ) ;
#53299=EDGE_CURVE ( 'NONE', #29827, #16936, #2571, .T. ) ;
#53301=ORIENTED_EDGE ( 'NONE', *, *, #28898, .T. ) ;
#53309=ORIENTED_EDGE ( 'NONE', *, *, #64218, .F. ) ;
#53311=DIRECTION ( 'NONE',  ( 0.000000000000000000, 0.000000000000000000, -1.000000000000000000 ) ) ;
#53328=CARTESIAN_POINT ( 'NONE',  ( 14.16025641025641235, -7.500000000000000000, 33.75000000000000000 ) ) ;
#53347=CARTESIAN_POINT ( 'NONE',  ( -18.03205128205128105, -3.499999999999999556, 29.75000000000000355 ) ) ;
#53361=DIRECTION ( 'NONE',  ( -1.000000000000000000, 0.000000000000000000, -0.000000000000000000 ) ) ;
#53370=DIRECTION ( 'NONE',  ( -1.000000000000000000, -0.000000000000000000, -0.000000000000000000 ) ) ;
#53373=ORIENTED_EDGE ( 'NONE', *, *, #25027, .T. ) ;
#53377=LINE ( 'NONE', #85840, #35862 ) ;
#53378=CARTESIAN_POINT ( 'NONE',  ( 11.97435897435897623, -3.499999999999999556, 29.75000000000000355 ) ) ;
#53381=ORIENTED_EDGE ( 'NONE', *, *, #42861, .T. ) ;
#53389=DIRECTION ( 'NONE',  ( -0.000000000000000000, 1.000000000000000000, -0.000000000000000000 ) ) ;
#53391=VERTEX_POINT ( 'NONE', #38594 ) ;
#53393=VECTOR ( 'NONE', #81806, 1000.000000000000000 ) ;
#53413=AXIS2_PLACEMENT_3D ( 'NONE', #76573, #34701, #56738 ) ;
#53430=EDGE_CURVE ( 'NONE', #24285, #6115, #60184, .T. ) ;
#53465=CARTESIAN_POINT ( 'NONE',  ( -11.00641025641025550, -3.499999999999999556, 29.75000000000000355 ) ) ;
#53483=AXIS2_PLACEMENT_3D ( 'NONE', #59178, #26286, #48324 ) ;
#53497=ORIENTED_EDGE ( 'NONE', *, *, #15907, .T. ) ;
#53502=DIRECTION ( 'NONE',  ( 1.000000000000000000, 0.000000000000000000, 0.000000000000000000 ) ) ;
#53506=DIRECTION ( 'NONE',  ( 0.000000000000000000, 0.000000000000000000, -1.000000000000000000 ) ) ;
#53510=VECTOR ( 'NONE', #22521, 1000.000000000000000 ) ;
#53512=DIRECTION ( 'NONE',  ( 0.000000000000000000, 0.000000000000000000, -1.000000000000000000 ) ) ;
#53515=DIRECTION ( 'NONE',  ( 0.000000000000000000, 0.000000000000000000, -1.000000000000000000 ) ) ;
#53517=EDGE_LOOP ( 'NONE', ( #78075, #7214, #48617, #57042 ) ) ;
#53523=EDGE_CURVE ( 'NONE', #19429, #29827, #20967, .T. ) ;
#53528=DIRECTION ( 'NONE',  ( -1.000000000000000000, -0.000000000000000000, -0.000000000000000000 ) ) ;
#53539=ORIENTED_EDGE ( 'NONE', *, *, #19160, .T. ) ;
#53545=DIRECTION ( 'NONE',  ( 1.000000000000000000, 0.000000000000000000, 0.000000000000000000 ) ) ;
#53557=CIRCLE ( 'NONE', #40647, 4.000000000000000000 ) ;
#53563=AXIS2_PLACEMENT_3D ( 'NONE', #28782, #49494, #29665 ) ;
#53565=CARTESIAN_POINT ( 'NONE',  ( -16.09615384615384670, -3.499999999999999556, 29.75000000000000355 ) ) ;
#53573=ORIENTED_EDGE ( 'NONE', *, *, #22708, .T. ) ;
#53577=DIRECTION ( 'NONE',  ( 0.000000000000000000, 0.000000000000000000, -1.000000000000000000 ) ) ;
#53592=DIRECTION ( 'NONE',  ( -0.000000000000000000, 0.000000000000000000, 1.000000000000000000 ) ) ;
#53595=DIRECTION ( 'NONE',  ( -0.000000000000000000, 1.000000000000000000, -0.000000000000000000 ) ) ;
#53603=ORIENTED_EDGE ( 'NONE', *, *, #23999, .T. ) ;
#53605=ORIENTED_EDGE ( 'NONE', *, *, #84059, .T. ) ;
#53610=ORIENTED_EDGE ( 'NONE', *, *, #13385, .F. ) ;
#53616=VERTEX_POINT ( 'NONE', #56541 ) ;
#53617=CIRCLE ( 'NONE', #26299, 4.000000000000000000 ) ;
#53639=LINE ( 'NONE', #81569, #25007 ) ;
#53641=DIRECTION ( 'NONE',  ( -1.000000000000000000, -0.000000000000000000, -0.000000000000000000 ) ) ;
#53642=VERTEX_POINT ( 'NONE', #22745 ) ;
#53657=PLANE ( 'NONE',  #53907 ) ;
#53659=DIRECTION ( 'NONE',  ( -0.000000000000000000, 1.000000000000000000, -0.000000000000000000 ) ) ;
#53662=CIRCLE ( 'NONE', #68014, 4.000000000000000000 ) ;
#53664=ORIENTED_EDGE ( 'NONE', *, *, #866, .T. ) ;
#53683=AXIS2_PLACEMENT_3D ( 'NONE', #70386, #15446, #8691 ) ;
#53685=DIRECTION ( 'NONE',  ( 1.000000000000000000, 0.000000000000000000, 0.000000000000000000 ) ) ;
#53689=EDGE_CURVE ( 'NONE', #47713, #87461, #41907, .T. ) ;
#53690=CYLINDRICAL_SURFACE ( 'NONE', #58451, 4.000000000000000000 ) ;
#53695=ORIENTED_EDGE ( 'NONE', *, *, #78372, .T. ) ;
#53704=FACE_OUTER_BOUND ( 'NONE', #11334, .T. ) ;
#53705=AXIS2_PLACEMENT_3D ( 'NONE', #86424, #24695, #47632 ) ;
#53737=EDGE_CURVE ( 'NONE', #23542, #13174, #14509, .T. ) ;
#53759=DIRECTION ( 'NONE',  ( 0.000000000000000000, 0.000000000000000000, 1.000000000000000000 ) ) ;
#53775=AXIS2_PLACEMENT_3D ( 'NONE', #41217, #61034, #88536 ) ;
#53786=ORIENTED_EDGE ( 'NONE', *, *, #43956, .T. ) ;
#53792=CARTESIAN_POINT ( 'NONE',  ( -19.50000000000000000, -3.499999999999999556, 29.75000000000000355 ) ) ;
#53794=LINE ( 'NONE', #81285, #5139 ) ;
#53808=EDGE_CURVE ( 'NONE', #29864, #80082, #70794, .T. ) ;
#53825=VERTEX_POINT ( 'NONE', #77541 ) ;
#53828=ORIENTED_EDGE ( 'NONE', *, *, #48136, .T. ) ;
#53841=VERTEX_POINT ( 'NONE', #22593 ) ;
#53846=EDGE_LOOP ( 'NONE', ( #31228, #66085, #19216, #45403 ) ) ;
#53855=LINE ( 'NONE', #34469, #80167 ) ;
#53857=CARTESIAN_POINT ( 'NONE',  ( 14.87820512820512953, -7.500000000000000000, 29.75000000000000355 ) ) ;
#53863=CARTESIAN_POINT ( 'NONE',  ( -6.416666666666667851, -3.499999999999999556, 29.75000000000000355 ) ) ;
#53866=CARTESIAN_POINT ( 'NONE',  ( 20.00000000000000000, -4.000000000000000000, 29.75000000000000355 ) ) ;
#53884=EDGE_LOOP ( 'NONE', ( #57619, #32233, #58428, #51782 ) ) ;
#53890=ORIENTED_EDGE ( 'NONE', *, *, #78124, .F. ) ;
#53902=CARTESIAN_POINT ( 'NONE',  ( -19.50000000000000000, -3.499999999999999556, 29.75000000000000355 ) ) ;
#53904=LINE ( 'NONE', #39963, #62855 ) ;
#53907=AXIS2_PLACEMENT_3D ( 'NONE', #73941, #26189, #12676 ) ;
#53914=ORIENTED_EDGE ( 'NONE', *, *, #3448, .F. ) ;
#53918=ORIENTED_EDGE ( 'NONE', *, *, #46501, .T. ) ;
#53934=ORIENTED_EDGE ( 'NONE', *, *, #32395, .F. ) ;
#53936=ORIENTED_EDGE ( 'NONE', *, *, #30402, .T. ) ;
#53939=CARTESIAN_POINT ( 'NONE',  ( 0.6089743589743589203, -11.50000000000000000, 29.75000000000000355 ) ) ;
#53942=EDGE_CURVE ( 'NONE', #37401, #50277, #7154, .T. ) ;
#53945=VERTEX_POINT ( 'NONE', #73850 ) ;
#53955=EDGE_CURVE ( 'NONE', #51834, #39901, #39629, .T. ) ;
#53958=LINE ( 'NONE', #67924, #26706 ) ;
#53960=CARTESIAN_POINT ( 'NONE',  ( 20.00000000000000000, -4.000000000000000000, 29.75000000000000355 ) ) ;
#53965=CARTESIAN_POINT ( 'NONE',  ( -18.75000000000000000, -7.500000000000000000, 29.75000000000000355 ) ) ;
#53967=VERTEX_POINT ( 'NONE', #5826 ) ;
#53983=DIRECTION ( 'NONE',  ( 1.000000000000000000, 0.000000000000000000, 0.000000000000000000 ) ) ;
#54015=CARTESIAN_POINT ( 'NONE',  ( -6.166666666666667851, -7.500000000000000000, 29.75000000000000355 ) ) ;
#54025=ORIENTED_EDGE ( 'NONE', *, *, #17480, .T. ) ;
#54038=EDGE_LOOP ( 'NONE', ( #72332, #12684, #50587, #17668 ) ) ;
#54040=DIRECTION ( 'NONE',  ( 1.000000000000000000, 0.000000000000000000, 0.000000000000000000 ) ) ;
#54044=CARTESIAN_POINT ( 'NONE',  ( -8.352564102564102200, -4.000000000000000000, 29.75000000000000355 ) ) ;
#54060=CARTESIAN_POINT ( 'NONE',  ( -12.22435897435897267, -7.500000000000000000, 29.75000000000000355 ) ) ;
#54061=CARTESIAN_POINT ( 'NONE',  ( 9.070512820512819374, -11.50000000000000000, 29.75000000000000355 ) ) ;
#54068=LINE ( 'NONE', #13538, #76446 ) ;
#54074=VECTOR ( 'NONE', #5588, 1000.000000000000000 ) ;
#54079=EDGE_CURVE ( 'NONE', #86419, #55273, #71063, .T. ) ;
#54108=FACE_OUTER_BOUND ( 'NONE', #28691, .T. ) ;
#54120=EDGE_LOOP ( 'NONE', ( #61767, #12871, #24086, #33239 ) ) ;
#54125=ORIENTED_EDGE ( 'NONE', *, *, #13667, .F. ) ;
#54140=ORIENTED_EDGE ( 'NONE', *, *, #17869, .T. ) ;
#54141=LINE ( 'NONE', #68996, #88939 ) ;
#54153=ORIENTED_EDGE ( 'NONE', *, *, #13358, .T. ) ;
#54155=EDGE_CURVE ( 'NONE', #3262, #37853, #11137, .T. ) ;
#54157=CARTESIAN_POINT ( 'NONE',  ( -3.262820512820514107, -7.500000000000000000, 29.75000000000000355 ) ) ;
#54163=DIRECTION ( 'NONE',  ( -1.000000000000000000, -0.000000000000000000, -0.000000000000000000 ) ) ;
#54173=CARTESIAN_POINT ( 'NONE',  ( -8.352564102564102200, -3.499999999999999556, 29.75000000000000355 ) ) ;
#54174=LINE ( 'NONE', #47420, #1051 ) ;
#54186=DIRECTION ( 'NONE',  ( -1.000000000000000000, -0.000000000000000000, -0.000000000000000000 ) ) ;
#54200=DIRECTION ( 'NONE',  ( 1.000000000000000000, -0.000000000000000000, 0.000000000000000000 ) ) ;
#54207=AXIS2_PLACEMENT_3D ( 'NONE', #18361, #85929, #79617 ) ;
#54208=LINE ( 'NONE', #74950, #75441 ) ;
#54210=DIRECTION ( 'NONE',  ( 1.000000000000000000, 0.000000000000000000, 0.000000000000000000 ) ) ;
#54242=DIRECTION ( 'NONE',  ( 1.000000000000000000, 0.000000000000000000, 0.000000000000000000 ) ) ;
#54243=CARTESIAN_POINT ( 'NONE',  ( -15.84615384615384670, -7.500000000000000000, 33.75000000000000000 ) ) ;
#54263=EDGE_LOOP ( 'NONE', ( #88437, #29967, #7921, #89164, #85082 ) ) ;
#54289=AXIS2_PLACEMENT_3D ( 'NONE', #38585, #44882, #45778 ) ;
#54295=CARTESIAN_POINT ( 'NONE',  ( -19.50000000000000000, -11.50000000000000000, 29.75000000000000355 ) ) ;
#54326=PLANE ( 'NONE',  #26827 ) ;
#54353=EDGE_CURVE ( 'NONE', #26695, #23520, #70525, .T. ) ;
#54375=VECTOR ( 'NONE', #81623, 1000.000000000000000 ) ;
#54385=ORIENTED_EDGE ( 'NONE', *, *, #30456, .T. ) ;
#54390=ORIENTED_EDGE ( 'NONE', *, *, #12281, .T. ) ;
#54404=LINE ( 'NONE', #81899, #9483 ) ;
#54412=LINE ( 'NONE', #73819, #64522 ) ;
#54413=DIRECTION ( 'NONE',  ( 0.000000000000000000, 0.000000000000000000, 1.000000000000000000 ) ) ;
#54429=AXIS2_PLACEMENT_3D ( 'NONE', #77682, #49766, #15550 ) ;
#54436=CARTESIAN_POINT ( 'NONE',  ( -19.50000000000000000, -3.499999999999999556, 29.75000000000000355 ) ) ;
#54452=FACE_BOUND ( 'NONE', #44616, .T. ) ;
#54458=EDGE_CURVE ( 'NONE', #78293, #36536, #64632, .T. ) ;
#54464=ORIENTED_EDGE ( 'NONE', *, *, #51318, .T. ) ;
#54472=VERTEX_POINT ( 'NONE', #72288 ) ;
#54484=ORIENTED_EDGE ( 'NONE', *, *, #10311, .T. ) ;
#54485=ORIENTED_EDGE ( 'NONE', *, *, #22053, .F. ) ;
#54499=CIRCLE ( 'NONE', #70325, 4.000000000000000000 ) ;
#54505=CARTESIAN_POINT ( 'NONE',  ( 5.198717948717946236, -7.500000000000000000, 29.75000000000000355 ) ) ;
#54515=EDGE_LOOP ( 'NONE', ( #74162, #22811, #63140, #24343 ) ) ;
#54533=ORIENTED_EDGE ( 'NONE', *, *, #2890, .F. ) ;
#54542=VERTEX_POINT ( 'NONE', #51111 ) ;
#54552=DIRECTION ( 'NONE',  ( 0.000000000000000000, 0.000000000000000000, -1.000000000000000000 ) ) ;
#54555=VECTOR ( 'NONE', #57291, 1000.000000000000000 ) ;
#54556=VECTOR ( 'NONE', #80986, 1000.000000000000000 ) ;
#54562=VECTOR ( 'NONE', #89094, 1000.000000000000000 ) ;
#54566=DIRECTION ( 'NONE',  ( 0.000000000000000000, 0.000000000000000000, -1.000000000000000000 ) ) ;
#54573=DIRECTION ( 'NONE',  ( -1.000000000000000000, -0.000000000000000000, -0.000000000000000000 ) ) ;
#54611=VECTOR ( 'NONE', #45898, 1000.000000000000000 ) ;
#54620=ORIENTED_EDGE ( 'NONE', *, *, #88036, .T. ) ;
#54655=ORIENTED_EDGE ( 'NONE', *, *, #73718, .F. ) ;
#54656=LINE ( 'NONE', #82608, #1627 ) ;
#54658=EDGE_CURVE ( 'NONE', #60613, #51834, #60111, .T. ) ;
#54670=DIRECTION ( 'NONE',  ( 0.000000000000000000, 0.000000000000000000, 1.000000000000000000 ) ) ;
#54682=VERTEX_POINT ( 'NONE', #67764 ) ;
#54693=CARTESIAN_POINT ( 'NONE',  ( 7.134615384615385025, -3.499999999999999556, 29.75000000000000355 ) ) ;
#54712=VECTOR ( 'NONE', #42608, 1000.000000000000000 ) ;
#54718=ORIENTED_EDGE ( 'NONE', *, *, #17708, .T. ) ;
#54739=DIRECTION ( 'NONE',  ( -1.000000000000000000, -0.000000000000000000, -0.000000000000000000 ) ) ;
#54769=DIRECTION ( 'NONE',  ( 0.000000000000000000, 0.000000000000000000, -1.000000000000000000 ) ) ;
#54773=EDGE_CURVE ( 'NONE', #59060, #64127, #79393, .T. ) ;
#54775=DIRECTION ( 'NONE',  ( -1.000000000000000000, -0.000000000000000000, 0.000000000000000000 ) ) ;
#54792=CARTESIAN_POINT ( 'NONE',  ( -19.50000000000000000, -11.50000000000000000, 29.75000000000000355 ) ) ;
#54804=AXIS2_PLACEMENT_3D ( 'NONE', #83370, #41489, #68957 ) ;
#54821=ORIENTED_EDGE ( 'NONE', *, *, #48086, .F. ) ;
#54825=FACE_OUTER_BOUND ( 'NONE', #86196, .T. ) ;
#54826=EDGE_CURVE ( 'NONE', #7446, #45168, #70771, .T. ) ;
#54831=DIRECTION ( 'NONE',  ( -1.000000000000000000, -0.000000000000000000, 0.000000000000000000 ) ) ;
#54834=ORIENTED_EDGE ( 'NONE', *, *, #79424, .T. ) ;
#54838=VERTEX_POINT ( 'NONE', #29879 ) ;
#54840=VECTOR ( 'NONE', #48161, 1000.000000000000000 ) ;
#54841=EDGE_CURVE ( 'NONE', #57687, #19139, #63652, .T. ) ;
#54843=ORIENTED_EDGE ( 'NONE', *, *, #34410, .F. ) ;
#54845=PLANE ( 'NONE',  #71001 ) ;
#54846=CARTESIAN_POINT ( 'NONE',  ( 4.480769230769229061, -7.500000000000000000, 29.75000000000000355 ) ) ;
#54873=CARTESIAN_POINT ( 'NONE',  ( -14.16025641025641058, -7.500000000000000000, 29.75000000000000355 ) ) ;
#54904=DIRECTION ( 'NONE',  ( -0.000000000000000000, 0.000000000000000000, 1.000000000000000000 ) ) ;
#54908=ORIENTED_EDGE ( 'NONE', *, *, #31627, .F. ) ;
#54913=DIRECTION ( 'NONE',  ( -0.000000000000000000, 0.000000000000000000, 1.000000000000000000 ) ) ;
#54916=CIRCLE ( 'NONE', #20386, 4.000000000000000000 ) ;
#54933=ADVANCED_FACE ( 'NONE', ( #13483 ), #13044, .F. ) ;
#54941=VECTOR ( 'NONE', #51738, 1000.000000000000000 ) ;
#54950=LINE ( 'NONE', #13957, #75622 ) ;
#54958=DIRECTION ( 'NONE',  ( -0.000000000000000000, 1.000000000000000000, -0.000000000000000000 ) ) ;
#54962=LINE ( 'NONE', #41901, #22262 ) ;
#54963=DIRECTION ( 'NONE',  ( 0.000000000000000000, 0.000000000000000000, 1.000000000000000000 ) ) ;
#55000=EDGE_CURVE ( 'NONE', #4543, #427, #69355, .T. ) ;
#55021=CIRCLE ( 'NONE', #78025, 4.000000000000000000 ) ;
#55022=CARTESIAN_POINT ( 'NONE',  ( -10.28846153846153832, -3.499999999999999556, 29.75000000000000355 ) ) ;
#55033=( LENGTH_UNIT ( ) NAMED_UNIT ( * ) SI_UNIT ( .MILLI., .METRE. ) );
#55036=CARTESIAN_POINT ( 'NONE',  ( 3.512820512820510555, -3.499999999999999556, 29.75000000000000355 ) ) ;
#55046=FACE_OUTER_BOUND ( 'NONE', #88641, .T. ) ;
#55049=VERTEX_POINT ( 'NONE', #42298 ) ;
#55050=ORIENTED_EDGE ( 'NONE', *, *, #64218, .T. ) ;
#55054=CARTESIAN_POINT ( 'NONE',  ( -6.416666666666667851, -3.499999999999999556, 29.75000000000000355 ) ) ;
#55061=DIRECTION ( 'NONE',  ( 1.000000000000000000, 0.000000000000000000, 0.000000000000000000 ) ) ;
#55066=ORIENTED_EDGE ( 'NONE', *, *, #23002, .T. ) ;
#55084=FACE_OUTER_BOUND ( 'NONE', #41803, .T. ) ;
#55086=DIRECTION ( 'NONE',  ( 1.000000000000000000, 0.000000000000000000, 0.000000000000000000 ) ) ;
#55104=ADVANCED_FACE ( 'NONE', ( #50787 ), #56244, .T. ) ;
#55140=CARTESIAN_POINT ( 'NONE',  ( 0.000000000000000000, -11.00000000000000000, 29.75000000000000355 ) ) ;
#55156=ORIENTED_EDGE ( 'NONE', *, *, #22729, .T. ) ;
#55161=EDGE_CURVE ( 'NONE', #16151, #30233, #3185, .T. ) ;
#55166=ORIENTED_EDGE ( 'NONE', *, *, #19926, .F. ) ;
#55174=VECTOR ( 'NONE', #10631, 1000.000000000000000 ) ;
#55177=DIRECTION ( 'NONE',  ( -0.000000000000000000, 1.000000000000000000, -0.000000000000000000 ) ) ;
#55182=DIRECTION ( 'NONE',  ( -1.000000000000000000, -0.000000000000000000, 0.000000000000000000 ) ) ;
#55218=DIRECTION ( 'NONE',  ( -0.000000000000000000, 1.000000000000000000, -0.000000000000000000 ) ) ;
#55231=DIRECTION ( 'NONE',  ( -1.000000000000000000, 0.000000000000000000, -0.000000000000000000 ) ) ;
#55235=ORIENTED_EDGE ( 'NONE', *, *, #47631, .F. ) ;
#55262=EDGE_LOOP ( 'NONE', ( #86858, #17832, #62279, #35678, #62760 ) ) ;
#55266=PLANE ( 'NONE',  #14254 ) ;
#55273=VERTEX_POINT ( 'NONE', #53465 ) ;
#55275=ORIENTED_EDGE ( 'NONE', *, *, #82150, .T. ) ;
#55278=ORIENTED_EDGE ( 'NONE', *, *, #31527, .F. ) ;
#55284=DIRECTION ( 'NONE',  ( 1.000000000000000000, 0.000000000000000000, 0.000000000000000000 ) ) ;
#55300=EDGE_LOOP ( 'NONE', ( #42990, #74941, #51634, #44179, #2519 ) ) ;
#55328=LINE ( 'NONE', #1268, #71211 ) ;
#55336=DIRECTION ( 'NONE',  ( -1.000000000000000000, 0.000000000000000000, -0.000000000000000000 ) ) ;
#55350=DIRECTION ( 'NONE',  ( 0.000000000000000000, 0.000000000000000000, -1.000000000000000000 ) ) ;
#55353=EDGE_CURVE ( 'NONE', #51205, #85537, #69642, .T. ) ;
#55359=ADVANCED_FACE ( 'NONE', ( #36745 ), #8393, .F. ) ;
#55380=VECTOR ( 'NONE', #56003, 1000.000000000000000 ) ;
#55403=ORIENTED_EDGE ( 'NONE', *, *, #27739, .T. ) ;
#55405=VECTOR ( 'NONE', #37265, 1000.000000000000000 ) ;
#55419=DIRECTION ( 'NONE',  ( -0.000000000000000000, 1.000000000000000000, -0.000000000000000000 ) ) ;
#55429=LINE ( 'NONE', #9459, #88364 ) ;
#55445=EDGE_CURVE ( 'NONE', #81881, #58148, #42190, .T. ) ;
#55449=LINE ( 'NONE', #21218, #24630 ) ;
#55462=LINE ( 'NONE', #83396, #20627 ) ;
#55463=ORIENTED_EDGE ( 'NONE', *, *, #67995, .F. ) ;
#55465=EDGE_CURVE ( 'NONE', #18250, #55647, #4291, .T. ) ;
#55469=CIRCLE ( 'NONE', #78674, 4.000000000000000000 ) ;
#55477=DIRECTION ( 'NONE',  ( 0.000000000000000000, 0.000000000000000000, -1.000000000000000000 ) ) ;
#55494=ORIENTED_EDGE ( 'NONE', *, *, #60417, .T. ) ;
#55497=EDGE_CURVE ( 'NONE', #86970, #5565, #38076, .T. ) ;
#55525=CYLINDRICAL_SURFACE ( 'NONE', #63415, 4.000000000000000000 ) ;
#55534=ORIENTED_EDGE ( 'NONE', *, *, #59719, .T. ) ;
#55547=CARTESIAN_POINT ( 'NONE',  ( 14.16025641025641235, -4.000000000000000000, 29.75000000000000355 ) ) ;
#55554=CARTESIAN_POINT ( 'NONE',  ( -8.352564102564102200, -11.00000000000000000, 29.75000000000000355 ) ) ;
#55556=DIRECTION ( 'NONE',  ( 0.000000000000000000, 0.000000000000000000, -1.000000000000000000 ) ) ;
#55571=ORIENTED_EDGE ( 'NONE', *, *, #89074, .F. ) ;
#55574=DIRECTION ( 'NONE',  ( -1.000000000000000000, 0.000000000000000000, -0.000000000000000000 ) ) ;
#55588=DIRECTION ( 'NONE',  ( 1.000000000000000000, 0.000000000000000000, 0.000000000000000000 ) ) ;
#55597=EDGE_CURVE ( 'NONE', #7139, #49175, #55021, .T. ) ;
#55612=PLANE ( 'NONE',  #63521 ) ;
#55627=LINE ( 'NONE', #34914, #18398 ) ;
#55629=ORIENTED_EDGE ( 'NONE', *, *, #79741, .T. ) ;
#55632=DIRECTION ( 'NONE',  ( 0.000000000000000000, 0.000000000000000000, -1.000000000000000000 ) ) ;
#55640=DIRECTION ( 'NONE',  ( -0.000000000000000000, 1.000000000000000000, -0.000000000000000000 ) ) ;
#55647=VERTEX_POINT ( 'NONE', #74094 ) ;
#55653=ORIENTED_EDGE ( 'NONE', *, *, #8635, .F. ) ;
#55654=LINE ( 'NONE', #34063, #3805 ) ;
#55660=LINE ( 'NONE', #286, #68900 ) ;
#55668=DIRECTION ( 'NONE',  ( 1.000000000000000000, 0.000000000000000000, 0.000000000000000000 ) ) ;
#55674=DIRECTION ( 'NONE',  ( 0.000000000000000000, 0.000000000000000000, -1.000000000000000000 ) ) ;
#55679=ADVANCED_FACE ( 'NONE', ( #74532 ), #60120, .F. ) ;
#55685=EDGE_CURVE ( 'NONE', #24805, #1012, #33100, .T. ) ;
#55691=FACE_OUTER_BOUND ( 'NONE', #71864, .T. ) ;
#55699=EDGE_CURVE ( 'NONE', #37657, #48658, #12827, .T. ) ;
#55705=ORIENTED_EDGE ( 'NONE', *, *, #18193, .F. ) ;
#55750=DIRECTION ( 'NONE',  ( -1.000000000000000000, 0.000000000000000000, -0.000000000000000000 ) ) ;
#55773=DIRECTION ( 'NONE',  ( 1.000000000000000000, 0.000000000000000000, 0.000000000000000000 ) ) ;
#55782=ORIENTED_EDGE ( 'NONE', *, *, #24656, .F. ) ;
#55785=VERTEX_POINT ( 'NONE', #69103 ) ;
#55789=EDGE_CURVE ( 'NONE', #75410, #4576, #70437, .T. ) ;
#55793=CARTESIAN_POINT ( 'NONE',  ( 10.28846153846153832, -3.499999999999999556, 29.75000000000000355 ) ) ;
#55794=ORIENTED_EDGE ( 'NONE', *, *, #45969, .F. ) ;
#55807=EDGE_CURVE ( 'NONE', #74851, #46484, #59315, .T. ) ;
#55808=CARTESIAN_POINT ( 'NONE',  ( 18.03205128205128105, -4.000000000000000000, 29.75000000000000355 ) ) ;
#55822=ADVANCED_FACE ( 'NONE', ( #49710 ), #63666, .F. ) ;
#55842=CARTESIAN_POINT ( 'NONE',  ( 0.000000000000000000, -11.00000000000000000, 29.75000000000000355 ) ) ;
#55847=ORIENTED_EDGE ( 'NONE', *, *, #17513, .T. ) ;
#55849=CARTESIAN_POINT ( 'NONE',  ( -9.320512820512821150, -3.499999999999999556, 29.75000000000000355 ) ) ;
#55858=PLANE ( 'NONE',  #81898 ) ;
#55872=CYLINDRICAL_SURFACE ( 'NONE', #25891, 4.000000000000000000 ) ;
#55875=ORIENTED_EDGE ( 'NONE', *, *, #46089, .T. ) ;
#55879=FACE_OUTER_BOUND ( 'NONE', #31431, .T. ) ;
#55916=ADVANCED_FACE ( 'NONE', ( #24892 ), #29892, .F. ) ;
#55917=AXIS2_PLACEMENT_3D ( 'NONE', #32702, #39926, #18313 ) ;
#55946=ORIENTED_EDGE ( 'NONE', *, *, #26750, .T. ) ;
#55969=VECTOR ( 'NONE', #21702, 1000.000000000000000 ) ;
#55977=FACE_OUTER_BOUND ( 'NONE', #44217, .T. ) ;
#55979=VECTOR ( 'NONE', #87770, 1000.000000000000000 ) ;
#55984=EDGE_LOOP ( 'NONE', ( #13958, #26300, #53373, #54140, #70511 ) ) ;
#56003=DIRECTION ( 'NONE',  ( -1.000000000000000000, -0.000000000000000000, 0.000000000000000000 ) ) ;
#56010=CARTESIAN_POINT ( 'NONE',  ( -8.102564102564102200, -3.499999999999999556, 29.75000000000000355 ) ) ;
#56028=CARTESIAN_POINT ( 'NONE',  ( -0.6089743589743593644, -7.500000000000000000, 29.75000000000000355 ) ) ;
#56036=DIRECTION ( 'NONE',  ( 0.000000000000000000, 0.000000000000000000, -1.000000000000000000 ) ) ;
#56062=DIRECTION ( 'NONE',  ( 0.000000000000000000, 0.000000000000000000, -1.000000000000000000 ) ) ;
#56073=LINE ( 'NONE', #49321, #76484 ) ;
#56092=AXIS2_PLACEMENT_3D ( 'NONE', #49189, #43759, #9527 ) ;
#56095=FACE_OUTER_BOUND ( 'NONE', #2237, .T. ) ;
#56101=VECTOR ( 'NONE', #5685, 1000.000000000000000 ) ;
#56114=CIRCLE ( 'NONE', #24463, 4.000000000000000000 ) ;
#56116=CARTESIAN_POINT ( 'NONE',  ( 12.22435897435897267, -11.00000000000000000, 29.75000000000000355 ) ) ;
#56126=EDGE_CURVE ( 'NONE', #58001, #58140, #537, .T. ) ;
#56139=VECTOR ( 'NONE', #48014, 1000.000000000000000 ) ;
#56155=EDGE_LOOP ( 'NONE', ( #82364, #985, #33672, #4866 ) ) ;
#56156=LINE ( 'NONE', #82755, #5696 ) ;
#56159=CARTESIAN_POINT ( 'NONE',  ( -8.102564102564102200, -7.500000000000000000, 29.75000000000000355 ) ) ;
#56162=VECTOR ( 'NONE', #58322, 1000.000000000000000 ) ;
#56193=DIRECTION ( 'NONE',  ( -1.000000000000000000, -0.000000000000000000, -0.000000000000000000 ) ) ;
#56198=CARTESIAN_POINT ( 'NONE',  ( -12.94230769230769162, -11.50000000000000000, 29.75000000000000355 ) ) ;
#56208=ORIENTED_EDGE ( 'NONE', *, *, #65273, .T. ) ;
#56221=DIRECTION ( 'NONE',  ( -1.000000000000000000, -0.000000000000000000, -0.000000000000000000 ) ) ;
#56239=CARTESIAN_POINT ( 'NONE',  ( -3.262820512820514107, -3.499999999999999556, 29.75000000000000355 ) ) ;
#56244=CYLINDRICAL_SURFACE ( 'NONE', #6036, 4.000000000000000000 ) ;
#56245=CIRCLE ( 'NONE', #15991, 4.000000000000000000 ) ;
#56246=FACE_OUTER_BOUND ( 'NONE', #30546, .T. ) ;
#56248=EDGE_LOOP ( 'NONE', ( #72670, #87397, #16525, #8651 ) ) ;
#56268=ORIENTED_EDGE ( 'NONE', *, *, #26522, .F. ) ;
#56276=ORIENTED_EDGE ( 'NONE', *, *, #42871, .F. ) ;
#56286=VECTOR ( 'NONE', #74697, 1000.000000000000000 ) ;
#56287=ADVANCED_FACE ( 'NONE', ( #9074 ), #63992, .F. ) ;
#56297=AXIS2_PLACEMENT_3D ( 'NONE', #84913, #37146, #2908 ) ;
#56322=DIRECTION ( 'NONE',  ( 0.000000000000000000, 0.000000000000000000, 1.000000000000000000 ) ) ;
#56342=EDGE_CURVE ( 'NONE', #43796, #75345, #5864, .T. ) ;
#56350=CARTESIAN_POINT ( 'NONE',  ( -3.262820512820514995, -4.000000000000000000, 29.75000000000000355 ) ) ;
#56364=DIRECTION ( 'NONE',  ( -0.000000000000000000, 1.000000000000000000, -0.000000000000000000 ) ) ;
#56366=CARTESIAN_POINT ( 'NONE',  ( 4.230769230769229061, -3.499999999999999556, 29.75000000000000355 ) ) ;
#56370=CARTESIAN_POINT ( 'NONE',  ( -20.00000000000000000, -11.50000000000000000, 29.75000000000000355 ) ) ;
#56414=CARTESIAN_POINT ( 'NONE',  ( -10.03846153846153832, -3.499999999999999556, 29.75000000000000355 ) ) ;
#56436=CARTESIAN_POINT ( 'NONE',  ( -16.81410256410256565, -3.499999999999999556, 29.75000000000000355 ) ) ;
#56442=LINE ( 'NONE', #68623, #42094 ) ;
#56448=EDGE_LOOP ( 'NONE', ( #62901, #60539, #83076, #87951 ) ) ;
#56453=DIRECTION ( 'NONE',  ( 1.000000000000000000, 0.000000000000000000, 0.000000000000000000 ) ) ;
#56480=EDGE_LOOP ( 'NONE', ( #67663, #86711, #21947, #41288, #681 ) ) ;
#56481=ADVANCED_FACE ( 'NONE', ( #7190 ), #78183, .F. ) ;
#56492=ORIENTED_EDGE ( 'NONE', *, *, #5941, .F. ) ;
#56495=CARTESIAN_POINT ( 'NONE',  ( 9.320512820512821150, -11.50000000000000000, 29.75000000000000355 ) ) ;
#56504=EDGE_LOOP ( 'NONE', ( #62551, #66584, #41262, #88628 ) ) ;
#56511=AXIS2_PLACEMENT_3D ( 'NONE', #82493, #75283, #6390 ) ;
#56533=DIRECTION ( 'NONE',  ( -1.000000000000000000, -0.000000000000000000, -0.000000000000000000 ) ) ;
#56541=CARTESIAN_POINT ( 'NONE',  ( -10.03846153846153832, -4.000000000000000000, 28.25000000000000000 ) ) ;
#56571=EDGE_CURVE ( 'NONE', #4984, #53967, #51567, .T. ) ;
#56580=VECTOR ( 'NONE', #7074, 1000.000000000000000 ) ;
#56602=DIRECTION ( 'NONE',  ( 1.000000000000000000, 0.000000000000000000, 0.000000000000000000 ) ) ;
#56605=ORIENTED_EDGE ( 'NONE', *, *, #2631, .F. ) ;
#56613=DIRECTION ( 'NONE',  ( 0.000000000000000000, 0.000000000000000000, -1.000000000000000000 ) ) ;
#56615=EDGE_CURVE ( 'NONE', #27341, #856, #53662, .T. ) ;
#56618=LINE ( 'NONE', #76453, #33595 ) ;
#56630=ORIENTED_EDGE ( 'NONE', *, *, #83250, .T. ) ;
#56636=DIRECTION ( 'NONE',  ( 1.000000000000000000, 0.000000000000000000, 0.000000000000000000 ) ) ;
#56648=EDGE_LOOP ( 'NONE', ( #23255, #36688, #16812, #61860 ) ) ;
#56661=FACE_OUTER_BOUND ( 'NONE', #76343, .T. ) ;
#56671=VECTOR ( 'NONE', #85172, 1000.000000000000000 ) ;
#56683=CARTESIAN_POINT ( 'NONE',  ( -16.09615384615384670, -7.500000000000000000, 29.75000000000000355 ) ) ;
#56708=ORIENTED_EDGE ( 'NONE', *, *, #35687, .T. ) ;
#56720=LINE ( 'NONE', #58041, #30687 ) ;
#56721=DIRECTION ( 'NONE',  ( -1.000000000000000000, -0.000000000000000000, -0.000000000000000000 ) ) ;
#56729=LINE ( 'NONE', #63918, #11492 ) ;
#56738=DIRECTION ( 'NONE',  ( -1.000000000000000000, 0.000000000000000000, -0.000000000000000000 ) ) ;
#56753=EDGE_LOOP ( 'NONE', ( #46631, #39575, #15169, #53605 ) ) ;
#56777=LINE ( 'NONE', #35636, #66317 ) ;
#56784=EDGE_CURVE ( 'NONE', #15438, #34255, #32123, .T. ) ;
#56793=EDGE_CURVE ( 'NONE', #21434, #83848, #64110, .T. ) ;
#56797=ORIENTED_EDGE ( 'NONE', *, *, #25275, .T. ) ;
#56809=CARTESIAN_POINT ( 'NONE',  ( 0.000000000000000000, -11.00000000000000000, 29.75000000000000355 ) ) ;
#56814=VECTOR ( 'NONE', #52613, 1000.000000000000000 ) ;
#56816=VERTEX_POINT ( 'NONE', #8751 ) ;
#56827=EDGE_CURVE ( 'NONE', #73862, #85779, #82281, .T. ) ;
#56829=EDGE_CURVE ( 'NONE', #4690, #71093, #63229, .T. ) ;
#56849=CARTESIAN_POINT ( 'NONE',  ( -19.50000000000000000, -11.50000000000000000, 29.75000000000000355 ) ) ;
#56873=CARTESIAN_POINT ( 'NONE',  ( 1.576923076923075762, -7.500000000000000000, 29.75000000000000355 ) ) ;
#56874=DIRECTION ( 'NONE',  ( -0.000000000000000000, 1.000000000000000000, -0.000000000000000000 ) ) ;
#56886=DIRECTION ( 'NONE',  ( -1.000000000000000000, -0.000000000000000000, -0.000000000000000000 ) ) ;
#56891=CARTESIAN_POINT ( 'NONE',  ( 0.000000000000000000, -11.00000000000000000, 29.75000000000000355 ) ) ;
#56894=DIRECTION ( 'NONE',  ( -1.000000000000000000, -0.000000000000000000, 0.000000000000000000 ) ) ;
#56919=VECTOR ( 'NONE', #15636, 1000.000000000000000 ) ;
#56938=VECTOR ( 'NONE', #22883, 1000.000000000000000 ) ;
#56951=CARTESIAN_POINT ( 'NONE',  ( -8.102564102564102200, -7.500000000000000000, 29.75000000000000355 ) ) ;
#56953=ORIENTED_EDGE ( 'NONE', *, *, #5376, .T. ) ;
#56974=CARTESIAN_POINT ( 'NONE',  ( -19.50000000000000000, -3.499999999999999556, 29.75000000000000355 ) ) ;
#56977=VERTEX_POINT ( 'NONE', #78516 ) ;
#57015=EDGE_LOOP ( 'NONE', ( #29860, #15498, #39106, #43327 ) ) ;
#57027=VECTOR ( 'NONE', #80277, 1000.000000000000000 ) ;
#57028=ORIENTED_EDGE ( 'NONE', *, *, #45385, .T. ) ;
#57029=ADVANCED_FACE ( 'NONE', ( #87986 ), #73997, .T. ) ;
#57031=ORIENTED_EDGE ( 'NONE', *, *, #12931, .T. ) ;
#57042=ORIENTED_EDGE ( 'NONE', *, *, #16601, .F. ) ;
#57047=CARTESIAN_POINT ( 'NONE',  ( 0.000000000000000000, -11.00000000000000000, 29.75000000000000355 ) ) ;
#57052=EDGE_CURVE ( 'NONE', #14174, #73862, #60910, .T. ) ;
#57053=CARTESIAN_POINT ( 'NONE',  ( 17.06410256410256565, -3.499999999999999556, 29.75000000000000355 ) ) ;
#57065=ORIENTED_EDGE ( 'NONE', *, *, #64014, .T. ) ;
#57070=DIRECTION ( 'NONE',  ( 0.000000000000000000, 0.000000000000000000, 1.000000000000000000 ) ) ;
#57079=VECTOR ( 'NONE', #65187, 1000.000000000000000 ) ;
#57083=CARTESIAN_POINT ( 'NONE',  ( 14.16025641025641235, -7.500000000000000000, 29.75000000000000355 ) ) ;
#57089=CARTESIAN_POINT ( 'NONE',  ( -4.230769230769230838, -7.500000000000000000, 33.75000000000000000 ) ) ;
#57091=CARTESIAN_POINT ( 'NONE',  ( -19.50000000000000000, -3.499999999999999556, 29.75000000000000355 ) ) ;
#57101=AXIS2_PLACEMENT_3D ( 'NONE', #16362, #78061, #58225 ) ;
#57114=CARTESIAN_POINT ( 'NONE',  ( 6.416666666666664298, -7.500000000000000000, 29.75000000000000355 ) ) ;
#57143=AXIS2_PLACEMENT_3D ( 'NONE', #21000, #43057, #55674 ) ;
#57152=ORIENTED_EDGE ( 'NONE', *, *, #38614, .T. ) ;
#57155=ORIENTED_EDGE ( 'NONE', *, *, #20804, .T. ) ;
#57162=DIRECTION ( 'NONE',  ( 0.000000000000000000, 0.000000000000000000, -1.000000000000000000 ) ) ;
#57175=AXIS2_PLACEMENT_3D ( 'NONE', #72174, #78486, #51889 ) ;
#57177=ORIENTED_EDGE ( 'NONE', *, *, #6944, .F. ) ;
#57194=VERTEX_POINT ( 'NONE', #39762 ) ;
#57206=DIRECTION ( 'NONE',  ( -1.000000000000000000, -0.000000000000000000, -0.000000000000000000 ) ) ;
#57207=VERTEX_POINT ( 'NONE', #68118 ) ;
#57215=LINE ( 'NONE', #50446, #39003 ) ;
#57245=AXIS2_PLACEMENT_3D ( 'NONE', #6764, #40572, #11759 ) ;
#57250=ORIENTED_EDGE ( 'NONE', *, *, #24038, .T. ) ;
#57252=DIRECTION ( 'NONE',  ( -1.000000000000000000, 0.000000000000000000, -0.000000000000000000 ) ) ;
#57269=VECTOR ( 'NONE', #79953, 1000.000000000000000 ) ;
#57272=LINE ( 'NONE', #23040, #51120 ) ;
#57280=PRODUCT_DEFINITION_CONTEXT ( 'detailed design', #42340, 'design' ) ;
#57282=ORIENTED_EDGE ( 'NONE', *, *, #4853, .F. ) ;
#57291=DIRECTION ( 'NONE',  ( -0.000000000000000000, 1.000000000000000000, -0.000000000000000000 ) ) ;
#57296=AXIS2_PLACEMENT_3D ( 'NONE', #21284, #17647, #9986 ) ;
#57301=DIRECTION ( 'NONE',  ( -0.000000000000000000, 1.000000000000000000, -0.000000000000000000 ) ) ;
#57303=EDGE_LOOP ( 'NONE', ( #54843, #18816, #13947, #44173, #14397 ) ) ;
#57320=LINE ( 'NONE', #22644, #25941 ) ;
#57324=ORIENTED_EDGE ( 'NONE', *, *, #23452, .F. ) ;
#57333=CARTESIAN_POINT ( 'NONE',  ( 12.94230769230769340, -7.500000000000000000, 33.75000000000000000 ) ) ;
#57341=CARTESIAN_POINT ( 'NONE',  ( -7.134615384615385025, -3.499999999999999556, 29.75000000000000355 ) ) ;
#57343=CARTESIAN_POINT ( 'NONE',  ( 12.22435897435897267, -3.499999999999999556, 29.75000000000000355 ) ) ;
#57381=PLANE ( 'NONE',  #80493 ) ;
#57382=ORIENTED_EDGE ( 'NONE', *, *, #49700, .T. ) ;
#57384=CARTESIAN_POINT ( 'NONE',  ( 13.91025641025641235, -7.500000000000000000, 33.75000000000000000 ) ) ;
#57392=ORIENTED_EDGE ( 'NONE', *, *, #29078, .F. ) ;
#57420=ORIENTED_EDGE ( 'NONE', *, *, #83250, .F. ) ;
#57446=DIRECTION ( 'NONE',  ( -1.000000000000000000, 0.000000000000000000, -0.000000000000000000 ) ) ;
#57462=EDGE_LOOP ( 'NONE', ( #55403, #59417, #45980, #88287, #59254 ) ) ;
#57464=LINE ( 'NONE', #76866, #61880 ) ;
#57504=VECTOR ( 'NONE', #69573, 1000.000000000000000 ) ;
#57507=EDGE_LOOP ( 'NONE', ( #9404, #30933, #1206, #71791 ) ) ;
#57514=AXIS2_PLACEMENT_3D ( 'NONE', #22381, #1669, #56613 ) ;
#57541=CARTESIAN_POINT ( 'NONE',  ( 2.544871794871792936, -3.499999999999999556, 29.75000000000000355 ) ) ;
#57543=EDGE_CURVE ( 'NONE', #63049, #68522, #24794, .T. ) ;
#57547=AXIS2_PLACEMENT_3D ( 'NONE', #73046, #17665, #45119 ) ;
#57564=ORIENTED_EDGE ( 'NONE', *, *, #76189, .T. ) ;
#57574=AXIS2_PLACEMENT_3D ( 'NONE', #29534, #51101, #58320 ) ;
#57580=VECTOR ( 'NONE', #12809, 1000.000000000000000 ) ;
#57581=DIRECTION ( 'NONE',  ( 0.000000000000000000, 0.000000000000000000, 1.000000000000000000 ) ) ;
#57583=ORIENTED_EDGE ( 'NONE', *, *, #4735, .F. ) ;
#57596=LINE ( 'NONE', #3089, #66118 ) ;
#57607=DIRECTION ( 'NONE',  ( -0.000000000000000000, 0.000000000000000000, 1.000000000000000000 ) ) ;
#57615=VERTEX_POINT ( 'NONE', #48165 ) ;
#57619=ORIENTED_EDGE ( 'NONE', *, *, #54658, .F. ) ;
#57645=VECTOR ( 'NONE', #42031, 1000.000000000000000 ) ;
#57652=CARTESIAN_POINT ( 'NONE',  ( -14.87820512820512953, -7.500000000000000000, 29.75000000000000355 ) ) ;
#57675=CARTESIAN_POINT ( 'NONE',  ( 20.00000000000000000, -4.000000000000000000, 29.75000000000000355 ) ) ;
#57687=VERTEX_POINT ( 'NONE', #26132 ) ;
#57694=CARTESIAN_POINT ( 'NONE',  ( -11.00641025641025550, -7.500000000000000000, 29.75000000000000355 ) ) ;
#57700=ORIENTED_EDGE ( 'NONE', *, *, #29929, .T. ) ;
#57703=AXIS2_PLACEMENT_3D ( 'NONE', #6349, #68043, #54963 ) ;
#57708=VECTOR ( 'NONE', #14964, 1000.000000000000000 ) ;
#57719=DIRECTION ( 'NONE',  ( -0.000000000000000000, 1.000000000000000000, -0.000000000000000000 ) ) ;
#57729=LINE ( 'NONE', #71231, #64917 ) ;
#57736=EDGE_CURVE ( 'NONE', #48416, #47272, #35100, .T. ) ;
#57738=CYLINDRICAL_SURFACE ( 'NONE', #57296, 4.000000000000000000 ) ;
#57742=VECTOR ( 'NONE', #4036, 1000.000000000000000 ) ;
#57744=EDGE_CURVE ( 'NONE', #43102, #6970, #49507, .T. ) ;
#57747=DIRECTION ( 'NONE',  ( -1.000000000000000000, -0.000000000000000000, 0.000000000000000000 ) ) ;
#57750=CARTESIAN_POINT ( 'NONE',  ( 0.000000000000000000, -11.00000000000000000, 29.75000000000000355 ) ) ;
#57752=DIRECTION ( 'NONE',  ( -0.000000000000000000, 1.000000000000000000, -0.000000000000000000 ) ) ;
#57754=ORIENTED_EDGE ( 'NONE', *, *, #47841, .F. ) ;
#57764=CARTESIAN_POINT ( 'NONE',  ( 14.16025641025641235, -3.499999999999999556, 29.75000000000000355 ) ) ;
#57768=FACE_OUTER_BOUND ( 'NONE', #31699, .T. ) ;
#57770=AXIS2_PLACEMENT_3D ( 'NONE', #60608, #54739, #47537 ) ;
#57776=VECTOR ( 'NONE', #18897, 1000.000000000000000 ) ;
#57791=LINE ( 'NONE', #29453, #41206 ) ;
#57798=VECTOR ( 'NONE', #52740, 1000.000000000000000 ) ;
#57803=CIRCLE ( 'NONE', #23265, 4.000000000000000000 ) ;
#57814=EDGE_LOOP ( 'NONE', ( #28485, #34894, #30582, #76872 ) ) ;
#57815=ORIENTED_EDGE ( 'NONE', *, *, #22750, .F. ) ;
#57822=CIRCLE ( 'NONE', #26208, 4.000000000000000000 ) ;
#57835=DIRECTION ( 'NONE',  ( -1.000000000000000000, -0.000000000000000000, -0.000000000000000000 ) ) ;
#57844=CARTESIAN_POINT ( 'NONE',  ( 0.6089743589743582541, -7.500000000000000000, 29.75000000000000355 ) ) ;
#57855=VECTOR ( 'NONE', #12771, 1000.000000000000000 ) ;
#57858=PLANE ( 'NONE',  #48455 ) ;
#57899=ADVANCED_FACE ( 'NONE', ( #3956 ), #31443, .T. ) ;
#57903=DIRECTION ( 'NONE',  ( -0.000000000000000000, 1.000000000000000000, -0.000000000000000000 ) ) ;
#57906=DIRECTION ( 'NONE',  ( -0.000000000000000000, 1.000000000000000000, -0.000000000000000000 ) ) ;
#57934=FACE_OUTER_BOUND ( 'NONE', #39672, .T. ) ;
#57936=EDGE_CURVE ( 'NONE', #34055, #23619, #50805, .T. ) ;
#57956=VECTOR ( 'NONE', #57906, 1000.000000000000000 ) ;
#58001=VERTEX_POINT ( 'NONE', #10733 ) ;
#58007=DIRECTION ( 'NONE',  ( -1.000000000000000000, -0.000000000000000000, 0.000000000000000000 ) ) ;
#58009=DIRECTION ( 'NONE',  ( -1.000000000000000000, -0.000000000000000000, -0.000000000000000000 ) ) ;
#58019=DIRECTION ( 'NONE',  ( -1.000000000000000000, 0.000000000000000000, -0.000000000000000000 ) ) ;
#58025=EDGE_CURVE ( 'NONE', #50717, #44728, #26472, .T. ) ;
#58036=DIRECTION ( 'NONE',  ( -0.000000000000000000, 1.000000000000000000, -0.000000000000000000 ) ) ;
#58040=DIRECTION ( 'NONE',  ( 0.000000000000000000, 0.000000000000000000, 1.000000000000000000 ) ) ;
#58041=CARTESIAN_POINT ( 'NONE',  ( 0.000000000000000000, -11.00000000000000000, 29.75000000000000355 ) ) ;
#58069=PLANE ( 'NONE',  #13278 ) ;
#58072=ORIENTED_EDGE ( 'NONE', *, *, #71147, .F. ) ;
#58105=DIRECTION ( 'NONE',  ( 0.000000000000000000, 0.000000000000000000, -1.000000000000000000 ) ) ;
#58106=ORIENTED_EDGE ( 'NONE', *, *, #67215, .F. ) ;
#58108=CARTESIAN_POINT ( 'NONE',  ( -5.198717948717948012, -11.00000000000000000, 29.75000000000000355 ) ) ;
#58127=CARTESIAN_POINT ( 'NONE',  ( 19.00000000000000000, -7.500000000000000000, 33.75000000000000000 ) ) ;
#58131=ORIENTED_EDGE ( 'NONE', *, *, #80306, .F. ) ;
#58136=AXIS2_PLACEMENT_3D ( 'NONE', #17672, #60424, #18560 ) ;
#58140=VERTEX_POINT ( 'NONE', #7526 ) ;
#58141=ORIENTED_EDGE ( 'NONE', *, *, #66192, .F. ) ;
#58143=ORIENTED_EDGE ( 'NONE', *, *, #49509, .F. ) ;
#58148=VERTEX_POINT ( 'NONE', #28227 ) ;
#58158=VERTEX_POINT ( 'NONE', #70103 ) ;
#58161=CARTESIAN_POINT ( 'NONE',  ( -19.50000000000000000, -11.50000000000000000, 29.75000000000000355 ) ) ;
#58164=DIRECTION ( 'NONE',  ( -1.000000000000000000, -0.000000000000000000, -0.000000000000000000 ) ) ;
#58191=DIRECTION ( 'NONE',  ( 1.000000000000000000, 0.000000000000000000, 0.000000000000000000 ) ) ;
#58196=DIRECTION ( 'NONE',  ( 0.000000000000000000, 0.000000000000000000, -1.000000000000000000 ) ) ;
#58204=AXIS2_PLACEMENT_3D ( 'NONE', #60826, #12204, #32465 ) ;
#58213=PLANE ( 'NONE',  #57175 ) ;
#58225=DIRECTION ( 'NONE',  ( 0.000000000000000000, 0.000000000000000000, -1.000000000000000000 ) ) ;
#58226=ORIENTED_EDGE ( 'NONE', *, *, #79560, .F. ) ;
#58228=DIRECTION ( 'NONE',  ( -1.000000000000000000, 0.000000000000000000, -0.000000000000000000 ) ) ;
#58234=DIRECTION ( 'NONE',  ( -0.000000000000000000, 1.000000000000000000, -0.000000000000000000 ) ) ;
#58243=ADVANCED_FACE ( 'NONE', ( #9303 ), #25807, .T. ) ;
#58259=DIRECTION ( 'NONE',  ( 0.000000000000000000, 0.000000000000000000, -1.000000000000000000 ) ) ;
#58268=ORIENTED_EDGE ( 'NONE', *, *, #4458, .T. ) ;
#58286=ORIENTED_EDGE ( 'NONE', *, *, #78682, .F. ) ;
#58310=LINE ( 'NONE', #85357, #79472 ) ;
#58314=ORIENTED_EDGE ( 'NONE', *, *, #77565, .T. ) ;
#58320=DIRECTION ( 'NONE',  ( 0.000000000000000000, 0.000000000000000000, -1.000000000000000000 ) ) ;
#58322=DIRECTION ( 'NONE',  ( -0.000000000000000000, 1.000000000000000000, -0.000000000000000000 ) ) ;
#58324=CARTESIAN_POINT ( 'NONE',  ( 0.000000000000000000, -11.00000000000000000, 29.75000000000000355 ) ) ;
#58331=FACE_OUTER_BOUND ( 'NONE', #80259, .T. ) ;
#58359=EDGE_LOOP ( 'NONE', ( #77066, #22438, #33498, #9059, #10303 ) ) ;
#58367=AXIS2_PLACEMENT_3D ( 'NONE', #6384, #75277, #74386 ) ;
#58376=FACE_OUTER_BOUND ( 'NONE', #37820, .T. ) ;
#58381=ORIENTED_EDGE ( 'NONE', *, *, #30456, .F. ) ;
#58383=AXIS2_PLACEMENT_3D ( 'NONE', #61780, #48718, #55477 ) ;
#58389=FACE_OUTER_BOUND ( 'NONE', #34531, .T. ) ;
#58397=CARTESIAN_POINT ( 'NONE',  ( 15.84615384615384670, -7.500000000000000000, 29.75000000000000355 ) ) ;
#58403=VECTOR ( 'NONE', #41062, 1000.000000000000000 ) ;
#58407=ADVANCED_FACE ( 'NONE', ( #993 ), #12734, .T. ) ;
#58409=PLANE ( 'NONE',  #35436 ) ;
#58420=EDGE_CURVE ( 'NONE', #3529, #38748, #48727, .T. ) ;
#58428=ORIENTED_EDGE ( 'NONE', *, *, #18270, .T. ) ;
#58435=DIRECTION ( 'NONE',  ( 0.000000000000000000, 0.000000000000000000, 1.000000000000000000 ) ) ;
#58451=AXIS2_PLACEMENT_3D ( 'NONE', #76176, #46924, #27104 ) ;
#58464=AXIS2_PLACEMENT_3D ( 'NONE', #71741, #11837, #58228 ) ;
#58473=CARTESIAN_POINT ( 'NONE',  ( 20.00000000000000000, -11.50000000000000000, 28.25000000000000000 ) ) ;
#58480=PLANE ( 'NONE',  #83502 ) ;
#58483=DIRECTION ( 'NONE',  ( 0.000000000000000000, 0.000000000000000000, 1.000000000000000000 ) ) ;
#58488=ORIENTED_EDGE ( 'NONE', *, *, #55000, .F. ) ;
#58496=CIRCLE ( 'NONE', #54207, 4.000000000000000000 ) ;
#58501=DIRECTION ( 'NONE',  ( 0.000000000000000000, 0.000000000000000000, -1.000000000000000000 ) ) ;
#58502=CIRCLE ( 'NONE', #83170, 4.000000000000000000 ) ;
#58522=DIRECTION ( 'NONE',  ( -1.000000000000000000, -0.000000000000000000, -0.000000000000000000 ) ) ;
#58524=CARTESIAN_POINT ( 'NONE',  ( -7.134615384615385025, -11.50000000000000000, 29.75000000000000355 ) ) ;
#58538=VECTOR ( 'NONE', #16916, 1000.000000000000000 ) ;
#58564=LINE ( 'NONE', #86057, #82185 ) ;
#58584=ORIENTED_EDGE ( 'NONE', *, *, #54773, .T. ) ;
#58585=CARTESIAN_POINT ( 'NONE',  ( -9.070512820512819374, -7.500000000000000000, 33.75000000000000000 ) ) ;
#58593=FACE_OUTER_BOUND ( 'NONE', #46033, .T. ) ;
#58600=ORIENTED_EDGE ( 'NONE', *, *, #46962, .T. ) ;
#58601=CARTESIAN_POINT ( 'NONE',  ( 20.00000000000000000, -4.000000000000000000, 29.75000000000000355 ) ) ;
#58603=VERTEX_POINT ( 'NONE', #24803 ) ;
#58615=PLANE ( 'NONE',  #17115 ) ;
#58637=DIRECTION ( 'NONE',  ( -1.000000000000000000, -0.000000000000000000, 0.000000000000000000 ) ) ;
#58641=CARTESIAN_POINT ( 'NONE',  ( -17.78205128205128105, -7.500000000000000000, 29.75000000000000355 ) ) ;
#58676=DIRECTION ( 'NONE',  ( 1.000000000000000000, 0.000000000000000000, 0.000000000000000000 ) ) ;
#58677=CARTESIAN_POINT ( 'NONE',  ( -19.50000000000000000, -3.499999999999999556, 29.75000000000000355 ) ) ;
#58678=CIRCLE ( 'NONE', #42876, 4.000000000000000000 ) ;
#58692=FACE_OUTER_BOUND ( 'NONE', #36874, .T. ) ;
#58709=DIRECTION ( 'NONE',  ( -0.000000000000000000, 1.000000000000000000, -0.000000000000000000 ) ) ;
#58713=CARTESIAN_POINT ( 'NONE',  ( 1.576923076923075762, -3.499999999999999556, 29.75000000000000355 ) ) ;
#58726=VERTEX_POINT ( 'NONE', #54044 ) ;
#58729=VECTOR ( 'NONE', #8352, 1000.000000000000000 ) ;
#58733=DIRECTION ( 'NONE',  ( 1.000000000000000000, 0.000000000000000000, 0.000000000000000000 ) ) ;
#58735=ORIENTED_EDGE ( 'NONE', *, *, #84991, .T. ) ;
#58742=PLANE ( 'NONE',  #63209 ) ;
#58747=CARTESIAN_POINT ( 'NONE',  ( 15.84615384615384670, -3.499999999999999556, 29.75000000000000355 ) ) ;
#58754=FACE_OUTER_BOUND ( 'NONE', #52393, .T. ) ;
#58755=AXIS2_PLACEMENT_3D ( 'NONE', #11321, #52300, #45547 ) ;
#58779=VECTOR ( 'NONE', #64811, 1000.000000000000000 ) ;
#58784=LINE ( 'NONE', #52023, #42628 ) ;
#58786=DIRECTION ( 'NONE',  ( -1.000000000000000000, -0.000000000000000000, -0.000000000000000000 ) ) ;
#58787=LINE ( 'NONE', #86290, #31337 ) ;
#58789=ORIENTED_EDGE ( 'NONE', *, *, #2716, .F. ) ;
#58804=ORIENTED_EDGE ( 'NONE', *, *, #87197, .F. ) ;
#58806=FACE_OUTER_BOUND ( 'NONE', #18743, .T. ) ;
#58809=LINE ( 'NONE', #72766, #35575 ) ;
#58814=EDGE_LOOP ( 'NONE', ( #22115, #48757, #61832, #12089 ) ) ;
#58816=VERTEX_POINT ( 'NONE', #69351 ) ;
#58820=FACE_OUTER_BOUND ( 'NONE', #71743, .T. ) ;
#58828=PLANE ( 'NONE',  #88797 ) ;
#58832=CARTESIAN_POINT ( 'NONE',  ( 19.50000000000000000, -7.500000000000000000, 29.75000000000000355 ) ) ;
#58862=AXIS2_PLACEMENT_3D ( 'NONE', #9086, #28464, #77534 ) ;
#58874=FACE_OUTER_BOUND ( 'NONE', #53517, .T. ) ;
#58886=ORIENTED_EDGE ( 'NONE', *, *, #73551, .T. ) ;
#58888=AXIS2_PLACEMENT_3D ( 'NONE', #57114, #84607, #15696 ) ;
#58897=CARTESIAN_POINT ( 'NONE',  ( 18.03205128205128105, -7.500000000000000000, 33.75000000000000000 ) ) ;
#58899=LINE ( 'NONE', #71523, #13973 ) ;
#58906=DIRECTION ( 'NONE',  ( -1.000000000000000000, -0.000000000000000000, -0.000000000000000000 ) ) ;
#58920=VECTOR ( 'NONE', #39504, 1000.000000000000000 ) ;
#58926=DIRECTION ( 'NONE',  ( 1.000000000000000000, 0.000000000000000000, 0.000000000000000000 ) ) ;
#58939=CARTESIAN_POINT ( 'NONE',  ( 11.00641025641025550, -3.499999999999999556, 29.75000000000000355 ) ) ;
#58964=VERTEX_POINT ( 'NONE', #17500 ) ;
#58973=CARTESIAN_POINT ( 'NONE',  ( 2.544871794871793824, -11.50000000000000000, 29.75000000000000355 ) ) ;
#58982=AXIS2_PLACEMENT_3D ( 'NONE', #84223, #49083, #83328 ) ;
#59011=PLANE ( 'NONE',  #49951 ) ;
#59013=PLANE ( 'NONE',  #83129 ) ;
#59047=CARTESIAN_POINT ( 'NONE',  ( -19.50000000000000000, -3.499999999999999556, 29.75000000000000355 ) ) ;
#59051=ORIENTED_EDGE ( 'NONE', *, *, #57543, .T. ) ;
#59060=VERTEX_POINT ( 'NONE', #13841 ) ;
#59062=PLANE ( 'NONE',  #35710 ) ;
#59065=EDGE_CURVE ( 'NONE', #87793, #63742, #47635, .T. ) ;
#59074=ADVANCED_FACE ( 'NONE', ( #81431 ), #33680, .F. ) ;
#59081=ORIENTED_EDGE ( 'NONE', *, *, #9513, .T. ) ;
#59097=ORIENTED_EDGE ( 'NONE', *, *, #14110, .F. ) ;
#59099=DIRECTION ( 'NONE',  ( 0.000000000000000000, 0.000000000000000000, -1.000000000000000000 ) ) ;
#59110=VECTOR ( 'NONE', #69046, 1000.000000000000000 ) ;
#59122=DIRECTION ( 'NONE',  ( 1.000000000000000000, 0.000000000000000000, 0.000000000000000000 ) ) ;
#59129=VERTEX_POINT ( 'NONE', #48061 ) ;
#59137=DIRECTION ( 'NONE',  ( -1.000000000000000000, -0.000000000000000000, -0.000000000000000000 ) ) ;
#59143=VECTOR ( 'NONE', #61327, 1000.000000000000000 ) ;
#59157=VERTEX_POINT ( 'NONE', #5764 ) ;
#59168=EDGE_CURVE ( 'NONE', #13394, #13635, #45027, .T. ) ;
#59169=VECTOR ( 'NONE', #74495, 1000.000000000000000 ) ;
#59173=EDGE_CURVE ( 'NONE', #24890, #26148, #63740, .T. ) ;
#59178=CARTESIAN_POINT ( 'NONE',  ( 18.03205128205128105, -7.500000000000000000, 29.75000000000000355 ) ) ;
#59189=EDGE_LOOP ( 'NONE', ( #71128, #57282, #28582, #85924, #6226 ) ) ;
#59193=CARTESIAN_POINT ( 'NONE',  ( 9.070512820512819374, -7.500000000000000000, 29.75000000000000355 ) ) ;
#59206=ADVANCED_FACE ( 'NONE', ( #21034 ), #77316, .T. ) ;
#59214=LINE ( 'NONE', #88494, #73467 ) ;
#59228=ORIENTED_EDGE ( 'NONE', *, *, #7715, .T. ) ;
#59232=CARTESIAN_POINT ( 'NONE',  ( -4.480769230769230838, -3.499999999999999556, 29.75000000000000355 ) ) ;
#59238=ORIENTED_EDGE ( 'NONE', *, *, #77003, .F. ) ;
#59242=CIRCLE ( 'NONE', #70762, 4.000000000000000000 ) ;
#59245=DIRECTION ( 'NONE',  ( 0.000000000000000000, 0.000000000000000000, -1.000000000000000000 ) ) ;
#59248=CARTESIAN_POINT ( 'NONE',  ( -12.22435897435897267, -11.00000000000000000, 29.75000000000000355 ) ) ;
#59254=ORIENTED_EDGE ( 'NONE', *, *, #49265, .T. ) ;
#59256=DIRECTION ( 'NONE',  ( -0.000000000000000000, 0.000000000000000000, 1.000000000000000000 ) ) ;
#59267=ORIENTED_EDGE ( 'NONE', *, *, #36001, .F. ) ;
#59276=ADVANCED_FACE ( 'NONE', ( #84968 ), #78643, .T. ) ;
#59285=DIRECTION ( 'NONE',  ( 1.000000000000000000, 0.000000000000000000, 0.000000000000000000 ) ) ;
#59308=LINE ( 'NONE', #86814, #26236 ) ;
#59310=DIRECTION ( 'NONE',  ( 0.000000000000000000, 0.000000000000000000, -1.000000000000000000 ) ) ;
#59315=CIRCLE ( 'NONE', #17607, 4.000000000000000000 ) ;
#59324=ORIENTED_EDGE ( 'NONE', *, *, #44827, .F. ) ;
#59326=PLANE ( 'NONE',  #34510 ) ;
#59330=PLANE ( 'NONE',  #74302 ) ;
#59339=CARTESIAN_POINT ( 'NONE',  ( 2.544871794871792936, -3.499999999999999556, 29.75000000000000355 ) ) ;
#59342=CARTESIAN_POINT ( 'NONE',  ( 3.262820512820510999, -7.500000000000000000, 29.75000000000000355 ) ) ;
#59364=EDGE_CURVE ( 'NONE', #11346, #7995, #25482, .T. ) ;
#59365=DIRECTION ( 'NONE',  ( 1.000000000000000000, 0.000000000000000000, 0.000000000000000000 ) ) ;
#59374=EDGE_LOOP ( 'NONE', ( #64586, #69546, #49045, #46558 ) ) ;
#59379=CYLINDRICAL_SURFACE ( 'NONE', #76961, 4.000000000000000000 ) ;
#59392=DIRECTION ( 'NONE',  ( -1.000000000000000000, -0.000000000000000000, -0.000000000000000000 ) ) ;
#59393=ORIENTED_EDGE ( 'NONE', *, *, #21667, .F. ) ;
#59402=VECTOR ( 'NONE', #74848, 1000.000000000000000 ) ;
#59405=CARTESIAN_POINT ( 'NONE',  ( 12.22435897435897267, -3.499999999999999556, 29.75000000000000355 ) ) ;
#59417=ORIENTED_EDGE ( 'NONE', *, *, #64405, .T. ) ;
#59425=LINE ( 'NONE', #60310, #64737 ) ;
#59448=EDGE_CURVE ( 'NONE', #1012, #36253, #75009, .T. ) ;
#59451=EDGE_CURVE ( 'NONE', #1878, #19254, #88980, .T. ) ;
#59468=CARTESIAN_POINT ( 'NONE',  ( -19.50000000000000000, -11.50000000000000000, 29.75000000000000355 ) ) ;
#59471=AXIS2_PLACEMENT_3D ( 'NONE', #85292, #29031, #30774 ) ;
#59474=EDGE_LOOP ( 'NONE', ( #15531, #84394, #68884, #83923, #87902 ) ) ;
#59492=CARTESIAN_POINT ( 'NONE',  ( -6.166666666666667851, -7.500000000000000000, 29.75000000000000355 ) ) ;
#59497=PLANE ( 'NONE',  #78255 ) ;
#59499=ORIENTED_EDGE ( 'NONE', *, *, #13382, .T. ) ;
#59507=DIRECTION ( 'NONE',  ( 0.000000000000000000, 1.000000000000000000, -0.000000000000000000 ) ) ;
#59518=ORIENTED_EDGE ( 'NONE', *, *, #69647, .F. ) ;
#59549=DIRECTION ( 'NONE',  ( -1.000000000000000000, -0.000000000000000000, 0.000000000000000000 ) ) ;
#59552=CARTESIAN_POINT ( 'NONE',  ( 10.28846153846153832, -11.50000000000000000, 29.75000000000000355 ) ) ;
#59553=ORIENTED_EDGE ( 'NONE', *, *, #5423, .F. ) ;
#59557=CARTESIAN_POINT ( 'NONE',  ( -9.070512820512819374, -11.50000000000000000, 29.75000000000000355 ) ) ;
#59565=FACE_OUTER_BOUND ( 'NONE', #50818, .T. ) ;
#59576=ADVANCED_FACE ( 'NONE', ( #7873 ), #28134, .T. ) ;
#59590=VERTEX_POINT ( 'NONE', #29920 ) ;
#59601=CARTESIAN_POINT ( 'NONE',  ( 18.03205128205128105, -7.500000000000000000, 29.75000000000000355 ) ) ;
#59625=CARTESIAN_POINT ( 'NONE',  ( -19.50000000000000000, -3.499999999999999556, 29.75000000000000355 ) ) ;
#59644=DIRECTION ( 'NONE',  ( -1.000000000000000000, -0.000000000000000000, -0.000000000000000000 ) ) ;
#59652=ORIENTED_EDGE ( 'NONE', *, *, #18699, .F. ) ;
#59655=LINE ( 'NONE', #67311, #25417 ) ;
#59663=LINE ( 'NONE', #72727, #83308 ) ;
#59670=DIRECTION ( 'NONE',  ( -0.000000000000000000, 0.000000000000000000, 1.000000000000000000 ) ) ;
#59686=ORIENTED_EDGE ( 'NONE', *, *, #50256, .T. ) ;
#59702=DIRECTION ( 'NONE',  ( 1.000000000000000000, 0.000000000000000000, 0.000000000000000000 ) ) ;
#59719=EDGE_CURVE ( 'NONE', #427, #82221, #63793, .T. ) ;
#59724=EDGE_CURVE ( 'NONE', #48246, #13160, #12746, .T. ) ;
#59728=CARTESIAN_POINT ( 'NONE',  ( 1.326923076923075762, -7.500000000000000000, 29.75000000000000355 ) ) ;
#59729=CARTESIAN_POINT ( 'NONE',  ( 9.320512820512821150, -3.499999999999999556, 29.75000000000000355 ) ) ;
#59730=ADVANCED_FACE ( 'NONE', ( #67696 ), #88002, .F. ) ;
#59745=CARTESIAN_POINT ( 'NONE',  ( 20.00000000000000000, -4.000000000000000000, 29.75000000000000355 ) ) ;
#59757=DIRECTION ( 'NONE',  ( 0.000000000000000000, 0.000000000000000000, -1.000000000000000000 ) ) ;
#59779=DIRECTION ( 'NONE',  ( 0.000000000000000000, 0.000000000000000000, -1.000000000000000000 ) ) ;
#59786=VECTOR ( 'NONE', #31762, 1000.000000000000000 ) ;
#59814=AXIS2_PLACEMENT_3D ( 'NONE', #67815, #47528, #47972 ) ;
#59819=LINE ( 'NONE', #67031, #67499 ) ;
#59822=LINE ( 'NONE', #39124, #52503 ) ;
#59825=CARTESIAN_POINT ( 'NONE',  ( -1.326923076923076206, -11.50000000000000000, 29.75000000000000355 ) ) ;
#59833=EDGE_CURVE ( 'NONE', #32893, #87104, #56720, .T. ) ;
#59842=VECTOR ( 'NONE', #43832, 1000.000000000000000 ) ;
#59850=EDGE_CURVE ( 'NONE', #28389, #20358, #22931, .T. ) ;
#59851=CARTESIAN_POINT ( 'NONE',  ( 4.480769230769229061, -7.500000000000000000, 33.75000000000000000 ) ) ;
#59873=ADVANCED_FACE ( 'NONE', ( #77873 ), #9422, .F. ) ;
#59881=EDGE_CURVE ( 'NONE', #87104, #47433, #78310, .T. ) ;
#59895=ORIENTED_EDGE ( 'NONE', *, *, #81264, .T. ) ;
#59901=ORIENTED_EDGE ( 'NONE', *, *, #46089, .F. ) ;
#59909=DIRECTION ( 'NONE',  ( -0.000000000000000000, 1.000000000000000000, -0.000000000000000000 ) ) ;
#59915=ORIENTED_EDGE ( 'NONE', *, *, #6420, .F. ) ;
#59917=ORIENTED_EDGE ( 'NONE', *, *, #18918, .T. ) ;
#59941=EDGE_CURVE ( 'NONE', #48029, #61382, #10308, .T. ) ;
#59985=DIRECTION ( 'NONE',  ( 1.000000000000000000, 0.000000000000000000, 0.000000000000000000 ) ) ;
#59989=CARTESIAN_POINT ( 'NONE',  ( 17.06410256410256565, -7.500000000000000000, 29.75000000000000355 ) ) ;
#59998=LINE ( 'NONE', #12704, #3939 ) ;
#60009=LINE ( 'NONE', #73542, #74520 ) ;
#60013=VECTOR ( 'NONE', #67652, 1000.000000000000000 ) ;
#60018=DIRECTION ( 'NONE',  ( 1.000000000000000000, 0.000000000000000000, 0.000000000000000000 ) ) ;
#60026=CARTESIAN_POINT ( 'NONE',  ( 4.230769230769229061, -3.499999999999999556, 29.75000000000000355 ) ) ;
#60029=CARTESIAN_POINT ( 'NONE',  ( 0.000000000000000000, -11.00000000000000000, 29.75000000000000355 ) ) ;
#60033=VERTEX_POINT ( 'NONE', #18847 ) ;
#60034=AXIS2_PLACEMENT_3D ( 'NONE', #15256, #62972, #1733 ) ;
#60051=CARTESIAN_POINT ( 'NONE',  ( 0.000000000000000000, -4.000000000000000000, 28.75000000000000000 ) ) ;
#60055=ORIENTED_EDGE ( 'NONE', *, *, #44827, .T. ) ;
#60058=DIRECTION ( 'NONE',  ( -0.000000000000000000, 1.000000000000000000, -0.000000000000000000 ) ) ;
#60066=LINE ( 'NONE', #79008, #1587 ) ;
#60068=ORIENTED_EDGE ( 'NONE', *, *, #41100, .T. ) ;
#60074=FACE_OUTER_BOUND ( 'NONE', #45924, .T. ) ;
#60091=DIRECTION ( 'NONE',  ( 0.000000000000000000, 0.000000000000000000, -1.000000000000000000 ) ) ;
#60093=EDGE_CURVE ( 'NONE', #20476, #24943, #81448, .T. ) ;
#60110=DIRECTION ( 'NONE',  ( -0.000000000000000000, 1.000000000000000000, -0.000000000000000000 ) ) ;
#60111=LINE ( 'NONE', #88501, #82290 ) ;
#60120=PLANE ( 'NONE',  #13285 ) ;
#60122=AXIS2_PLACEMENT_3D ( 'NONE', #83117, #1584, #84895 ) ;
#60127=ORIENTED_EDGE ( 'NONE', *, *, #29678, .T. ) ;
#60164=ADVANCED_FACE ( 'NONE', ( #34128 ), #54845, .T. ) ;
#60170=ORIENTED_EDGE ( 'NONE', *, *, #3154, .F. ) ;
#60179=CARTESIAN_POINT ( 'NONE',  ( -5.448717948717948012, -7.500000000000000000, 29.75000000000000355 ) ) ;
#60184=LINE ( 'NONE', #4363, #10274 ) ;
#60230=EDGE_CURVE ( 'NONE', #86240, #22218, #56618, .T. ) ;
#60231=VECTOR ( 'NONE', #37234, 1000.000000000000000 ) ;
#60248=CARTESIAN_POINT ( 'NONE',  ( -8.102564102564102200, -3.499999999999999556, 29.75000000000000355 ) ) ;
#60250=AXIS2_PLACEMENT_3D ( 'NONE', #42461, #35706, #28959 ) ;
#60252=CARTESIAN_POINT ( 'NONE',  ( 0.000000000000000000, -11.00000000000000000, 29.75000000000000355 ) ) ;
#60259=CARTESIAN_POINT ( 'NONE',  ( -15.12820512820512953, -7.500000000000000000, 33.75000000000000000 ) ) ;
#60266=DIRECTION ( 'NONE',  ( -1.000000000000000000, -0.000000000000000000, -0.000000000000000000 ) ) ;
#60269=LINE ( 'NONE', #61152, #28440 ) ;
#60273=CIRCLE ( 'NONE', #68890, 4.000000000000000000 ) ;
#60288=EDGE_CURVE ( 'NONE', #76927, #20882, #28707, .T. ) ;
#60301=ORIENTED_EDGE ( 'NONE', *, *, #20827, .F. ) ;
#60305=CARTESIAN_POINT ( 'NONE',  ( -4.480769230769230838, -3.499999999999999556, 29.75000000000000355 ) ) ;
#60310=CARTESIAN_POINT ( 'NONE',  ( 0.000000000000000000, -11.00000000000000000, 29.75000000000000355 ) ) ;
#60320=ORIENTED_EDGE ( 'NONE', *, *, #19926, .T. ) ;
#60353=CARTESIAN_POINT ( 'NONE',  ( 20.00000000000000000, -4.000000000000000000, 29.75000000000000355 ) ) ;
#60356=EDGE_CURVE ( 'NONE', #2085, #34232, #82637, .T. ) ;
#60359=ORIENTED_EDGE ( 'NONE', *, *, #78616, .T. ) ;
#60373=CARTESIAN_POINT ( 'NONE',  ( 8.102564102564102200, -3.499999999999999556, 29.75000000000000355 ) ) ;
#60378=DIRECTION ( 'NONE',  ( 0.000000000000000000, 0.000000000000000000, -1.000000000000000000 ) ) ;
#60392=DIRECTION ( 'NONE',  ( -0.000000000000000000, 1.000000000000000000, -0.000000000000000000 ) ) ;
#60400=ORIENTED_EDGE ( 'NONE', *, *, #61975, .T. ) ;
#60405=ORIENTED_EDGE ( 'NONE', *, *, #64548, .T. ) ;
#60414=VECTOR ( 'NONE', #78654, 1000.000000000000000 ) ;
#60417=EDGE_CURVE ( 'NONE', #35014, #17254, #68658, .T. ) ;
#60420=ORIENTED_EDGE ( 'NONE', *, *, #26628, .T. ) ;
#60421=DIRECTION ( 'NONE',  ( -0.000000000000000000, 0.000000000000000000, 1.000000000000000000 ) ) ;
#60424=DIRECTION ( 'NONE',  ( -1.000000000000000000, -0.000000000000000000, -0.000000000000000000 ) ) ;
#60456=ADVANCED_FACE ( 'NONE', ( #36648 ), #44264, .F. ) ;
#60459=LINE ( 'NONE', #47384, #84004 ) ;
#60480=ORIENTED_EDGE ( 'NONE', *, *, #40650, .F. ) ;
#60499=DIRECTION ( 'NONE',  ( -0.000000000000000000, 1.000000000000000000, -0.000000000000000000 ) ) ;
#60506=ORIENTED_EDGE ( 'NONE', *, *, #70971, .T. ) ;
#60532=DIRECTION ( 'NONE',  ( -1.000000000000000000, -0.000000000000000000, -0.000000000000000000 ) ) ;
#60539=ORIENTED_EDGE ( 'NONE', *, *, #71147, .T. ) ;
#60540=CIRCLE ( 'NONE', #21699, 4.000000000000000000 ) ;
#60543=ORIENTED_EDGE ( 'NONE', *, *, #27334, .T. ) ;
#60549=CIRCLE ( 'NONE', #18824, 4.000000000000000000 ) ;
#60550=LINE ( 'NONE', #53792, #7253 ) ;
#60552=FACE_OUTER_BOUND ( 'NONE', #7054, .T. ) ;
#60562=CARTESIAN_POINT ( 'NONE',  ( -19.50000000000000000, -3.499999999999999556, 29.75000000000000355 ) ) ;
#60579=VERTEX_POINT ( 'NONE', #79411 ) ;
#60581=EDGE_CURVE ( 'NONE', #27068, #20882, #4183, .T. ) ;
#60587=DIRECTION ( 'NONE',  ( -0.000000000000000000, 1.000000000000000000, -0.000000000000000000 ) ) ;
#60589=AXIS2_PLACEMENT_3D ( 'NONE', #3988, #18412, #44082 ) ;
#60603=CARTESIAN_POINT ( 'NONE',  ( -12.94230769230769162, -3.499999999999999556, 29.75000000000000355 ) ) ;
#60607=DIRECTION ( 'NONE',  ( 1.000000000000000000, 0.000000000000000000, 0.000000000000000000 ) ) ;
#60608=CARTESIAN_POINT ( 'NONE',  ( 2.544871794871792936, -7.500000000000000000, 29.75000000000000355 ) ) ;
#60611=DIRECTION ( 'NONE',  ( 1.000000000000000000, 0.000000000000000000, 0.000000000000000000 ) ) ;
#60613=VERTEX_POINT ( 'NONE', #25795 ) ;
#60638=LINE ( 'NONE', #52547, #33758 ) ;
#60647=DIRECTION ( 'NONE',  ( -1.000000000000000000, -0.000000000000000000, 0.000000000000000000 ) ) ;
#60665=CARTESIAN_POINT ( 'NONE',  ( 19.50000000000000000, -11.00000000000000000, 28.25000000000000000 ) ) ;
#60667=DIRECTION ( 'NONE',  ( 0.000000000000000000, 0.000000000000000000, 1.000000000000000000 ) ) ;
#60670=VECTOR ( 'NONE', #37502, 1000.000000000000000 ) ;
#60686=CARTESIAN_POINT ( 'NONE',  ( 9.320512820512821150, -4.000000000000000000, 28.25000000000000000 ) ) ;
#60688=ORIENTED_EDGE ( 'NONE', *, *, #23816, .T. ) ;
#60700=DIRECTION ( 'NONE',  ( 1.000000000000000000, 0.000000000000000000, 0.000000000000000000 ) ) ;
#60711=ORIENTED_EDGE ( 'NONE', *, *, #6420, .T. ) ;
#60736=CARTESIAN_POINT ( 'NONE',  ( 3.512820512820510555, -7.500000000000000000, 33.75000000000000000 ) ) ;
#60750=FACE_OUTER_BOUND ( 'NONE', #13633, .T. ) ;
#60756=FACE_OUTER_BOUND ( 'NONE', #61735, .T. ) ;
#60762=DIRECTION ( 'NONE',  ( 1.000000000000000000, 0.000000000000000000, 0.000000000000000000 ) ) ;
#60788=ORIENTED_EDGE ( 'NONE', *, *, #32069, .T. ) ;
#60789=VECTOR ( 'NONE', #61745, 1000.000000000000000 ) ;
#60826=CARTESIAN_POINT ( 'NONE',  ( -4.230769230769230838, -7.500000000000000000, 29.75000000000000355 ) ) ;
#60876=DIRECTION ( 'NONE',  ( 1.000000000000000000, 0.000000000000000000, 0.000000000000000000 ) ) ;
#60895=DIRECTION ( 'NONE',  ( -1.000000000000000000, 0.000000000000000000, -0.000000000000000000 ) ) ;
#60898=VERTEX_POINT ( 'NONE', #28258 ) ;
#60906=ORIENTED_EDGE ( 'NONE', *, *, #17840, .F. ) ;
#60910=LINE ( 'NONE', #26686, #43430 ) ;
#60919=ADVANCED_FACE ( 'NONE', ( #357 ), #48980, .F. ) ;
#60922=DIRECTION ( 'NONE',  ( -1.000000000000000000, -0.000000000000000000, -0.000000000000000000 ) ) ;
#60983=AXIS2_PLACEMENT_3D ( 'NONE', #35466, #61602, #1231 ) ;
#60984=SHAPE_REPRESENTATION ( 'Dual Reciprocating Inner Cutter Blades', ( #83448 ), #70522 ) ;
#60991=EDGE_CURVE ( 'NONE', #55273, #75823, #33664, .T. ) ;
#60993=CARTESIAN_POINT ( 'NONE',  ( 0.000000000000000000, -11.00000000000000000, 29.75000000000000355 ) ) ;
#60996=DIRECTION ( 'NONE',  ( -1.000000000000000000, -0.000000000000000000, -0.000000000000000000 ) ) ;
#61005=ORIENTED_EDGE ( 'NONE', *, *, #52784, .T. ) ;
#61033=EDGE_CURVE ( 'NONE', #29561, #45384, #64245, .T. ) ;
#61034=DIRECTION ( 'NONE',  ( 1.000000000000000000, 0.000000000000000000, 0.000000000000000000 ) ) ;
#61055=EDGE_LOOP ( 'NONE', ( #17337, #69792, #22785, #37547 ) ) ;
#61072=ADVANCED_FACE ( 'NONE', ( #58376 ), #37225, .F. ) ;
#61079=DIRECTION ( 'NONE',  ( 0.000000000000000000, 0.000000000000000000, -1.000000000000000000 ) ) ;
#61086=ORIENTED_EDGE ( 'NONE', *, *, #2448, .F. ) ;
#61098=CIRCLE ( 'NONE', #74030, 4.000000000000000000 ) ;
#61100=LINE ( 'NONE', #48805, #21171 ) ;
#61108=PLANE ( 'NONE',  #44198 ) ;
#61109=LINE ( 'NONE', #54792, #84809 ) ;
#61111=ORIENTED_EDGE ( 'NONE', *, *, #40514, .T. ) ;
#61135=DIRECTION ( 'NONE',  ( -1.000000000000000000, 0.000000000000000000, -0.000000000000000000 ) ) ;
#61138=ORIENTED_EDGE ( 'NONE', *, *, #38778, .T. ) ;
#61141=CARTESIAN_POINT ( 'NONE',  ( -10.03846153846153832, -7.500000000000000000, 33.75000000000000000 ) ) ;
#61144=AXIS2_PLACEMENT_3D ( 'NONE', #21526, #22412, #55750 ) ;
#61152=CARTESIAN_POINT ( 'NONE',  ( 10.28846153846153832, -3.499999999999999556, 29.75000000000000355 ) ) ;
#61153=EDGE_CURVE ( 'NONE', #3259, #42959, #13599, .T. ) ;
#61156=FACE_OUTER_BOUND ( 'NONE', #87313, .T. ) ;
#61164=PLANE ( 'NONE',  #85191 ) ;
#61169=CARTESIAN_POINT ( 'NONE',  ( -5.448717948717948012, -3.499999999999999556, 29.75000000000000355 ) ) ;
#61175=EDGE_CURVE ( 'NONE', #34461, #46042, #26390, .T. ) ;
#61178=DIRECTION ( 'NONE',  ( 0.000000000000000000, 0.000000000000000000, -1.000000000000000000 ) ) ;
#61231=LINE ( 'NONE', #88739, #26529 ) ;
#61241=ORIENTED_EDGE ( 'NONE', *, *, #78640, .T. ) ;
#61244=AXIS2_PLACEMENT_3D ( 'NONE', #60562, #69101, #55574 ) ;
#61261=ORIENTED_EDGE ( 'NONE', *, *, #15711, .T. ) ;
#61273=PLANE ( 'NONE',  #86183 ) ;
#61275=CARTESIAN_POINT ( 'NONE',  ( 13.19230769230769340, -7.500000000000000000, 29.75000000000000355 ) ) ;
#61277=ORIENTED_EDGE ( 'NONE', *, *, #4526, .T. ) ;
#61289=ORIENTED_EDGE ( 'NONE', *, *, #3834, .F. ) ;
#61291=DIRECTION ( 'NONE',  ( 1.000000000000000000, 0.000000000000000000, 0.000000000000000000 ) ) ;
#61305=ADVANCED_FACE ( 'NONE', ( #24516 ), #38944, .T. ) ;
#61324=( NAMED_UNIT ( * ) SI_UNIT ( $, .STERADIAN. ) SOLID_ANGLE_UNIT ( ) );
#61327=DIRECTION ( 'NONE',  ( -0.000000000000000000, 1.000000000000000000, -0.000000000000000000 ) ) ;
#61345=CARTESIAN_POINT ( 'NONE',  ( -6.166666666666667851, -7.500000000000000000, 33.75000000000000000 ) ) ;
#61375=VECTOR ( 'NONE', #48553, 1000.000000000000000 ) ;
#61382=VERTEX_POINT ( 'NONE', #27633 ) ;
#61394=VERTEX_POINT ( 'NONE', #6914 ) ;
#61404=VECTOR ( 'NONE', #54573, 1000.000000000000000 ) ;
#61424=DIRECTION ( 'NONE',  ( 1.000000000000000000, 0.000000000000000000, 0.000000000000000000 ) ) ;
#61437=DIRECTION ( 'NONE',  ( 0.000000000000000000, 0.000000000000000000, -1.000000000000000000 ) ) ;
#61439=ORIENTED_EDGE ( 'NONE', *, *, #46965, .T. ) ;
#61453=EDGE_CURVE ( 'NONE', #51043, #86240, #54208, .T. ) ;
#61474=VECTOR ( 'NONE', #18346, 1000.000000000000000 ) ;
#61486=ORIENTED_EDGE ( 'NONE', *, *, #31527, .T. ) ;
#61489=CARTESIAN_POINT ( 'NONE',  ( -19.50000000000000000, -3.499999999999999556, 29.75000000000000355 ) ) ;
#61499=DIRECTION ( 'NONE',  ( -1.000000000000000000, -0.000000000000000000, 0.000000000000000000 ) ) ;
#61504=DIRECTION ( 'NONE',  ( 0.000000000000000000, 0.000000000000000000, -1.000000000000000000 ) ) ;
#61523=DIRECTION ( 'NONE',  ( 1.000000000000000000, 0.000000000000000000, 0.000000000000000000 ) ) ;
#61529=PLANE ( 'NONE',  #61889 ) ;
#61532=CARTESIAN_POINT ( 'NONE',  ( -14.87820512820512953, -3.499999999999999556, 29.75000000000000355 ) ) ;
#61548=ORIENTED_EDGE ( 'NONE', *, *, #82132, .F. ) ;
#61559=ORIENTED_EDGE ( 'NONE', *, *, #21341, .F. ) ;
#61561=ORIENTED_EDGE ( 'NONE', *, *, #72434, .T. ) ;
#61562=CIRCLE ( 'NONE', #80293, 4.000000000000000000 ) ;
#61563=CARTESIAN_POINT ( 'NONE',  ( -5.198717948717948012, -11.50000000000000000, 29.75000000000000355 ) ) ;
#61567=DIRECTION ( 'NONE',  ( -1.000000000000000000, 0.000000000000000000, -0.000000000000000000 ) ) ;
#61568=VECTOR ( 'NONE', #20828, 1000.000000000000000 ) ;
#61573=ADVANCED_FACE ( 'NONE', ( #86587 ), #46024, .T. ) ;
#61582=EDGE_LOOP ( 'NONE', ( #29689, #67750, #39341, #71274 ) ) ;
#61590=EDGE_CURVE ( 'NONE', #51043, #61382, #53219, .T. ) ;
#61594=CARTESIAN_POINT ( 'NONE',  ( -19.50000000000000000, -3.499999999999999556, 29.75000000000000355 ) ) ;
#61602=DIRECTION ( 'NONE',  ( 1.000000000000000000, 0.000000000000000000, 0.000000000000000000 ) ) ;
#61603=CYLINDRICAL_SURFACE ( 'NONE', #25934, 0.5000000000000004441 ) ;
#61617=DIRECTION ( 'NONE',  ( 1.000000000000000000, 0.000000000000000000, 0.000000000000000000 ) ) ;
#61622=DIRECTION ( 'NONE',  ( 1.000000000000000000, 0.000000000000000000, 0.000000000000000000 ) ) ;
#61628=CIRCLE ( 'NONE', #11292, 4.000000000000000000 ) ;
#61640=CARTESIAN_POINT ( 'NONE',  ( 20.00000000000000000, -7.500000000000000000, 29.75000000000000355 ) ) ;
#61661=CARTESIAN_POINT ( 'NONE',  ( -17.78205128205128105, -11.50000000000000000, 29.75000000000000355 ) ) ;
#61667=VECTOR ( 'NONE', #21972, 1000.000000000000000 ) ;
#61689=ORIENTED_EDGE ( 'NONE', *, *, #88080, .T. ) ;
#61705=LINE ( 'NONE', #55842, #9349 ) ;
#61731=DIRECTION ( 'NONE',  ( 0.000000000000000000, 0.000000000000000000, -1.000000000000000000 ) ) ;
#61733=LINE ( 'NONE', #15342, #5753 ) ;
#61735=EDGE_LOOP ( 'NONE', ( #27807, #30401, #63298, #15157, #80836, #40110, #78387, #75460, #51486, #82673, #12833, #9615, #57700, #32234, #11232, #69752, #78179, #70569, #66839, #56953, #72229, #24510, #71701, #41297, #59051, #9080, #67305, #49523, #26562, #41472, #62221, #70908, #11178, #78393, #87116, #26425, #75231, #66145, #87207, #58314, #26420, #38335, #46433, #84972, #61813, #19785, #53603, #72237, #2160, #4764, #19425, #56630, #14859, #76913, #47061, #41519, #70428, #36918, #61138, #55494, #54025, #60405, #34497, #29072, #30979, #75266, #29415, #70115, #39315, #6983, #72590, #68247, #31744, #40605, #21913, #46968, #82091, #41103, #68106, #51170, #18587, #56797, #4674, #19795, #75093, #55875, #48209, #25123, #60127, #46665, #73811, #54385, #65197, #26890, #51813 ) ) ;
#61745=DIRECTION ( 'NONE',  ( -1.000000000000000000, -0.000000000000000000, -0.000000000000000000 ) ) ;
#61754=DIRECTION ( 'NONE',  ( 1.000000000000000000, 0.000000000000000000, 0.000000000000000000 ) ) ;
#61755=CARTESIAN_POINT ( 'NONE',  ( 4.230769230769229061, -4.000000000000000000, 29.75000000000000355 ) ) ;
#61763=ORIENTED_EDGE ( 'NONE', *, *, #43683, .T. ) ;
#61767=ORIENTED_EDGE ( 'NONE', *, *, #39859, .F. ) ;
#61773=VERTEX_POINT ( 'NONE', #48233 ) ;
#61780=CARTESIAN_POINT ( 'NONE',  ( 9.070512820512819374, -7.500000000000000000, 29.75000000000000355 ) ) ;
#61799=VECTOR ( 'NONE', #41009, 1000.000000000000000 ) ;
#61813=ORIENTED_EDGE ( 'NONE', *, *, #53126, .T. ) ;
#61814=ORIENTED_EDGE ( 'NONE', *, *, #83855, .F. ) ;
#61830=VERTEX_POINT ( 'NONE', #63522 ) ;
#61832=ORIENTED_EDGE ( 'NONE', *, *, #15460, .T. ) ;
#61835=CARTESIAN_POINT ( 'NONE',  ( -9.320512820512821150, -1.926643599941765039, 29.65000000000000213 ) ) ;
#61836=DIRECTION ( 'NONE',  ( 0.000000000000000000, 0.000000000000000000, -1.000000000000000000 ) ) ;
#61854=FACE_OUTER_BOUND ( 'NONE', #78972, .T. ) ;
#61855=DIRECTION ( 'NONE',  ( -0.000000000000000000, 1.000000000000000000, -0.000000000000000000 ) ) ;
#61858=DIRECTION ( 'NONE',  ( -1.000000000000000000, -0.000000000000000000, 0.000000000000000000 ) ) ;
#61860=ORIENTED_EDGE ( 'NONE', *, *, #34410, .T. ) ;
#61862=ORIENTED_EDGE ( 'NONE', *, *, #76670, .T. ) ;
#61879=AXIS2_PLACEMENT_3D ( 'NONE', #6487, #21763, #20442 ) ;
#61880=VECTOR ( 'NONE', #16488, 1000.000000000000000 ) ;
#61882=VERTEX_POINT ( 'NONE', #31967 ) ;
#61889=AXIS2_PLACEMENT_3D ( 'NONE', #82266, #89037, #28649 ) ;
#61891=VECTOR ( 'NONE', #44633, 1000.000000000000000 ) ;
#61909=EDGE_CURVE ( 'NONE', #57687, #65753, #25650, .T. ) ;
#61914=LINE ( 'NONE', #82205, #25478 ) ;
#61926=ORIENTED_EDGE ( 'NONE', *, *, #85811, .F. ) ;
#61937=EDGE_CURVE ( 'NONE', #81881, #59129, #86483, .T. ) ;
#61956=FACE_OUTER_BOUND ( 'NONE', #46609, .T. ) ;
#61963=VERTEX_POINT ( 'NONE', #40511 ) ;
#61964=EDGE_CURVE ( 'NONE', #55273, #16936, #87824, .T. ) ;
#61966=ORIENTED_EDGE ( 'NONE', *, *, #18276, .T. ) ;
#61975=EDGE_CURVE ( 'NONE', #20924, #84442, #48566, .T. ) ;
#61986=VECTOR ( 'NONE', #57446, 1000.000000000000000 ) ;
#62009=VECTOR ( 'NONE', #68471, 1000.000000000000000 ) ;
#62021=FACE_OUTER_BOUND ( 'NONE', #52355, .T. ) ;
#62039=FACE_OUTER_BOUND ( 'NONE', #56480, .T. ) ;
#62059=CARTESIAN_POINT ( 'NONE',  ( 5.448717948717947124, -7.500000000000000000, 29.75000000000000355 ) ) ;
#62065=LINE ( 'NONE', #40047, #24580 ) ;
#62070=CARTESIAN_POINT ( 'NONE',  ( 2.294871794871793380, -11.00000000000000000, 29.75000000000000355 ) ) ;
#62075=VECTOR ( 'NONE', #26393, 1000.000000000000000 ) ;
#62081=DIRECTION ( 'NONE',  ( -1.000000000000000000, -0.000000000000000000, -0.000000000000000000 ) ) ;
#62084=DIRECTION ( 'NONE',  ( 1.000000000000000000, 0.000000000000000000, 0.000000000000000000 ) ) ;
#62095=DIRECTION ( 'NONE',  ( 1.000000000000000000, 0.000000000000000000, 0.000000000000000000 ) ) ;
#62100=FACE_BOUND ( 'NONE', #37281, .T. ) ;
#62110=CARTESIAN_POINT ( 'NONE',  ( 11.97435897435897267, -7.500000000000000000, 29.75000000000000355 ) ) ;
#62143=ORIENTED_EDGE ( 'NONE', *, *, #22053, .T. ) ;
#62162=ORIENTED_EDGE ( 'NONE', *, *, #51993, .T. ) ;
#62170=DIRECTION ( 'NONE',  ( -1.000000000000000000, -0.000000000000000000, -0.000000000000000000 ) ) ;
#62171=ORIENTED_EDGE ( 'NONE', *, *, #33556, .F. ) ;
#62185=LINE ( 'NONE', #5484, #19357 ) ;
#62189=ORIENTED_EDGE ( 'NONE', *, *, #77412, .F. ) ;
#62191=CARTESIAN_POINT ( 'NONE',  ( -1.576923076923076872, -7.500000000000000000, 29.75000000000000355 ) ) ;
#62193=CARTESIAN_POINT ( 'NONE',  ( 17.78205128205128105, -7.500000000000000000, 29.75000000000000355 ) ) ;
#62203=EDGE_LOOP ( 'NONE', ( #65849, #85416, #74507, #66990 ) ) ;
#62216=ORIENTED_EDGE ( 'NONE', *, *, #45903, .F. ) ;
#62221=ORIENTED_EDGE ( 'NONE', *, *, #81321, .T. ) ;
#62222=CARTESIAN_POINT ( 'NONE',  ( 11.25641025641025550, -7.500000000000000000, 29.75000000000000355 ) ) ;
#62224=LINE ( 'NONE', #82952, #68782 ) ;
#62225=CARTESIAN_POINT ( 'NONE',  ( 15.12820512820512953, -3.499999999999999556, 29.75000000000000355 ) ) ;
#62233=DIRECTION ( 'NONE',  ( -0.000000000000000000, 1.000000000000000000, -0.000000000000000000 ) ) ;
#62237=DIRECTION ( 'NONE',  ( 0.000000000000000000, 0.000000000000000000, -1.000000000000000000 ) ) ;
#62258=EDGE_LOOP ( 'NONE', ( #58286, #76240, #17948, #62143 ) ) ;
#62261=DIRECTION ( 'NONE',  ( 1.000000000000000000, 0.000000000000000000, 0.000000000000000000 ) ) ;
#62278=LINE ( 'NONE', #7794, #2979 ) ;
#62279=ORIENTED_EDGE ( 'NONE', *, *, #13025, .F. ) ;
#62290=VECTOR ( 'NONE', #49577, 1000.000000000000000 ) ;
#62295=CARTESIAN_POINT ( 'NONE',  ( 5.448717948717947124, -4.000000000000000000, 29.75000000000000355 ) ) ;
#62309=CARTESIAN_POINT ( 'NONE',  ( -8.352564102564102200, -3.499999999999999556, 29.75000000000000355 ) ) ;
#62312=CARTESIAN_POINT ( 'NONE',  ( -18.75000000000000000, -7.500000000000000000, 29.75000000000000355 ) ) ;
#62317=ADVANCED_FACE ( 'NONE', ( #41171 ), #34404, .T. ) ;
#62318=VECTOR ( 'NONE', #87533, 1000.000000000000000 ) ;
#62319=EDGE_CURVE ( 'NONE', #27068, #32893, #7388, .T. ) ;
#62320=CARTESIAN_POINT ( 'NONE',  ( -6.416666666666667851, -7.500000000000000000, 29.75000000000000355 ) ) ;
#62323=CIRCLE ( 'NONE', #6283, 4.000000000000000000 ) ;
#62374=CARTESIAN_POINT ( 'NONE',  ( -8.102564102564102200, -7.500000000000000000, 33.75000000000000000 ) ) ;
#62375=VERTEX_POINT ( 'NONE', #62309 ) ;
#62378=CARTESIAN_POINT ( 'NONE',  ( -10.03846153846153832, -7.500000000000000000, 29.75000000000000355 ) ) ;
#62410=FACE_OUTER_BOUND ( 'NONE', #85952, .T. ) ;
#62417=EDGE_CURVE ( 'NONE', #71459, #70755, #73012, .T. ) ;
#62421=DIRECTION ( 'NONE',  ( 1.000000000000000000, 0.000000000000000000, 0.000000000000000000 ) ) ;
#62434=VECTOR ( 'NONE', #20055, 1000.000000000000000 ) ;
#62441=LINE ( 'NONE', #14271, #35718 ) ;
#62443=ADVANCED_FACE ( 'NONE', ( #39241 ), #38788, .F. ) ;
#62446=ORIENTED_EDGE ( 'NONE', *, *, #67467, .F. ) ;
#62448=VERTEX_POINT ( 'NONE', #11308 ) ;
#62455=ADVANCED_FACE ( 'NONE', ( #19400 ), #74351, .F. ) ;
#62457=ADVANCED_FACE ( 'NONE', ( #25270 ), #19843, .T. ) ;
#62463=AXIS2_PLACEMENT_3D ( 'NONE', #66731, #37470, #24846 ) ;
#62469=DIRECTION ( 'NONE',  ( 0.000000000000000000, 0.000000000000000000, -1.000000000000000000 ) ) ;
#62471=CARTESIAN_POINT ( 'NONE',  ( 20.00000000000000000, -4.000000000000000000, 29.75000000000000355 ) ) ;
#62472=DIRECTION ( 'NONE',  ( -0.000000000000000000, 1.000000000000000000, -0.000000000000000000 ) ) ;
#62479=FACE_OUTER_BOUND ( 'NONE', #53846, .T. ) ;
#62491=ORIENTED_EDGE ( 'NONE', *, *, #52784, .F. ) ;
#62506=VECTOR ( 'NONE', #39915, 1000.000000000000000 ) ;
#62510=PLANE ( 'NONE',  #78353 ) ;
#62518=DIRECTION ( 'NONE',  ( 0.000000000000000000, 0.000000000000000000, 1.000000000000000000 ) ) ;
#62524=ORIENTED_EDGE ( 'NONE', *, *, #88551, .F. ) ;
#62541=PLANE ( 'NONE',  #27028 ) ;
#62551=ORIENTED_EDGE ( 'NONE', *, *, #6990, .F. ) ;
#62556=CARTESIAN_POINT ( 'NONE',  ( 2.544871794871792936, -3.499999999999999556, 29.75000000000000355 ) ) ;
#62576=EDGE_CURVE ( 'NONE', #58816, #50855, #41899, .T. ) ;
#62593=EDGE_LOOP ( 'NONE', ( #10131, #8649, #16072, #60906, #68614, #4495, #57028 ) ) ;
#62604=LINE ( 'NONE', #77023, #73468 ) ;
#62605=EDGE_CURVE ( 'NONE', #58964, #51776, #10899, .T. ) ;
#62640=FACE_OUTER_BOUND ( 'NONE', #53884, .T. ) ;
#62643=CARTESIAN_POINT ( 'NONE',  ( -16.09615384615384670, -4.000000000000000000, 29.75000000000000355 ) ) ;
#62667=LINE ( 'NONE', #981, #19582 ) ;
#62672=CARTESIAN_POINT ( 'NONE',  ( -16.81410256410256565, -3.499999999999999556, 29.75000000000000355 ) ) ;
#62676=DIRECTION ( 'NONE',  ( 0.000000000000000000, 0.000000000000000000, 1.000000000000000000 ) ) ;
#62677=LINE ( 'NONE', #19487, #66675 ) ;
#62680=ORIENTED_EDGE ( 'NONE', *, *, #24545, .T. ) ;
#62689=LINE ( 'NONE', #35691, #66762 ) ;
#62694=EDGE_CURVE ( 'NONE', #23520, #58603, #5920, .T. ) ;
#62697=UNCERTAINTY_MEASURE_WITH_UNIT (LENGTH_MEASURE( 1.000000000000000082E-05 ), #39608, 'distance_accuracy_value', 'NONE');
#62698=CARTESIAN_POINT ( 'NONE',  ( -11.25641025641025550, -7.500000000000000000, 29.75000000000000355 ) ) ;
#62705=ADVANCED_FACE ( 'NONE', ( #52760 ), #53657, .F. ) ;
#62722=DIRECTION ( 'NONE',  ( -1.000000000000000000, -0.000000000000000000, -0.000000000000000000 ) ) ;
#62724=ORIENTED_EDGE ( 'NONE', *, *, #18276, .F. ) ;
#62728=EDGE_LOOP ( 'NONE', ( #31148, #89132, #71027, #2855, #32095 ) ) ;
#62760=ORIENTED_EDGE ( 'NONE', *, *, #64924, .F. ) ;
#62763=CARTESIAN_POINT ( 'NONE',  ( 0.000000000000000000, 0.000000000000000000, 0.000000000000000000 ) ) ;
#62767=VECTOR ( 'NONE', #48028, 1000.000000000000000 ) ;
#62775=ADVANCED_FACE ( 'NONE', ( #81145 ), #19430, .T. ) ;
#62792=ORIENTED_EDGE ( 'NONE', *, *, #40514, .F. ) ;
#62816=DIRECTION ( 'NONE',  ( 1.000000000000000000, 0.000000000000000000, 0.000000000000000000 ) ) ;
#62827=CARTESIAN_POINT ( 'NONE',  ( -3.512820512820514995, -3.499999999999999556, 29.75000000000000355 ) ) ;
#62836=ORIENTED_EDGE ( 'NONE', *, *, #15271, .F. ) ;
#62845=LINE ( 'NONE', #76379, #47481 ) ;
#62855=VECTOR ( 'NONE', #80502, 1000.000000000000000 ) ;
#62861=CARTESIAN_POINT ( 'NONE',  ( -15.84615384615384670, -3.499999999999999556, 29.75000000000000355 ) ) ;
#62870=DIRECTION ( 'NONE',  ( 1.000000000000000000, 0.000000000000000000, 0.000000000000000000 ) ) ;
#62888=VERTEX_POINT ( 'NONE', #22091 ) ;
#62901=ORIENTED_EDGE ( 'NONE', *, *, #76854, .F. ) ;
#62912=CARTESIAN_POINT ( 'NONE',  ( 2.294871794871793824, -4.000000000000000000, 29.75000000000000355 ) ) ;
#62922=LINE ( 'NONE', #34137, #9291 ) ;
#62929=FACE_OUTER_BOUND ( 'NONE', #85938, .T. ) ;
#62935=CARTESIAN_POINT ( 'NONE',  ( 20.00000000000000000, -4.000000000000000000, 29.75000000000000355 ) ) ;
#62941=AXIS2_PLACEMENT_3D ( 'NONE', #70688, #69365, #7666 ) ;
#62949=CARTESIAN_POINT ( 'NONE',  ( 20.00000000000000000, -11.50000000000000000, 29.75000000000000355 ) ) ;
#62968=EDGE_CURVE ( 'NONE', #77757, #30410, #36495, .T. ) ;
#62970=DIRECTION ( 'NONE',  ( -0.000000000000000000, 1.000000000000000000, -0.000000000000000000 ) ) ;
#62972=DIRECTION ( 'NONE',  ( 1.000000000000000000, 0.000000000000000000, 0.000000000000000000 ) ) ;
#62992=FACE_OUTER_BOUND ( 'NONE', #78301, .T. ) ;
#62993=DIRECTION ( 'NONE',  ( -0.000000000000000000, 0.000000000000000000, 1.000000000000000000 ) ) ;
#63001=VECTOR ( 'NONE', #15877, 1000.000000000000000 ) ;
#63021=FACE_OUTER_BOUND ( 'NONE', #4049, .T. ) ;
#63023=EDGE_CURVE ( 'NONE', #15955, #12463, #16647, .T. ) ;
#63032=EDGE_LOOP ( 'NONE', ( #24297, #70453, #61763, #22084 ) ) ;
#63034=CIRCLE ( 'NONE', #31429, 4.000000000000000000 ) ;
#63042=ORIENTED_EDGE ( 'NONE', *, *, #72553, .F. ) ;
#63049=VERTEX_POINT ( 'NONE', #50431 ) ;
#63052=ORIENTED_EDGE ( 'NONE', *, *, #47248, .T. ) ;
#63059=CARTESIAN_POINT ( 'NONE',  ( 0.000000000000000000, -4.000000000000000000, 29.75000000000000355 ) ) ;
#63079=AXIS2_PLACEMENT_3D ( 'NONE', #34150, #61617, #69270 ) ;
#63085=ORIENTED_EDGE ( 'NONE', *, *, #27938, .T. ) ;
#63123=ORIENTED_EDGE ( 'NONE', *, *, #26438, .T. ) ;
#63124=ORIENTED_EDGE ( 'NONE', *, *, #82460, .T. ) ;
#63138=DIRECTION ( 'NONE',  ( -1.000000000000000000, -0.000000000000000000, -0.000000000000000000 ) ) ;
#63140=ORIENTED_EDGE ( 'NONE', *, *, #72074, .T. ) ;
#63145=DIRECTION ( 'NONE',  ( -1.000000000000000000, -0.000000000000000000, -0.000000000000000000 ) ) ;
#63154=CARTESIAN_POINT ( 'NONE',  ( -19.50000000000000000, -3.499999999999999556, 29.75000000000000355 ) ) ;
#63156=CARTESIAN_POINT ( 'NONE',  ( 17.06410256410256565, -7.500000000000000000, 33.75000000000000000 ) ) ;
#63159=EDGE_CURVE ( 'NONE', #25471, #43749, #21082, .T. ) ;
#63172=LINE ( 'NONE', #49228, #18819 ) ;
#63174=VECTOR ( 'NONE', #51034, 1000.000000000000000 ) ;
#63178=VECTOR ( 'NONE', #73524, 1000.000000000000000 ) ;
#63209=AXIS2_PLACEMENT_3D ( 'NONE', #8019, #51073, #71359 ) ;
#63212=ORIENTED_EDGE ( 'NONE', *, *, #55000, .T. ) ;
#63219=EDGE_CURVE ( 'NONE', #42018, #62448, #30068, .T. ) ;
#63229=LINE ( 'NONE', #83078, #4607 ) ;
#63231=VECTOR ( 'NONE', #60587, 1000.000000000000000 ) ;
#63237=CIRCLE ( 'NONE', #24400, 0.5000000000000004441 ) ;
#63238=VECTOR ( 'NONE', #71783, 1000.000000000000000 ) ;
#63252=DIRECTION ( 'NONE',  ( -0.000000000000000000, 1.000000000000000000, -0.000000000000000000 ) ) ;
#63253=ORIENTED_EDGE ( 'NONE', *, *, #55353, .F. ) ;
#63274=DIRECTION ( 'NONE',  ( 1.000000000000000000, 0.000000000000000000, 0.000000000000000000 ) ) ;
#63280=FACE_OUTER_BOUND ( 'NONE', #16250, .T. ) ;
#63286=VECTOR ( 'NONE', #45118, 1000.000000000000000 ) ;
#63298=ORIENTED_EDGE ( 'NONE', *, *, #16220, .F. ) ;
#63307=CARTESIAN_POINT ( 'NONE',  ( -9.320512820512821150, -7.500000000000000000, 29.75000000000000355 ) ) ;
#63310=CARTESIAN_POINT ( 'NONE',  ( -15.12820512820512953, -3.499999999999999556, 29.75000000000000355 ) ) ;
#63312=CARTESIAN_POINT ( 'NONE',  ( -14.16025641025641235, -4.000000000000000000, 29.75000000000000355 ) ) ;
#63313=VECTOR ( 'NONE', #29014, 1000.000000000000000 ) ;
#63324=DIRECTION ( 'NONE',  ( -1.000000000000000000, -0.000000000000000000, -0.000000000000000000 ) ) ;
#63329=FACE_OUTER_BOUND ( 'NONE', #10280, .T. ) ;
#63336=DIRECTION ( 'NONE',  ( -0.000000000000000000, 1.000000000000000000, -0.000000000000000000 ) ) ;
#63361=ORIENTED_EDGE ( 'NONE', *, *, #16712, .T. ) ;
#63367=CARTESIAN_POINT ( 'NONE',  ( -14.16025641025641058, -3.499999999999999556, 29.75000000000000355 ) ) ;
#63372=DIRECTION ( 'NONE',  ( -1.000000000000000000, -0.000000000000000000, -0.000000000000000000 ) ) ;
#63387=DIRECTION ( 'NONE',  ( -1.000000000000000000, -0.000000000000000000, 0.000000000000000000 ) ) ;
#63390=LINE ( 'NONE', #62935, #17383 ) ;
#63412=LINE ( 'NONE', #64288, #55405 ) ;
#63415=AXIS2_PLACEMENT_3D ( 'NONE', #28965, #22192, #83010 ) ;
#63438=FACE_OUTER_BOUND ( 'NONE', #8005, .T. ) ;
#63439=EDGE_CURVE ( 'NONE', #30233, #52641, #80031, .T. ) ;
#63440=FACE_OUTER_BOUND ( 'NONE', #42746, .T. ) ;
#63442=EDGE_CURVE ( 'NONE', #80730, #11720, #33621, .T. ) ;
#63443=ORIENTED_EDGE ( 'NONE', *, *, #77262, .F. ) ;
#63451=PLANE ( 'NONE',  #3488 ) ;
#63464=ORIENTED_EDGE ( 'NONE', *, *, #33015, .T. ) ;
#63467=DIRECTION ( 'NONE',  ( 1.000000000000000000, 0.000000000000000000, 0.000000000000000000 ) ) ;
#63468=EDGE_CURVE ( 'NONE', #51615, #65753, #68289, .T. ) ;
#63484=EDGE_LOOP ( 'NONE', ( #59652, #4074, #6319, #24592, #32393, #70541, #17170 ) ) ;
#63496=ORIENTED_EDGE ( 'NONE', *, *, #33312, .F. ) ;
#63506=DIRECTION ( 'NONE',  ( -1.000000000000000000, 0.000000000000000000, -0.000000000000000000 ) ) ;
#63521=AXIS2_PLACEMENT_3D ( 'NONE', #21837, #76785, #1565 ) ;
#63522=CARTESIAN_POINT ( 'NONE',  ( 2.544871794871792936, -7.500000000000000000, 33.75000000000000000 ) ) ;
#63539=DIRECTION ( 'NONE',  ( 1.000000000000000000, 0.000000000000000000, 0.000000000000000000 ) ) ;
#63557=CARTESIAN_POINT ( 'NONE',  ( -17.06410256410256565, -3.499999999999999556, 29.75000000000000355 ) ) ;
#63569=EDGE_CURVE ( 'NONE', #19556, #23382, #24087, .T. ) ;
#63576=AXIS2_PLACEMENT_3D ( 'NONE', #85120, #51744, #78792 ) ;
#63587=DIRECTION ( 'NONE',  ( -1.000000000000000000, 0.000000000000000000, -0.000000000000000000 ) ) ;
#63589=PLANE ( 'NONE',  #31798 ) ;
#63595=CYLINDRICAL_SURFACE ( 'NONE', #66245, 4.000000000000000000 ) ;
#63602=CARTESIAN_POINT ( 'NONE',  ( -2.544871794871794268, -3.499999999999999556, 29.75000000000000355 ) ) ;
#63612=VECTOR ( 'NONE', #69278, 1000.000000000000000 ) ;
#63623=VECTOR ( 'NONE', #66442, 1000.000000000000000 ) ;
#63639=DIRECTION ( 'NONE',  ( -0.000000000000000000, 1.000000000000000000, -0.000000000000000000 ) ) ;
#63640=ORIENTED_EDGE ( 'NONE', *, *, #27657, .F. ) ;
#63649=CIRCLE ( 'NONE', #24809, 4.000000000000000000 ) ;
#63652=LINE ( 'NONE', #57341, #41977 ) ;
#63666=PLANE ( 'NONE',  #67942 ) ;
#63699=AXIS2_PLACEMENT_3D ( 'NONE', #35404, #55668, #293 ) ;
#63715=DIRECTION ( 'NONE',  ( 1.000000000000000000, 0.000000000000000000, 0.000000000000000000 ) ) ;
#63721=CYLINDRICAL_SURFACE ( 'NONE', #51316, 4.000000000000000000 ) ;
#63723=DIRECTION ( 'NONE',  ( 0.000000000000000000, 0.000000000000000000, -1.000000000000000000 ) ) ;
#63731=LINE ( 'NONE', #49341, #48716 ) ;
#63740=CIRCLE ( 'NONE', #27801, 4.000000000000000000 ) ;
#63742=VERTEX_POINT ( 'NONE', #21775 ) ;
#63745=VERTEX_POINT ( 'NONE', #55554 ) ;
#63758=LINE ( 'NONE', #16467, #75228 ) ;
#63761=CARTESIAN_POINT ( 'NONE',  ( 19.00000000000000000, -11.00000000000000000, 29.75000000000000355 ) ) ;
#63793=CIRCLE ( 'NONE', #75323, 4.000000000000000000 ) ;
#63804=DIRECTION ( 'NONE',  ( -0.000000000000000000, 1.000000000000000000, -0.000000000000000000 ) ) ;
#63876=DIRECTION ( 'NONE',  ( 0.000000000000000000, 0.000000000000000000, -1.000000000000000000 ) ) ;
#63880=DIRECTION ( 'NONE',  ( 1.000000000000000000, 0.000000000000000000, 0.000000000000000000 ) ) ;
#63881=DIRECTION ( 'NONE',  ( -0.000000000000000000, 1.000000000000000000, -0.000000000000000000 ) ) ;
#63887=CARTESIAN_POINT ( 'NONE',  ( 3.262820512820510999, -7.500000000000000000, 29.75000000000000355 ) ) ;
#63893=ORIENTED_EDGE ( 'NONE', *, *, #24636, .F. ) ;
#63906=ORIENTED_EDGE ( 'NONE', *, *, #52809, .T. ) ;
#63907=ADVANCED_FACE ( 'NONE', ( #85582 ), #17573, .F. ) ;
#63916=AXIS2_PLACEMENT_3D ( 'NONE', #45684, #17779, #10572 ) ;
#63918=CARTESIAN_POINT ( 'NONE',  ( 20.00000000000000000, -4.000000000000000000, 29.75000000000000355 ) ) ;
#63933=ADVANCED_FACE ( 'NONE', ( #4034 ), #72952, .T. ) ;
#63948=DIRECTION ( 'NONE',  ( -0.000000000000000000, 1.000000000000000000, -0.000000000000000000 ) ) ;
#63976=ADVANCED_FACE ( 'NONE', ( #86944 ), #79718, .T. ) ;
#63981=CARTESIAN_POINT ( 'NONE',  ( 9.320512820512821150, -7.500000000000000000, 29.75000000000000355 ) ) ;
#63987=CARTESIAN_POINT ( 'NONE',  ( 20.00000000000000000, -3.499999999999999556, 28.25000000000000000 ) ) ;
#63992=PLANE ( 'NONE',  #82419 ) ;
#63997=VERTEX_POINT ( 'NONE', #9916 ) ;
#64005=DIRECTION ( 'NONE',  ( 1.000000000000000000, 0.000000000000000000, 0.000000000000000000 ) ) ;
#64008=CIRCLE ( 'NONE', #20888, 4.000000000000000000 ) ;
#64014=EDGE_CURVE ( 'NONE', #74179, #73852, #81500, .T. ) ;
#64028=CARTESIAN_POINT ( 'NONE',  ( -13.91025641025641058, -7.500000000000000000, 29.75000000000000355 ) ) ;
#64053=AXIS2_PLACEMENT_3D ( 'NONE', #57053, #84106, #77331 ) ;
#64088=DIRECTION ( 'NONE',  ( -1.000000000000000000, -0.000000000000000000, -0.000000000000000000 ) ) ;
#64089=DIRECTION ( 'NONE',  ( 0.000000000000000000, 0.000000000000000000, -1.000000000000000000 ) ) ;
#64104=LINE ( 'NONE', #37073, #12699 ) ;
#64110=LINE ( 'NONE', #82642, #37843 ) ;
#64116=ORIENTED_EDGE ( 'NONE', *, *, #67467, .T. ) ;
#64119=LINE ( 'NONE', #23584, #50243 ) ;
#64127=VERTEX_POINT ( 'NONE', #8492 ) ;
#64141=EDGE_CURVE ( 'NONE', #45062, #86240, #15434, .T. ) ;
#64155=DIRECTION ( 'NONE',  ( 0.000000000000000000, 0.000000000000000000, -1.000000000000000000 ) ) ;
#64157=PLANE ( 'NONE',  #31419 ) ;
#64162=LINE ( 'NONE', #85794, #44574 ) ;
#64183=DIRECTION ( 'NONE',  ( 0.000000000000000000, 0.000000000000000000, -1.000000000000000000 ) ) ;
#64203=CARTESIAN_POINT ( 'NONE',  ( 17.06410256410256565, -3.499999999999999556, 29.75000000000000355 ) ) ;
#64218=EDGE_CURVE ( 'NONE', #79996, #80137, #29648, .T. ) ;
#64220=VERTEX_POINT ( 'NONE', #24653 ) ;
#64224=PLANE ( 'NONE',  #68965 ) ;
#64234=CARTESIAN_POINT ( 'NONE',  ( -14.87820512820512953, -4.000000000000000000, 29.75000000000000355 ) ) ;
#64235=LINE ( 'NONE', #2538, #7193 ) ;
#64241=VERTEX_POINT ( 'NONE', #22874 ) ;
#64245=LINE ( 'NONE', #9332, #84009 ) ;
#64257=EDGE_CURVE ( 'NONE', #71435, #9433, #72389, .T. ) ;
#64268=AXIS2_PLACEMENT_3D ( 'NONE', #37830, #44128, #31974 ) ;
#64269=FACE_OUTER_BOUND ( 'NONE', #47228, .T. ) ;
#64270=DIRECTION ( 'NONE',  ( -1.000000000000000000, -0.000000000000000000, -0.000000000000000000 ) ) ;
#64271=LINE ( 'NONE', #9355, #63612 ) ;
#64288=CARTESIAN_POINT ( 'NONE',  ( -19.50000000000000000, -11.50000000000000000, 29.75000000000000355 ) ) ;
#64301=ORIENTED_EDGE ( 'NONE', *, *, #71995, .F. ) ;
#64306=EDGE_CURVE ( 'NONE', #77909, #46953, #53904, .T. ) ;
#64311=VERTEX_POINT ( 'NONE', #47589 ) ;
#64316=DIRECTION ( 'NONE',  ( -1.000000000000000000, 0.000000000000000000, -0.000000000000000000 ) ) ;
#64320=VECTOR ( 'NONE', #75898, 1000.000000000000000 ) ;
#64329=CIRCLE ( 'NONE', #60034, 4.000000000000000000 ) ;
#64343=VECTOR ( 'NONE', #12758, 1000.000000000000000 ) ;
#64347=DIRECTION ( 'NONE',  ( -1.000000000000000000, 0.000000000000000000, -0.000000000000000000 ) ) ;
#64364=CARTESIAN_POINT ( 'NONE',  ( -19.50000000000000000, -11.50000000000000000, 29.75000000000000355 ) ) ;
#64380=DIRECTION ( 'NONE',  ( 0.000000000000000000, 1.000000000000000000, -0.000000000000000000 ) ) ;
#64389=ORIENTED_EDGE ( 'NONE', *, *, #69448, .F. ) ;
#64399=CARTESIAN_POINT ( 'NONE',  ( 0.000000000000000000, -11.00000000000000000, 29.25000000000000000 ) ) ;
#64401=VERTEX_POINT ( 'NONE', #33639 ) ;
#64405=EDGE_CURVE ( 'NONE', #29561, #78266, #72972, .T. ) ;
#64425=LINE ( 'NONE', #43292, #88947 ) ;
#64457=CYLINDRICAL_SURFACE ( 'NONE', #56092, 4.000000000000000000 ) ;
#64463=ORIENTED_EDGE ( 'NONE', *, *, #85198, .T. ) ;
#64464=CARTESIAN_POINT ( 'NONE',  ( 20.00000000000000000, -4.000000000000000000, 29.75000000000000355 ) ) ;
#64476=AXIS2_PLACEMENT_3D ( 'NONE', #48884, #56533, #77243 ) ;
#64485=LINE ( 'NONE', #50541, #63286 ) ;
#64487=ADVANCED_FACE ( 'NONE', ( #20993 ), #83159, .F. ) ;
#64504=AXIS2_PLACEMENT_3D ( 'NONE', #41487, #68953, #7263 ) ;
#64505=ORIENTED_EDGE ( 'NONE', *, *, #83864, .F. ) ;
#64507=DIRECTION ( 'NONE',  ( 1.000000000000000000, 0.000000000000000000, 0.000000000000000000 ) ) ;
#64516=DIRECTION ( 'NONE',  ( -1.000000000000000000, -0.000000000000000000, 0.000000000000000000 ) ) ;
#64521=CARTESIAN_POINT ( 'NONE',  ( 3.512820512820510555, -7.500000000000000000, 29.75000000000000355 ) ) ;
#64522=VECTOR ( 'NONE', #32380, 1000.000000000000000 ) ;
#64526=ORIENTED_EDGE ( 'NONE', *, *, #36001, .T. ) ;
#64531=CARTESIAN_POINT ( 'NONE',  ( -10.03846153846153832, -1.926643599941765039, 29.65000000000000213 ) ) ;
#64534=ORIENTED_EDGE ( 'NONE', *, *, #70661, .T. ) ;
#64541=CARTESIAN_POINT ( 'NONE',  ( -1.576923076923076872, -7.500000000000000000, 33.75000000000000000 ) ) ;
#64542=EDGE_CURVE ( 'NONE', #39901, #48658, #7652, .T. ) ;
#64548=EDGE_CURVE ( 'NONE', #47272, #13621, #76393, .T. ) ;
#64551=EDGE_LOOP ( 'NONE', ( #37881, #51898, #83860, #22901 ) ) ;
#64561=AXIS2_PLACEMENT_3D ( 'NONE', #34438, #40764, #39882 ) ;
#64586=ORIENTED_EDGE ( 'NONE', *, *, #80249, .F. ) ;
#64591=DIRECTION ( 'NONE',  ( -0.000000000000000000, 1.000000000000000000, -0.000000000000000000 ) ) ;
#64594=ORIENTED_EDGE ( 'NONE', *, *, #17674, .F. ) ;
#64595=EDGE_CURVE ( 'NONE', #6322, #7995, #14695, .T. ) ;
#64600=FACE_OUTER_BOUND ( 'NONE', #6732, .T. ) ;
#64616=EDGE_LOOP ( 'NONE', ( #59518, #79908, #42632, #43 ) ) ;
#64632=LINE ( 'NONE', #43493, #75087 ) ;
#64633=EDGE_CURVE ( 'NONE', #34232, #88674, #63758, .T. ) ;
#64636=AXIS2_PLACEMENT_3D ( 'NONE', #72346, #46216, #10656 ) ;
#64649=EDGE_LOOP ( 'NONE', ( #66020, #17358, #28074, #17008 ) ) ;
#64680=LINE ( 'NONE', #36345, #43587 ) ;
#64685=VECTOR ( 'NONE', #27075, 1000.000000000000000 ) ;
#64690=DIRECTION ( 'NONE',  ( 0.000000000000000000, 0.000000000000000000, -1.000000000000000000 ) ) ;
#64702=AXIS2_PLACEMENT_3D ( 'NONE', #47356, #60876, #39734 ) ;
#64714=CARTESIAN_POINT ( 'NONE',  ( 15.12820512820512953, -7.500000000000000000, 29.75000000000000355 ) ) ;
#64716=FACE_OUTER_BOUND ( 'NONE', #65555, .T. ) ;
#64729=CARTESIAN_POINT ( 'NONE',  ( -2.544871794871794268, -3.499999999999999556, 29.75000000000000355 ) ) ;
#64732=DIRECTION ( 'NONE',  ( -1.000000000000000000, -0.000000000000000000, -0.000000000000000000 ) ) ;
#64737=VECTOR ( 'NONE', #52213, 1000.000000000000000 ) ;
#64761=ORIENTED_EDGE ( 'NONE', *, *, #10581, .F. ) ;
#64762=CIRCLE ( 'NONE', #83506, 4.000000000000000000 ) ;
#64764=DIRECTION ( 'NONE',  ( 0.000000000000000000, 0.000000000000000000, -1.000000000000000000 ) ) ;
#64768=AXIS2_PLACEMENT_3D ( 'NONE', #48529, #28721, #68370 ) ;
#64772=VERTEX_POINT ( 'NONE', #12380 ) ;
#64775=ADVANCED_FACE ( 'NONE', ( #19573 ), #52904, .F. ) ;
#64787=CARTESIAN_POINT ( 'NONE',  ( -6.416666666666667851, -4.000000000000000000, 29.75000000000000355 ) ) ;
#64805=EDGE_CURVE ( 'NONE', #1878, #75410, #46608, .T. ) ;
#64808=DIRECTION ( 'NONE',  ( 0.000000000000000000, 0.000000000000000000, -1.000000000000000000 ) ) ;
#64810=ORIENTED_EDGE ( 'NONE', *, *, #23529, .F. ) ;
#64811=DIRECTION ( 'NONE',  ( -0.000000000000000000, 1.000000000000000000, -0.000000000000000000 ) ) ;
#64816=LINE ( 'NONE', #86914, #51033 ) ;
#64830=EDGE_CURVE ( 'NONE', #21320, #16624, #11944, .T. ) ;
#64831=VECTOR ( 'NONE', #19092, 1000.000000000000000 ) ;
#64834=DIRECTION ( 'NONE',  ( -0.000000000000000000, 1.000000000000000000, -0.000000000000000000 ) ) ;
#64842=CARTESIAN_POINT ( 'NONE',  ( -12.94230769230769162, -11.50000000000000000, 29.75000000000000355 ) ) ;
#64860=ORIENTED_EDGE ( 'NONE', *, *, #43695, .T. ) ;
#64866=DIRECTION ( 'NONE',  ( 0.000000000000000000, 0.000000000000000000, -1.000000000000000000 ) ) ;
#64867=VECTOR ( 'NONE', #34079, 1000.000000000000000 ) ;
#64873=DIRECTION ( 'NONE',  ( 0.000000000000000000, 0.000000000000000000, -1.000000000000000000 ) ) ;
#64917=VECTOR ( 'NONE', #85211, 1000.000000000000000 ) ;
#64924=EDGE_CURVE ( 'NONE', #38748, #72142, #73817, .T. ) ;
#64936=ORIENTED_EDGE ( 'NONE', *, *, #36653, .F. ) ;
#64962=CARTESIAN_POINT ( 'NONE',  ( 10.28846153846153832, -3.499999999999999556, 29.75000000000000355 ) ) ;
#64966=CARTESIAN_POINT ( 'NONE',  ( 0.000000000000000000, -11.00000000000000000, 29.75000000000000355 ) ) ;
#65023=ORIENTED_EDGE ( 'NONE', *, *, #26876, .F. ) ;
#65029=DIRECTION ( 'NONE',  ( -1.000000000000000000, -0.000000000000000000, -0.000000000000000000 ) ) ;
#65043=CARTESIAN_POINT ( 'NONE',  ( 3.512820512820510555, -7.500000000000000000, 29.75000000000000355 ) ) ;
#65050=CARTESIAN_POINT ( 'NONE',  ( 3.512820512820510555, -7.500000000000000000, 29.75000000000000355 ) ) ;
#65058=ORIENTED_EDGE ( 'NONE', *, *, #32395, .T. ) ;
#65074=CARTESIAN_POINT ( 'NONE',  ( -19.50000000000000000, -3.499999999999999556, 29.75000000000000355 ) ) ;
#65078=LINE ( 'NONE', #10154, #18981 ) ;
#65088=CARTESIAN_POINT ( 'NONE',  ( 20.00000000000000000, -4.000000000000000000, 29.75000000000000355 ) ) ;
#65103=ADVANCED_FACE ( 'NONE', ( #51003 ), #84390, .T. ) ;
#65163=FACE_OUTER_BOUND ( 'NONE', #11047, .T. ) ;
#65174=DIRECTION ( 'NONE',  ( 0.000000000000000000, 0.000000000000000000, -1.000000000000000000 ) ) ;
#65179=AXIS2_PLACEMENT_3D ( 'NONE', #13411, #40460, #62469 ) ;
#65187=DIRECTION ( 'NONE',  ( -0.000000000000000000, 1.000000000000000000, -0.000000000000000000 ) ) ;
#65191=FACE_OUTER_BOUND ( 'NONE', #13549, .T. ) ;
#65197=ORIENTED_EDGE ( 'NONE', *, *, #71669, .F. ) ;
#65208=EDGE_LOOP ( 'NONE', ( #22478, #64505, #2307, #34288 ) ) ;
#65212=ORIENTED_EDGE ( 'NONE', *, *, #46037, .F. ) ;
#65238=FACE_OUTER_BOUND ( 'NONE', #9902, .T. ) ;
#65250=DIRECTION ( 'NONE',  ( 1.000000000000000000, 0.000000000000000000, 0.000000000000000000 ) ) ;
#65258=DIRECTION ( 'NONE',  ( 1.000000000000000000, 0.000000000000000000, 0.000000000000000000 ) ) ;
#65260=ORIENTED_EDGE ( 'NONE', *, *, #62605, .F. ) ;
#65261=DIRECTION ( 'NONE',  ( 1.000000000000000000, 0.000000000000000000, 0.000000000000000000 ) ) ;
#65263=VECTOR ( 'NONE', #56602, 1000.000000000000000 ) ;
#65272=ORIENTED_EDGE ( 'NONE', *, *, #36986, .F. ) ;
#65273=EDGE_CURVE ( 'NONE', #24805, #6496, #55462, .T. ) ;
#65278=ORIENTED_EDGE ( 'NONE', *, *, #25018, .T. ) ;
#65280=CARTESIAN_POINT ( 'NONE',  ( -19.50000000000000000, -11.00000000000000000, 29.75000000000000355 ) ) ;
#65292=DIRECTION ( 'NONE',  ( -1.000000000000000000, -0.000000000000000000, -0.000000000000000000 ) ) ;
#65296=CARTESIAN_POINT ( 'NONE',  ( -19.50000000000000000, -3.499999999999999556, 29.75000000000000355 ) ) ;
#65302=CARTESIAN_POINT ( 'NONE',  ( 20.00000000000000000, -11.50000000000000000, 28.25000000000000000 ) ) ;
#65315=LINE ( 'NONE', #84728, #80901 ) ;
#65320=ORIENTED_EDGE ( 'NONE', *, *, #3770, .F. ) ;
#65323=ORIENTED_EDGE ( 'NONE', *, *, #19505, .F. ) ;
#65324=FACE_OUTER_BOUND ( 'NONE', #43408, .T. ) ;
#65353=ADVANCED_FACE ( 'NONE', ( #50033 ), #15821, .T. ) ;
#65358=ORIENTED_EDGE ( 'NONE', *, *, #17708, .F. ) ;
#65359=CARTESIAN_POINT ( 'NONE',  ( -8.102564102564102200, -11.00000000000000000, 29.75000000000000355 ) ) ;
#65365=DIRECTION ( 'NONE',  ( -1.000000000000000000, -0.000000000000000000, 0.000000000000000000 ) ) ;
#65377=CARTESIAN_POINT ( 'NONE',  ( -16.81410256410256565, -7.500000000000000000, 29.75000000000000355 ) ) ;
#65402=CARTESIAN_POINT ( 'NONE',  ( -19.50000000000000000, -3.499999999999999556, 29.75000000000000355 ) ) ;
#65410=VECTOR ( 'NONE', #71250, 1000.000000000000000 ) ;
#65420=EDGE_CURVE ( 'NONE', #8287, #26079, #39202, .T. ) ;
#65425=DIRECTION ( 'NONE',  ( -1.000000000000000000, -0.000000000000000000, 0.000000000000000000 ) ) ;
#65443=CARTESIAN_POINT ( 'NONE',  ( -19.50000000000000000, -11.50000000000000000, 29.75000000000000355 ) ) ;
#65454=EDGE_CURVE ( 'NONE', #32893, #13118, #17132, .T. ) ;
#65459=EDGE_CURVE ( 'NONE', #79307, #36536, #79292, .T. ) ;
#65461=ORIENTED_EDGE ( 'NONE', *, *, #39912, .F. ) ;
#65462=VECTOR ( 'NONE', #85552, 1000.000000000000000 ) ;
#65469=CARTESIAN_POINT ( 'NONE',  ( -16.09615384615384670, -3.499999999999999556, 29.75000000000000355 ) ) ;
#65503=CARTESIAN_POINT ( 'NONE',  ( -0.3589743589743593088, -7.500000000000000000, 29.75000000000000355 ) ) ;
#65508=LINE ( 'NONE', #86702, #5761 ) ;
#65515=VERTEX_POINT ( 'NONE', #16090 ) ;
#65536=ORIENTED_EDGE ( 'NONE', *, *, #80652, .F. ) ;
#65539=CARTESIAN_POINT ( 'NONE',  ( 20.00000000000000000, -4.000000000000000000, 29.75000000000000355 ) ) ;
#65540=CARTESIAN_POINT ( 'NONE',  ( 0.3589743589743582541, -11.00000000000000000, 29.75000000000000355 ) ) ;
#65543=ADVANCED_FACE ( 'NONE', ( #8457 ), #79123, .T. ) ;
#65555=EDGE_LOOP ( 'NONE', ( #27516, #76860, #40927, #12969, #69541 ) ) ;
#65565=ORIENTED_EDGE ( 'NONE', *, *, #25917, .F. ) ;
#65574=VECTOR ( 'NONE', #25067, 1000.000000000000000 ) ;
#65588=AXIS2_PLACEMENT_3D ( 'NONE', #57694, #14492, #85176 ) ;
#65605=ORIENTED_EDGE ( 'NONE', *, *, #43118, .T. ) ;
#65644=DIRECTION ( 'NONE',  ( -0.000000000000000000, 1.000000000000000000, -0.000000000000000000 ) ) ;
#65645=EDGE_CURVE ( 'NONE', #78266, #30104, #43556, .T. ) ;
#65663=PLANE ( 'NONE',  #53705 ) ;
#65671=AXIS2_PLACEMENT_3D ( 'NONE', #42962, #29889, #21794 ) ;
#65672=ORIENTED_EDGE ( 'NONE', *, *, #77434, .T. ) ;
#65677=EDGE_LOOP ( 'NONE', ( #26711, #60170, #79231, #24785, #77575 ) ) ;
#65678=VECTOR ( 'NONE', #11578, 1000.000000000000000 ) ;
#65689=PLANE ( 'NONE',  #60589 ) ;
#65697=DIRECTION ( 'NONE',  ( 1.000000000000000000, 0.000000000000000000, 0.000000000000000000 ) ) ;
#65700=ORIENTED_EDGE ( 'NONE', *, *, #42726, .F. ) ;
#65705=LINE ( 'NONE', #36593, #2966 ) ;
#65719=DIRECTION ( 'NONE',  ( -0.000000000000000000, 1.000000000000000000, -0.000000000000000000 ) ) ;
#65753=VERTEX_POINT ( 'NONE', #38132 ) ;
#65761=CARTESIAN_POINT ( 'NONE',  ( 18.03205128205128105, -11.50000000000000000, 29.75000000000000355 ) ) ;
#65770=CARTESIAN_POINT ( 'NONE',  ( 11.25641025641025550, -3.499999999999999556, 29.75000000000000355 ) ) ;
#65778=EDGE_CURVE ( 'NONE', #15288, #75095, #36447, .T. ) ;
#65780=AXIS2_PLACEMENT_3D ( 'NONE', #70626, #51656, #37271 ) ;
#65784=ORIENTED_EDGE ( 'NONE', *, *, #66192, .T. ) ;
#65786=ORIENTED_EDGE ( 'NONE', *, *, #24427, .F. ) ;
#65792=ORIENTED_EDGE ( 'NONE', *, *, #15133, .T. ) ;
#65810=ADVANCED_FACE ( 'NONE', ( #83913 ), #77139, .T. ) ;
#65813=FACE_OUTER_BOUND ( 'NONE', #82954, .T. ) ;
#65817=ORIENTED_EDGE ( 'NONE', *, *, #16779, .T. ) ;
#65825=PLANE ( 'NONE',  #62463 ) ;
#65837=DIRECTION ( 'NONE',  ( -1.000000000000000000, 0.000000000000000000, -0.000000000000000000 ) ) ;
#65845=CARTESIAN_POINT ( 'NONE',  ( 11.25641025641025550, -4.000000000000000000, 29.75000000000000355 ) ) ;
#65849=ORIENTED_EDGE ( 'NONE', *, *, #42568, .F. ) ;
#65856=CARTESIAN_POINT ( 'NONE',  ( -5.198717948717948012, -3.499999999999999556, 29.75000000000000355 ) ) ;
#65886=DIRECTION ( 'NONE',  ( -1.000000000000000000, -0.000000000000000000, -0.000000000000000000 ) ) ;
#65894=ORIENTED_EDGE ( 'NONE', *, *, #39153, .F. ) ;
#65905=DIRECTION ( 'NONE',  ( -1.000000000000000000, -0.000000000000000000, -0.000000000000000000 ) ) ;
#65919=ORIENTED_EDGE ( 'NONE', *, *, #43835, .T. ) ;
#65929=LINE ( 'NONE', #18657, #64831 ) ;
#65936=ADVANCED_FACE ( 'NONE', ( #62039 ), #82327, .T. ) ;
#65939=ORIENTED_EDGE ( 'NONE', *, *, #66537, .T. ) ;
#65956=DIRECTION ( 'NONE',  ( -1.000000000000000000, 0.000000000000000000, -0.000000000000000000 ) ) ;
#65981=DIRECTION ( 'NONE',  ( 0.000000000000000000, 0.000000000000000000, -1.000000000000000000 ) ) ;
#65989=ORIENTED_EDGE ( 'NONE', *, *, #41874, .T. ) ;
#65994=DIRECTION ( 'NONE',  ( -1.000000000000000000, -0.000000000000000000, -0.000000000000000000 ) ) ;
#65998=ORIENTED_EDGE ( 'NONE', *, *, #9062, .F. ) ;
#66000=ORIENTED_EDGE ( 'NONE', *, *, #42735, .F. ) ;
#66002=CARTESIAN_POINT ( 'NONE',  ( -15.12820512820512953, -11.00000000000000000, 29.75000000000000355 ) ) ;
#66003=CARTESIAN_POINT ( 'NONE',  ( 13.19230769230769340, -3.499999999999999556, 29.75000000000000355 ) ) ;
#66005=CARTESIAN_POINT ( 'NONE',  ( -14.87820512820512953, -7.500000000000000000, 29.75000000000000355 ) ) ;
#66020=ORIENTED_EDGE ( 'NONE', *, *, #17401, .F. ) ;
#66044=CARTESIAN_POINT ( 'NONE',  ( 0.000000000000000000, -11.00000000000000000, 29.75000000000000355 ) ) ;
#66054=VECTOR ( 'NONE', #70154, 1000.000000000000000 ) ;
#66070=AXIS2_PLACEMENT_3D ( 'NONE', #19247, #12488, #39971 ) ;
#66082=DIRECTION ( 'NONE',  ( 0.000000000000000000, 0.000000000000000000, -1.000000000000000000 ) ) ;
#66083=CARTESIAN_POINT ( 'NONE',  ( -11.97435897435897267, -11.00000000000000000, 29.75000000000000355 ) ) ;
#66085=ORIENTED_EDGE ( 'NONE', *, *, #76135, .T. ) ;
#66090=DIRECTION ( 'NONE',  ( -0.000000000000000000, 1.000000000000000000, -0.000000000000000000 ) ) ;
#66098=VERTEX_POINT ( 'NONE', #44860 ) ;
#66106=VECTOR ( 'NONE', #20730, 1000.000000000000000 ) ;
#66109=ORIENTED_EDGE ( 'NONE', *, *, #83072, .F. ) ;
#66118=VECTOR ( 'NONE', #58036, 1000.000000000000000 ) ;
#66122=EDGE_CURVE ( 'NONE', #46484, #26148, #71894, .T. ) ;
#66129=CARTESIAN_POINT ( 'NONE',  ( -10.03846153846153832, -11.00000000000000000, 29.25000000000000000 ) ) ;
#66133=LINE ( 'NONE', #86889, #12595 ) ;
#66142=DIRECTION ( 'NONE',  ( -0.000000000000000000, 1.000000000000000000, -0.000000000000000000 ) ) ;
#66145=ORIENTED_EDGE ( 'NONE', *, *, #65420, .T. ) ;
#66152=EDGE_LOOP ( 'NONE', ( #58381, #51276, #66000, #29150 ) ) ;
#66191=VECTOR ( 'NONE', #37109, 1000.000000000000000 ) ;
#66192=EDGE_CURVE ( 'NONE', #37853, #9873, #72235, .T. ) ;
#66216=ORIENTED_EDGE ( 'NONE', *, *, #21341, .T. ) ;
#66217=DIRECTION ( 'NONE',  ( 1.000000000000000000, 0.000000000000000000, 0.000000000000000000 ) ) ;
#66245=AXIS2_PLACEMENT_3D ( 'NONE', #64028, #8221, #37001 ) ;
#66262=PLANE ( 'NONE',  #5532 ) ;
#66271=ORIENTED_EDGE ( 'NONE', *, *, #70345, .T. ) ;
#66291=AXIS2_PLACEMENT_3D ( 'NONE', #59342, #80519, #18811 ) ;
#66300=CARTESIAN_POINT ( 'NONE',  ( -19.00000000000000000, -11.50000000000000000, 29.75000000000000355 ) ) ;
#66306=ORIENTED_EDGE ( 'NONE', *, *, #74615, .T. ) ;
#66309=CARTESIAN_POINT ( 'NONE',  ( 0.000000000000000000, -11.00000000000000000, 29.75000000000000355 ) ) ;
#66317=VECTOR ( 'NONE', #14470, 1000.000000000000000 ) ;
#66332=DIRECTION ( 'NONE',  ( -1.000000000000000000, -0.000000000000000000, -0.000000000000000000 ) ) ;
#66345=CYLINDRICAL_SURFACE ( 'NONE', #40184, 4.000000000000000000 ) ;
#66347=DIRECTION ( 'NONE',  ( 0.000000000000000000, 0.000000000000000000, 1.000000000000000000 ) ) ;
#66351=ORIENTED_EDGE ( 'NONE', *, *, #29295, .F. ) ;
#66382=CARTESIAN_POINT ( 'NONE',  ( 3.512820512820511443, -4.000000000000000000, 29.75000000000000355 ) ) ;
#66387=ORIENTED_EDGE ( 'NONE', *, *, #55699, .F. ) ;
#66391=ORIENTED_EDGE ( 'NONE', *, *, #33742, .F. ) ;
#66407=CARTESIAN_POINT ( 'NONE',  ( -11.97435897435897267, -11.50000000000000000, 29.75000000000000355 ) ) ;
#66414=EDGE_CURVE ( 'NONE', #13929, #14132, #77120, .T. ) ;
#66435=CARTESIAN_POINT ( 'NONE',  ( 5.448717948717947124, -3.499999999999999556, 29.75000000000000355 ) ) ;
#66436=ORIENTED_EDGE ( 'NONE', *, *, #67215, .T. ) ;
#66440=DIRECTION ( 'NONE',  ( -0.000000000000000000, 1.000000000000000000, -0.000000000000000000 ) ) ;
#66442=DIRECTION ( 'NONE',  ( -1.000000000000000000, -0.000000000000000000, 0.000000000000000000 ) ) ;
#66457=AXIS2_PLACEMENT_3D ( 'NONE', #62110, #417, #53577 ) ;
#66458=ORIENTED_EDGE ( 'NONE', *, *, #71272, .F. ) ;
#66461=VERTEX_POINT ( 'NONE', #76681 ) ;
#66464=CARTESIAN_POINT ( 'NONE',  ( 5.448717948717947124, -3.499999999999999556, 29.75000000000000355 ) ) ;
#66480=ADVANCED_FACE ( 'NONE', ( #30266 ), #31135, .T. ) ;
#66488=CARTESIAN_POINT ( 'NONE',  ( 15.12820512820512953, -7.500000000000000000, 29.75000000000000355 ) ) ;
#66518=VECTOR ( 'NONE', #83300, 1000.000000000000000 ) ;
#66519=DIRECTION ( 'NONE',  ( 1.000000000000000000, 0.000000000000000000, 0.000000000000000000 ) ) ;
#66522=DIRECTION ( 'NONE',  ( -1.000000000000000000, -0.000000000000000000, -0.000000000000000000 ) ) ;
#66537=EDGE_CURVE ( 'NONE', #43796, #28699, #4107, .T. ) ;
#66560=EDGE_CURVE ( 'NONE', #64311, #47437, #27904, .T. ) ;
#66576=AXIS2_PLACEMENT_3D ( 'NONE', #21408, #15543, #28614 ) ;
#66584=ORIENTED_EDGE ( 'NONE', *, *, #81321, .F. ) ;
#66610=AXIS2_PLACEMENT_3D ( 'NONE', #66435, #59670, #86731 ) ;
#66625=ORIENTED_EDGE ( 'NONE', *, *, #61937, .F. ) ;
#66635=CARTESIAN_POINT ( 'NONE',  ( -19.50000000000000000, -3.499999999999999556, 29.75000000000000355 ) ) ;
#66645=DIRECTION ( 'NONE',  ( 0.000000000000000000, 0.000000000000000000, -1.000000000000000000 ) ) ;
#66662=ORIENTED_EDGE ( 'NONE', *, *, #66560, .F. ) ;
#66664=VERTEX_POINT ( 'NONE', #75250 ) ;
#66665=LINE ( 'NONE', #10834, #35512 ) ;
#66666=ADVANCED_FACE ( 'NONE', ( #88344 ), #68052, .T. ) ;
#66675=VECTOR ( 'NONE', #13617, 1000.000000000000000 ) ;
#66680=EDGE_CURVE ( 'NONE', #86970, #20358, #53639, .T. ) ;
#66694=VECTOR ( 'NONE', #70460, 1000.000000000000000 ) ;
#66699=PLANE ( 'NONE',  #19791 ) ;
#66729=DIRECTION ( 'NONE',  ( 0.000000000000000000, 0.000000000000000000, 1.000000000000000000 ) ) ;
#66731=CARTESIAN_POINT ( 'NONE',  ( 9.320512820512821150, -1.926643599941765039, 29.65000000000000213 ) ) ;
#66740=CARTESIAN_POINT ( 'NONE',  ( 9.070512820512819374, -7.500000000000000000, 33.75000000000000000 ) ) ;
#66746=ORIENTED_EDGE ( 'NONE', *, *, #33748, .T. ) ;
#66762=VECTOR ( 'NONE', #63138, 1000.000000000000000 ) ;
#66765=ORIENTED_EDGE ( 'NONE', *, *, #21316, .F. ) ;
#66773=ORIENTED_EDGE ( 'NONE', *, *, #10586, .F. ) ;
#66783=DIRECTION ( 'NONE',  ( -1.000000000000000000, -0.000000000000000000, -0.000000000000000000 ) ) ;
#66786=DIRECTION ( 'NONE',  ( 1.000000000000000000, 0.000000000000000000, 0.000000000000000000 ) ) ;
#66789=CARTESIAN_POINT ( 'NONE',  ( -11.97435897435897267, -7.500000000000000000, 29.75000000000000355 ) ) ;
#66791=CARTESIAN_POINT ( 'NONE',  ( -7.134615384615385025, -11.00000000000000000, 29.75000000000000355 ) ) ;
#66808=DIRECTION ( 'NONE',  ( 1.000000000000000000, 0.000000000000000000, 0.000000000000000000 ) ) ;
#66819=DIRECTION ( 'NONE',  ( 0.000000000000000000, 0.000000000000000000, -1.000000000000000000 ) ) ;
#66823=ORIENTED_EDGE ( 'NONE', *, *, #88647, .T. ) ;
#66825=AXIS2_PLACEMENT_3D ( 'NONE', #43622, #50803, #71532 ) ;
#66832=LINE ( 'NONE', #3789, #44858 ) ;
#66836=CARTESIAN_POINT ( 'NONE',  ( 9.320512820512821150, -4.000000000000000000, 29.25000000000000000 ) ) ;
#66839=ORIENTED_EDGE ( 'NONE', *, *, #75843, .T. ) ;
#66841=CARTESIAN_POINT ( 'NONE',  ( -7.384615384615385025, -11.00000000000000000, 29.75000000000000355 ) ) ;
#66855=DIRECTION ( 'NONE',  ( -0.000000000000000000, 1.000000000000000000, -0.000000000000000000 ) ) ;
#66875=DIRECTION ( 'NONE',  ( -0.000000000000000000, 1.000000000000000000, -0.000000000000000000 ) ) ;
#66880=CARTESIAN_POINT ( 'NONE',  ( 0.000000000000000000, -11.00000000000000000, 29.75000000000000355 ) ) ;
#66890=AXIS2_PLACEMENT_3D ( 'NONE', #61275, #6787, #88792 ) ;
#66894=ORIENTED_EDGE ( 'NONE', *, *, #87731, .F. ) ;
#66897=CARTESIAN_POINT ( 'NONE',  ( -4.230769230769230838, -3.499999999999999556, 29.75000000000000355 ) ) ;
#66939=CARTESIAN_POINT ( 'NONE',  ( -18.75000000000000000, -3.499999999999999556, 29.75000000000000355 ) ) ;
#66946=DIRECTION ( 'NONE',  ( -1.000000000000000000, -0.000000000000000000, -0.000000000000000000 ) ) ;
#66961=ORIENTED_EDGE ( 'NONE', *, *, #70111, .F. ) ;
#66965=DIRECTION ( 'NONE',  ( -0.000000000000000000, 1.000000000000000000, -0.000000000000000000 ) ) ;
#66966=LINE ( 'NONE', #67849, #82685 ) ;
#66978=LINE ( 'NONE', #26436, #69874 ) ;
#66984=CARTESIAN_POINT ( 'NONE',  ( 5.448717948717947124, -7.500000000000000000, 29.75000000000000355 ) ) ;
#66988=CARTESIAN_POINT ( 'NONE',  ( 0.6089743589743582541, -7.500000000000000000, 33.75000000000000000 ) ) ;
#66990=ORIENTED_EDGE ( 'NONE', *, *, #68044, .T. ) ;
#66991=VECTOR ( 'NONE', #1495, 1000.000000000000000 ) ;
#66998=EDGE_CURVE ( 'NONE', #48416, #74021, #85544, .T. ) ;
#67022=EDGE_CURVE ( 'NONE', #72142, #32479, #82683, .T. ) ;
#67028=EDGE_LOOP ( 'NONE', ( #68062, #83202, #37474, #57065 ) ) ;
#67031=CARTESIAN_POINT ( 'NONE',  ( 0.000000000000000000, -11.00000000000000000, 29.75000000000000355 ) ) ;
#67044=CARTESIAN_POINT ( 'NONE',  ( 12.94230769230769340, -7.500000000000000000, 29.75000000000000355 ) ) ;
#67049=CARTESIAN_POINT ( 'NONE',  ( 12.22435897435897267, -3.499999999999999556, 29.75000000000000355 ) ) ;
#67064=CARTESIAN_POINT ( 'NONE',  ( -17.78205128205128105, -3.499999999999999556, 29.75000000000000355 ) ) ;
#67075=DIRECTION ( 'NONE',  ( 0.000000000000000000, 0.000000000000000000, -1.000000000000000000 ) ) ;
#67087=CARTESIAN_POINT ( 'NONE',  ( -0.6089743589743593644, -3.499999999999999556, 29.75000000000000355 ) ) ;
#67120=VECTOR ( 'NONE', #72963, 1000.000000000000000 ) ;
#67129=VERTEX_POINT ( 'NONE', #70930 ) ;
#67176=DIRECTION ( 'NONE',  ( -1.000000000000000000, -0.000000000000000000, -0.000000000000000000 ) ) ;
#67183=CIRCLE ( 'NONE', #74245, 4.000000000000000000 ) ;
#67204=CARTESIAN_POINT ( 'NONE',  ( 16.09615384615384670, -11.50000000000000000, 29.75000000000000355 ) ) ;
#67205=ORIENTED_EDGE ( 'NONE', *, *, #2680, .T. ) ;
#67210=DIRECTION ( 'NONE',  ( -1.000000000000000000, 0.000000000000000000, -0.000000000000000000 ) ) ;
#67215=EDGE_CURVE ( 'NONE', #82495, #76951, #9665, .T. ) ;
#67223=PLANE ( 'NONE',  #8357 ) ;
#67224=FILL_AREA_STYLE_COLOUR ( '', #44640 ) ;
#67241=VECTOR ( 'NONE', #40794, 1000.000000000000000 ) ;
#67246=EDGE_LOOP ( 'NONE', ( #77077, #74340, #8312, #19072 ) ) ;
#67248=ORIENTED_EDGE ( 'NONE', *, *, #4526, .F. ) ;
#67257=ORIENTED_EDGE ( 'NONE', *, *, #44833, .F. ) ;
#67260=ORIENTED_EDGE ( 'NONE', *, *, #72534, .T. ) ;
#67265=EDGE_CURVE ( 'NONE', #9623, #83736, #30820, .T. ) ;
#67274=ORIENTED_EDGE ( 'NONE', *, *, #45903, .T. ) ;
#67294=LINE ( 'NONE', #7367, #54074 ) ;
#67305=ORIENTED_EDGE ( 'NONE', *, *, #2890, .T. ) ;
#67311=CARTESIAN_POINT ( 'NONE',  ( -19.50000000000000000, -11.50000000000000000, 29.75000000000000355 ) ) ;
#67339=ORIENTED_EDGE ( 'NONE', *, *, #71393, .F. ) ;
#67347=CARTESIAN_POINT ( 'NONE',  ( 19.50000000000000000, -11.00000000000000000, 29.25000000000000000 ) ) ;
#67394=CARTESIAN_POINT ( 'NONE',  ( 14.87820512820512953, -7.500000000000000000, 29.75000000000000355 ) ) ;
#67399=ORIENTED_EDGE ( 'NONE', *, *, #33015, .F. ) ;
#67413=LINE ( 'NONE', #82265, #56139 ) ;
#67415=CARTESIAN_POINT ( 'NONE',  ( -19.50000000000000000, -3.499999999999999556, 29.75000000000000355 ) ) ;
#67446=VERTEX_POINT ( 'NONE', #9560 ) ;
#67452=EDGE_CURVE ( 'NONE', #33780, #16151, #42478, .T. ) ;
#67467=EDGE_CURVE ( 'NONE', #45953, #35283, #21750, .T. ) ;
#67479=DIRECTION ( 'NONE',  ( 1.000000000000000000, 0.000000000000000000, 0.000000000000000000 ) ) ;
#67496=ORIENTED_EDGE ( 'NONE', *, *, #33799, .T. ) ;
#67499=VECTOR ( 'NONE', #79652, 1000.000000000000000 ) ;
#67508=CARTESIAN_POINT ( 'NONE',  ( -19.50000000000000000, -11.50000000000000000, 29.75000000000000355 ) ) ;
#67527=CARTESIAN_POINT ( 'NONE',  ( 15.84615384615384670, -4.000000000000000000, 29.75000000000000355 ) ) ;
#67549=ADVANCED_FACE ( 'NONE', ( #72145 ), #65825, .T. ) ;
#67574=CARTESIAN_POINT ( 'NONE',  ( -14.87820512820512953, -7.500000000000000000, 29.75000000000000355 ) ) ;
#67595=DIRECTION ( 'NONE',  ( 1.000000000000000000, 0.000000000000000000, 0.000000000000000000 ) ) ;
#67596=CARTESIAN_POINT ( 'NONE',  ( -18.75000000000000000, -7.500000000000000000, 29.75000000000000355 ) ) ;
#67597=CYLINDRICAL_SURFACE ( 'NONE', #57703, 4.000000000000000000 ) ;
#67606=EDGE_CURVE ( 'NONE', #12551, #6115, #88803, .T. ) ;
#67608=CARTESIAN_POINT ( 'NONE',  ( 8.352564102564102200, -3.499999999999999556, 29.75000000000000355 ) ) ;
#67610=ORIENTED_EDGE ( 'NONE', *, *, #70971, .F. ) ;
#67618=VERTEX_POINT ( 'NONE', #41038 ) ;
#67619=VECTOR ( 'NONE', #58040, 1000.000000000000000 ) ;
#67644=PLANE ( 'NONE',  #27366 ) ;
#67652=DIRECTION ( 'NONE',  ( -0.000000000000000000, 1.000000000000000000, -0.000000000000000000 ) ) ;
#67663=ORIENTED_EDGE ( 'NONE', *, *, #21877, .T. ) ;
#67680=EDGE_CURVE ( 'NONE', #47848, #11498, #62185, .T. ) ;
#67691=CARTESIAN_POINT ( 'NONE',  ( -7.134615384615385025, -3.499999999999999556, 29.75000000000000355 ) ) ;
#67696=FACE_OUTER_BOUND ( 'NONE', #8144, .T. ) ;
#67697=CARTESIAN_POINT ( 'NONE',  ( 20.00000000000000000, -4.000000000000000000, 29.75000000000000355 ) ) ;
#67700=ORIENTED_EDGE ( 'NONE', *, *, #2608, .F. ) ;
#67712=PLANE ( 'NONE',  #34674 ) ;
#67714=CIRCLE ( 'NONE', #51875, 4.000000000000000000 ) ;
#67723=CARTESIAN_POINT ( 'NONE',  ( -19.50000000000000000, -11.50000000000000000, 29.75000000000000355 ) ) ;
#67750=ORIENTED_EDGE ( 'NONE', *, *, #25064, .F. ) ;
#67761=DIRECTION ( 'NONE',  ( 0.000000000000000000, 0.000000000000000000, -1.000000000000000000 ) ) ;
#67764=CARTESIAN_POINT ( 'NONE',  ( -11.97435897435897267, -11.50000000000000000, 29.75000000000000355 ) ) ;
#67777=DIRECTION ( 'NONE',  ( -1.000000000000000000, -0.000000000000000000, -0.000000000000000000 ) ) ;
#67779=DIRECTION ( 'NONE',  ( 0.000000000000000000, 0.000000000000000000, -1.000000000000000000 ) ) ;
#67780=ORIENTED_EDGE ( 'NONE', *, *, #53942, .F. ) ;
#67781=AXIS2_PLACEMENT_3D ( 'NONE', #12361, #5155, #4717 ) ;
#67795=EDGE_CURVE ( 'NONE', #73790, #30150, #43682, .T. ) ;
#67799=FACE_OUTER_BOUND ( 'NONE', #8411, .T. ) ;
#67812=EDGE_CURVE ( 'NONE', #26079, #85537, #55429, .T. ) ;
#67815=CARTESIAN_POINT ( 'NONE',  ( -4.480769230769230838, -7.500000000000000000, 29.75000000000000355 ) ) ;
#67816=EDGE_LOOP ( 'NONE', ( #66387, #26571, #28124, #21706 ) ) ;
#67827=VECTOR ( 'NONE', #7231, 1000.000000000000000 ) ;
#67830=CARTESIAN_POINT ( 'NONE',  ( 7.384615384615385025, -4.000000000000000000, 29.75000000000000355 ) ) ;
#67834=FACE_OUTER_BOUND ( 'NONE', #57507, .T. ) ;
#67837=LINE ( 'NONE', #5687, #19913 ) ;
#67848=CARTESIAN_POINT ( 'NONE',  ( -7.384615384615385025, -7.500000000000000000, 29.75000000000000355 ) ) ;
#67849=CARTESIAN_POINT ( 'NONE',  ( -6.166666666666667851, -11.50000000000000000, 29.75000000000000355 ) ) ;
#67861=EDGE_CURVE ( 'NONE', #34265, #3876, #9027, .T. ) ;
#67866=DIRECTION ( 'NONE',  ( -1.000000000000000000, 0.000000000000000000, -0.000000000000000000 ) ) ;
#67871=ORIENTED_EDGE ( 'NONE', *, *, #14850, .T. ) ;
#67872=CARTESIAN_POINT ( 'NONE',  ( -5.448717948717948012, -3.499999999999999556, 29.75000000000000355 ) ) ;
#67873=CARTESIAN_POINT ( 'NONE',  ( 20.00000000000000000, -11.00000000000000000, 28.25000000000000000 ) ) ;
#67887=ORIENTED_EDGE ( 'NONE', *, *, #62319, .T. ) ;
#67896=FACE_OUTER_BOUND ( 'NONE', #31994, .T. ) ;
#67909=DIRECTION ( 'NONE',  ( 0.000000000000000000, 0.000000000000000000, -1.000000000000000000 ) ) ;
#67912=ORIENTED_EDGE ( 'NONE', *, *, #26803, .F. ) ;
#67922=CARTESIAN_POINT ( 'NONE',  ( 20.00000000000000000, -4.000000000000000000, 29.75000000000000355 ) ) ;
#67924=CARTESIAN_POINT ( 'NONE',  ( 20.00000000000000000, -4.000000000000000000, 29.75000000000000355 ) ) ;
#67929=AXIS2_PLACEMENT_3D ( 'NONE', #80591, #37804, #58501 ) ;
#67942=AXIS2_PLACEMENT_3D ( 'NONE', #29456, #86624, #71745 ) ;
#67943=CARTESIAN_POINT ( 'NONE',  ( 11.97435897435897267, -7.500000000000000000, 33.75000000000000000 ) ) ;
#67952=LINE ( 'NONE', #67064, #77619 ) ;
#67982=CARTESIAN_POINT ( 'NONE',  ( -9.320512820512821150, -1.926643599941765039, 29.65000000000000213 ) ) ;
#67995=EDGE_CURVE ( 'NONE', #19429, #21320, #46798, .T. ) ;
#67997=ORIENTED_EDGE ( 'NONE', *, *, #71965, .T. ) ;
#68001=ORIENTED_EDGE ( 'NONE', *, *, #10052, .F. ) ;
#68014=AXIS2_PLACEMENT_3D ( 'NONE', #38994, #11513, #87187 ) ;
#68024=ORIENTED_EDGE ( 'NONE', *, *, #17276, .T. ) ;
#68027=EDGE_LOOP ( 'NONE', ( #30795, #88273, #40793, #65320, #65786 ) ) ;
#68043=DIRECTION ( 'NONE',  ( -1.000000000000000000, -0.000000000000000000, -0.000000000000000000 ) ) ;
#68044=EDGE_CURVE ( 'NONE', #3756, #7644, #51015, .T. ) ;
#68046=ORIENTED_EDGE ( 'NONE', *, *, #20111, .T. ) ;
#68052=CYLINDRICAL_SURFACE ( 'NONE', #81090, 4.000000000000000000 ) ;
#68055=ORIENTED_EDGE ( 'NONE', *, *, #45490, .F. ) ;
#68062=ORIENTED_EDGE ( 'NONE', *, *, #87924, .F. ) ;
#68065=AXIS2_PLACEMENT_3D ( 'NONE', #74673, #60700, #67909 ) ;
#68067=ADVANCED_FACE ( 'NONE', ( #7589 ), #62510, .F. ) ;
#68099=VECTOR ( 'NONE', #59137, 1000.000000000000000 ) ;
#68106=ORIENTED_EDGE ( 'NONE', *, *, #62417, .T. ) ;
#68110=DIRECTION ( 'NONE',  ( -0.000000000000000000, 1.000000000000000000, -0.000000000000000000 ) ) ;
#68118=CARTESIAN_POINT ( 'NONE',  ( 16.09615384615384670, -3.499999999999999556, 29.75000000000000355 ) ) ;
#68132=ORIENTED_EDGE ( 'NONE', *, *, #67795, .F. ) ;
#68133=ORIENTED_EDGE ( 'NONE', *, *, #51536, .F. ) ;
#68158=LINE ( 'NONE', #46552, #45694 ) ;
#68161=LINE ( 'NONE', #83907, #59110 ) ;
#68164=DIRECTION ( 'NONE',  ( 0.000000000000000000, 0.000000000000000000, -1.000000000000000000 ) ) ;
#68207=CARTESIAN_POINT ( 'NONE',  ( 16.09615384615384670, -3.499999999999999556, 29.75000000000000355 ) ) ;
#68216=CARTESIAN_POINT ( 'NONE',  ( -19.50000000000000000, -11.50000000000000000, 29.75000000000000355 ) ) ;
#68218=DIRECTION ( 'NONE',  ( 0.000000000000000000, 0.000000000000000000, -1.000000000000000000 ) ) ;
#68229=EDGE_CURVE ( 'NONE', #54682, #75345, #60638, .T. ) ;
#68243=AXIS2_PLACEMENT_3D ( 'NONE', #53857, #5228, #87221 ) ;
#68247=ORIENTED_EDGE ( 'NONE', *, *, #71305, .T. ) ;
#68252=CARTESIAN_POINT ( 'NONE',  ( 18.03205128205128105, -7.500000000000000000, 29.75000000000000355 ) ) ;
#68289=LINE ( 'NONE', #34504, #26879 ) ;
#68292=ORIENTED_EDGE ( 'NONE', *, *, #37549, .T. ) ;
#68307=ORIENTED_EDGE ( 'NONE', *, *, #47127, .F. ) ;
#68330=EDGE_CURVE ( 'NONE', #84875, #72142, #66966, .T. ) ;
#68333=ADVANCED_FACE ( 'NONE', ( #5261 ), #32293, .F. ) ;
#68335=DIRECTION ( 'NONE',  ( 0.000000000000000000, 0.000000000000000000, 1.000000000000000000 ) ) ;
#68348=DIRECTION ( 'NONE',  ( -1.000000000000000000, -0.000000000000000000, 0.000000000000000000 ) ) ;
#68357=VERTEX_POINT ( 'NONE', #74165 ) ;
#68370=DIRECTION ( 'NONE',  ( 0.000000000000000000, 0.000000000000000000, -1.000000000000000000 ) ) ;
#68399=DIRECTION ( 'NONE',  ( 1.000000000000000000, 0.000000000000000000, 0.000000000000000000 ) ) ;
#68404=CARTESIAN_POINT ( 'NONE',  ( 0.000000000000000000, -11.00000000000000000, 29.75000000000000355 ) ) ;
#68405=DIRECTION ( 'NONE',  ( 1.000000000000000000, 0.000000000000000000, 0.000000000000000000 ) ) ;
#68415=EDGE_CURVE ( 'NONE', #34333, #23619, #37042, .T. ) ;
#68420=EDGE_LOOP ( 'NONE', ( #65565, #80181, #43725, #12168 ) ) ;
#68425=PLANE ( 'NONE',  #15519 ) ;
#68427=CARTESIAN_POINT ( 'NONE',  ( 1.576923076923076428, -11.50000000000000000, 29.75000000000000355 ) ) ;
#68461=EDGE_CURVE ( 'NONE', #87211, #68522, #43808, .T. ) ;
#68469=CARTESIAN_POINT ( 'NONE',  ( -3.262820512820514107, -7.500000000000000000, 33.75000000000000000 ) ) ;
#68471=DIRECTION ( 'NONE',  ( 1.000000000000000000, 0.000000000000000000, 0.000000000000000000 ) ) ;
#68474=ADVANCED_FACE ( 'NONE', ( #57768 ), #42939, .F. ) ;
#68484=VECTOR ( 'NONE', #78914, 1000.000000000000000 ) ;
#68488=PLANE ( 'NONE',  #66890 ) ;
#68504=DIRECTION ( 'NONE',  ( -1.000000000000000000, -0.000000000000000000, -0.000000000000000000 ) ) ;
#68506=ORIENTED_EDGE ( 'NONE', *, *, #10052, .T. ) ;
#68520=AXIS2_PLACEMENT_3D ( 'NONE', #34192, #53124, #25221 ) ;
#68522=VERTEX_POINT ( 'NONE', #65845 ) ;
#68527=LINE ( 'NONE', #32522, #11154 ) ;
#68538=EDGE_CURVE ( 'NONE', #47848, #78478, #46032, .T. ) ;
#68558=CIRCLE ( 'NONE', #36919, 4.000000000000000000 ) ;
#68567=CARTESIAN_POINT ( 'NONE',  ( 8.102564102564102200, -7.500000000000000000, 33.75000000000000000 ) ) ;
#68572=PLANE ( 'NONE',  #81620 ) ;
#68605=CARTESIAN_POINT ( 'NONE',  ( 20.00000000000000000, -7.500000000000000000, 33.75000000000000000 ) ) ;
#68614=ORIENTED_EDGE ( 'NONE', *, *, #46501, .F. ) ;
#68616=LINE ( 'NONE', #6911, #35552 ) ;
#68623=CARTESIAN_POINT ( 'NONE',  ( 2.544871794871792936, -3.499999999999999556, 29.75000000000000355 ) ) ;
#68626=AXIS2_PLACEMENT_3D ( 'NONE', #34875, #56036, #20036 ) ;
#68627=FACE_OUTER_BOUND ( 'NONE', #9463, .T. ) ;
#68654=ADVANCED_FACE ( 'NONE', ( #65238 ), #1774, .T. ) ;
#68658=LINE ( 'NONE', #6958, #30755 ) ;
#68668=CARTESIAN_POINT ( 'NONE',  ( 3.512820512820510555, -7.500000000000000000, 29.75000000000000355 ) ) ;
#68678=DIRECTION ( 'NONE',  ( -1.000000000000000000, -0.000000000000000000, -0.000000000000000000 ) ) ;
#68687=ADVANCED_FACE ( 'NONE', ( #44513 ), #70236, .T. ) ;
#68709=CIRCLE ( 'NONE', #28468, 4.000000000000000000 ) ;
#68714=EDGE_CURVE ( 'NONE', #44505, #58148, #59822, .T. ) ;
#68716=EDGE_CURVE ( 'NONE', #40595, #21236, #79655, .T. ) ;
#68727=VERTEX_POINT ( 'NONE', #74233 ) ;
#68740=CARTESIAN_POINT ( 'NONE',  ( -9.320512820512821150, -7.500000000000000000, 29.75000000000000355 ) ) ;
#68745=AXIS2_PLACEMENT_3D ( 'NONE', #28615, #22295, #83572 ) ;
#68777=ADVANCED_FACE ( 'NONE', ( #5330 ), #59379, .T. ) ;
#68782=VECTOR ( 'NONE', #972, 1000.000000000000000 ) ;
#68784=DIRECTION ( 'NONE',  ( -1.000000000000000000, -0.000000000000000000, -0.000000000000000000 ) ) ;
#68789=EDGE_CURVE ( 'NONE', #18370, #81105, #64008, .T. ) ;
#68793=ORIENTED_EDGE ( 'NONE', *, *, #25591, .F. ) ;
#68795=CARTESIAN_POINT ( 'NONE',  ( -11.00641025641025550, -3.499999999999999556, 29.75000000000000355 ) ) ;
#68801=EDGE_CURVE ( 'NONE', #51776, #85035, #19288, .T. ) ;
#68804=VECTOR ( 'NONE', #72130, 1000.000000000000000 ) ;
#68813=LINE ( 'NONE', #77340, #73602 ) ;
#68814=EDGE_LOOP ( 'NONE', ( #26460, #70030, #29151, #35724 ) ) ;
#68818=DIRECTION ( 'NONE',  ( -1.000000000000000000, -0.000000000000000000, -0.000000000000000000 ) ) ;
#68820=ORIENTED_EDGE ( 'NONE', *, *, #29613, .F. ) ;
#68826=CARTESIAN_POINT ( 'NONE',  ( 8.102564102564102200, -11.50000000000000000, 29.75000000000000355 ) ) ;
#68843=PLANE ( 'NONE',  #31651 ) ;
#68846=DIRECTION ( 'NONE',  ( 1.000000000000000000, 0.000000000000000000, 0.000000000000000000 ) ) ;
#68855=DIRECTION ( 'NONE',  ( 0.000000000000000000, 0.000000000000000000, -1.000000000000000000 ) ) ;
#68884=ORIENTED_EDGE ( 'NONE', *, *, #45812, .T. ) ;
#68890=AXIS2_PLACEMENT_3D ( 'NONE', #51466, #18611, #73561 ) ;
#68900=VECTOR ( 'NONE', #33184, 1000.000000000000000 ) ;
#68919=PLANE ( 'NONE',  #53413 ) ;
#68927=CARTESIAN_POINT ( 'NONE',  ( -19.50000000000000000, -3.499999999999999556, 29.75000000000000355 ) ) ;
#68929=ADVANCED_FACE ( 'NONE', ( #85679 ), #71704, .F. ) ;
#68952=DIRECTION ( 'NONE',  ( 0.000000000000000000, 0.000000000000000000, -1.000000000000000000 ) ) ;
#68953=DIRECTION ( 'NONE',  ( 1.000000000000000000, 0.000000000000000000, 0.000000000000000000 ) ) ;
#68957=DIRECTION ( 'NONE',  ( 0.000000000000000000, 0.000000000000000000, -1.000000000000000000 ) ) ;
#68965=AXIS2_PLACEMENT_3D ( 'NONE', #29144, #77310, #9737 ) ;
#68971=AXIS2_PLACEMENT_3D ( 'NONE', #44067, #63467, #50388 ) ;
#68972=CARTESIAN_POINT ( 'NONE',  ( -9.070512820512819374, -3.499999999999999556, 29.75000000000000355 ) ) ;
#68974=LINE ( 'NONE', #41508, #76738 ) ;
#68981=LINE ( 'NONE', #47376, #61404 ) ;
#68983=CARTESIAN_POINT ( 'NONE',  ( -19.50000000000000000, -3.499999999999999556, 29.75000000000000355 ) ) ;
#68989=ADVANCED_FACE ( 'NONE', ( #77591 ), #43360, .T. ) ;
#68996=CARTESIAN_POINT ( 'NONE',  ( -15.84615384615384670, -3.499999999999999556, 29.75000000000000355 ) ) ;
#68997=CIRCLE ( 'NONE', #53167, 4.000000000000000000 ) ;
#68998=ADVANCED_FACE ( 'NONE', ( #80716 ), #46018, .T. ) ;
#69015=CIRCLE ( 'NONE', #34501, 4.000000000000000000 ) ;
#69026=VECTOR ( 'NONE', #65365, 1000.000000000000000 ) ;
#69039=CARTESIAN_POINT ( 'NONE',  ( -13.19230769230769162, -7.500000000000000000, 29.75000000000000355 ) ) ;
#69046=DIRECTION ( 'NONE',  ( -0.000000000000000000, 1.000000000000000000, -0.000000000000000000 ) ) ;
#69056=EDGE_LOOP ( 'NONE', ( #30693, #51423, #81647, #42319 ) ) ;
#69059=CARTESIAN_POINT ( 'NONE',  ( -6.416666666666667851, -11.50000000000000000, 29.75000000000000355 ) ) ;
#69075=ADVANCED_FACE ( 'NONE', ( #498 ), #27525, .F. ) ;
#69090=CIRCLE ( 'NONE', #58982, 4.000000000000000000 ) ;
#69095=VECTOR ( 'NONE', #41557, 1000.000000000000000 ) ;
#69101=DIRECTION ( 'NONE',  ( 0.000000000000000000, 0.000000000000000000, -1.000000000000000000 ) ) ;
#69103=CARTESIAN_POINT ( 'NONE',  ( -10.03846153846153832, -4.000000000000000000, 29.65000000000000213 ) ) ;
#69112=PLANE ( 'NONE',  #68626 ) ;
#69117=ORIENTED_EDGE ( 'NONE', *, *, #85614, .F. ) ;
#69118=VERTEX_POINT ( 'NONE', #20329 ) ;
#69133=LINE ( 'NONE', #70467, #71782 ) ;
#69148=AXIS2_PLACEMENT_3D ( 'NONE', #34374, #77142, #598 ) ;
#69155=DIRECTION ( 'NONE',  ( -0.000000000000000000, 1.000000000000000000, -0.000000000000000000 ) ) ;
#69161=FACE_OUTER_BOUND ( 'NONE', #57015, .T. ) ;
#69197=CARTESIAN_POINT ( 'NONE',  ( -17.06410256410256565, -7.500000000000000000, 29.75000000000000355 ) ) ;
#69216=DIRECTION ( 'NONE',  ( -0.000000000000000000, 1.000000000000000000, -0.000000000000000000 ) ) ;
#69227=ORIENTED_EDGE ( 'NONE', *, *, #2360, .F. ) ;
#69228=ORIENTED_EDGE ( 'NONE', *, *, #53955, .F. ) ;
#69243=CARTESIAN_POINT ( 'NONE',  ( -2.294871794871793824, -11.50000000000000000, 29.75000000000000355 ) ) ;
#69258=CARTESIAN_POINT ( 'NONE',  ( 0.000000000000000000, -11.00000000000000000, 29.75000000000000355 ) ) ;
#69270=DIRECTION ( 'NONE',  ( 0.000000000000000000, 0.000000000000000000, -1.000000000000000000 ) ) ;
#69275=VECTOR ( 'NONE', #5504, 1000.000000000000000 ) ;
#69276=PLANE ( 'NONE',  #61144 ) ;
#69278=DIRECTION ( 'NONE',  ( -1.000000000000000000, -0.000000000000000000, -0.000000000000000000 ) ) ;
#69305=ORIENTED_EDGE ( 'NONE', *, *, #53942, .T. ) ;
#69311=CARTESIAN_POINT ( 'NONE',  ( -16.09615384615384670, -7.500000000000000000, 33.75000000000000000 ) ) ;
#69321=DIRECTION ( 'NONE',  ( 1.000000000000000000, 0.000000000000000000, 0.000000000000000000 ) ) ;
#69327=CARTESIAN_POINT ( 'NONE',  ( 10.03846153846153832, -3.499999999999999556, 29.75000000000000355 ) ) ;
#69334=CARTESIAN_POINT ( 'NONE',  ( 8.352564102564102200, -7.500000000000000000, 29.75000000000000355 ) ) ;
#69351=CARTESIAN_POINT ( 'NONE',  ( -13.91025641025641058, -11.00000000000000000, 29.75000000000000355 ) ) ;
#69355=CIRCLE ( 'NONE', #30511, 4.000000000000000000 ) ;
#69364=LINE ( 'NONE', #27487, #22600 ) ;
#69365=DIRECTION ( 'NONE',  ( -1.000000000000000000, -0.000000000000000000, -0.000000000000000000 ) ) ;
#69366=CARTESIAN_POINT ( 'NONE',  ( 0.000000000000000000, -11.00000000000000000, 29.75000000000000355 ) ) ;
#69385=CARTESIAN_POINT ( 'NONE',  ( 6.166666666666664298, -4.000000000000000000, 29.75000000000000355 ) ) ;
#69413=DIRECTION ( 'NONE',  ( -1.000000000000000000, -0.000000000000000000, -0.000000000000000000 ) ) ;
#69414=ADVANCED_FACE ( 'NONE', ( #73391 ), #11698, .F. ) ;
#69423=ORIENTED_EDGE ( 'NONE', *, *, #58025, .F. ) ;
#69431=DIRECTION ( 'NONE',  ( 1.000000000000000000, 0.000000000000000000, 0.000000000000000000 ) ) ;
#69433=EDGE_LOOP ( 'NONE', ( #1747, #67257, #50783, #42480 ) ) ;
#69448=EDGE_CURVE ( 'NONE', #9433, #13174, #21544, .T. ) ;
#69452=ORIENTED_EDGE ( 'NONE', *, *, #6860, .T. ) ;
#69455=CARTESIAN_POINT ( 'NONE',  ( 2.544871794871792936, -3.499999999999999556, 29.75000000000000355 ) ) ;
#69457=CARTESIAN_POINT ( 'NONE',  ( -5.198717948717948012, -3.499999999999999556, 29.75000000000000355 ) ) ;
#69462=VECTOR ( 'NONE', #53389, 1000.000000000000000 ) ;
#69482=ORIENTED_EDGE ( 'NONE', *, *, #86809, .T. ) ;
#69486=CARTESIAN_POINT ( 'NONE',  ( 3.512820512820510555, -7.500000000000000000, 33.75000000000000000 ) ) ;
#69496=EDGE_CURVE ( 'NONE', #78547, #42406, #13901, .T. ) ;
#69497=LINE ( 'NONE', #1490, #2827 ) ;
#69525=PLANE ( 'NONE',  #9727 ) ;
#69539=CARTESIAN_POINT ( 'NONE',  ( 20.00000000000000000, -4.000000000000000000, 29.75000000000000355 ) ) ;
#69541=ORIENTED_EDGE ( 'NONE', *, *, #79306, .T. ) ;
#69542=DIRECTION ( 'NONE',  ( 1.000000000000000000, 0.000000000000000000, 0.000000000000000000 ) ) ;
#69546=ORIENTED_EDGE ( 'NONE', *, *, #64548, .F. ) ;
#69551=DIRECTION ( 'NONE',  ( -0.000000000000000000, 1.000000000000000000, -0.000000000000000000 ) ) ;
#69552=EDGE_CURVE ( 'NONE', #18312, #64241, #55328, .T. ) ;
#69565=CARTESIAN_POINT ( 'NONE',  ( -17.06410256410256565, -3.499999999999999556, 29.75000000000000355 ) ) ;
#69568=ORIENTED_EDGE ( 'NONE', *, *, #37683, .F. ) ;
#69573=DIRECTION ( 'NONE',  ( -1.000000000000000000, -0.000000000000000000, -0.000000000000000000 ) ) ;
#69576=ADVANCED_FACE ( 'NONE', ( #56661 ), #83711, .F. ) ;
#69578=ORIENTED_EDGE ( 'NONE', *, *, #14074, .F. ) ;
#69582=VECTOR ( 'NONE', #66332, 1000.000000000000000 ) ;
#69586=EDGE_CURVE ( 'NONE', #61963, #12929, #63412, .T. ) ;
#69617=EDGE_LOOP ( 'NONE', ( #14924, #1406, #14373, #37972, #36488 ) ) ;
#69618=CARTESIAN_POINT ( 'NONE',  ( -19.50000000000000000, -3.499999999999999556, 29.75000000000000355 ) ) ;
#69624=VECTOR ( 'NONE', #44296, 1000.000000000000000 ) ;
#69642=LINE ( 'NONE', #22346, #10399 ) ;
#69646=VECTOR ( 'NONE', #50069, 1000.000000000000000 ) ;
#69647=EDGE_CURVE ( 'NONE', #67129, #21924, #8486, .T. ) ;
#69662=ORIENTED_EDGE ( 'NONE', *, *, #69552, .T. ) ;
#69665=CARTESIAN_POINT ( 'NONE',  ( 0.000000000000000000, -11.00000000000000000, 29.75000000000000355 ) ) ;
#69672=DIRECTION ( 'NONE',  ( -0.000000000000000000, 1.000000000000000000, -0.000000000000000000 ) ) ;
#69686=CARTESIAN_POINT ( 'NONE',  ( 14.16025641025641235, -3.499999999999999556, 29.75000000000000355 ) ) ;
#69730=DIRECTION ( 'NONE',  ( 0.000000000000000000, 0.000000000000000000, -1.000000000000000000 ) ) ;
#69736=LINE ( 'NONE', #68404, #882 ) ;
#69749=ORIENTED_EDGE ( 'NONE', *, *, #73675, .T. ) ;
#69752=ORIENTED_EDGE ( 'NONE', *, *, #69946, .T. ) ;
#69756=ORIENTED_EDGE ( 'NONE', *, *, #86362, .F. ) ;
#69777=ORIENTED_EDGE ( 'NONE', *, *, #33763, .T. ) ;
#69792=ORIENTED_EDGE ( 'NONE', *, *, #71393, .T. ) ;
#69803=ORIENTED_EDGE ( 'NONE', *, *, #72074, .F. ) ;
#69822=DIRECTION ( 'NONE',  ( -1.000000000000000000, -0.000000000000000000, -0.000000000000000000 ) ) ;
#69823=ORIENTED_EDGE ( 'NONE', *, *, #59881, .T. ) ;
#69842=DIRECTION ( 'NONE',  ( -0.000000000000000000, 1.000000000000000000, -0.000000000000000000 ) ) ;
#69845=EDGE_CURVE ( 'NONE', #35739, #88674, #7932, .T. ) ;
#69850=FACE_OUTER_BOUND ( 'NONE', #67028, .T. ) ;
#69874=VECTOR ( 'NONE', #86376, 1000.000000000000000 ) ;
#69891=ORIENTED_EDGE ( 'NONE', *, *, #55789, .F. ) ;
#69908=VECTOR ( 'NONE', #49858, 1000.000000000000000 ) ;
#69909=VERTEX_POINT ( 'NONE', #63312 ) ;
#69946=EDGE_CURVE ( 'NONE', #17400, #78293, #29106, .T. ) ;
#69989=LINE ( 'NONE', #26796, #78715 ) ;
#70012=CARTESIAN_POINT ( 'NONE',  ( 15.12820512820512953, -4.000000000000000000, 29.75000000000000355 ) ) ;
#70014=LINE ( 'NONE', #87776, #50366 ) ;
#70017=AXIS2_PLACEMENT_3D ( 'NONE', #3497, #71510, #30095 ) ;
#70030=ORIENTED_EDGE ( 'NONE', *, *, #59168, .F. ) ;
#70040=CARTESIAN_POINT ( 'NONE',  ( -17.78205128205128105, -7.500000000000000000, 29.75000000000000355 ) ) ;
#70042=FACE_OUTER_BOUND ( 'NONE', #50795, .T. ) ;
#70049=CARTESIAN_POINT ( 'NONE',  ( 19.00000000000000000, -7.500000000000000000, 29.75000000000000355 ) ) ;
#70059=EDGE_LOOP ( 'NONE', ( #29091, #47399, #80815, #53828, #14818 ) ) ;
#70066=CARTESIAN_POINT ( 'NONE',  ( 6.166666666666664298, -11.00000000000000000, 29.75000000000000355 ) ) ;
#70075=CARTESIAN_POINT ( 'NONE',  ( -11.97435897435897267, -7.500000000000000000, 29.75000000000000355 ) ) ;
#70086=DIRECTION ( 'NONE',  ( 0.000000000000000000, 0.000000000000000000, -1.000000000000000000 ) ) ;
#70103=CARTESIAN_POINT ( 'NONE',  ( -9.320512820512821150, -4.000000000000000000, 28.25000000000000000 ) ) ;
#70111=EDGE_CURVE ( 'NONE', #4346, #42531, #30853, .T. ) ;
#70115=ORIENTED_EDGE ( 'NONE', *, *, #33357, .T. ) ;
#70127=ADVANCED_FACE ( 'NONE', ( #24991 ), #52457, .F. ) ;
#70148=CARTESIAN_POINT ( 'NONE',  ( 20.00000000000000000, -4.000000000000000000, 29.75000000000000355 ) ) ;
#70151=EDGE_CURVE ( 'NONE', #48865, #59129, #13258, .T. ) ;
#70154=DIRECTION ( 'NONE',  ( -0.000000000000000000, 1.000000000000000000, -0.000000000000000000 ) ) ;
#70166=ADVANCED_FACE ( 'NONE', ( #60552 ), #33965, .T. ) ;
#70180=DIRECTION ( 'NONE',  ( -1.000000000000000000, -0.000000000000000000, -0.000000000000000000 ) ) ;
#70213=EDGE_CURVE ( 'NONE', #5990, #19429, #53794, .T. ) ;
#70216=FACE_OUTER_BOUND ( 'NONE', #17149, .T. ) ;
#70225=ORIENTED_EDGE ( 'NONE', *, *, #40029, .F. ) ;
#70236=CYLINDRICAL_SURFACE ( 'NONE', #74120, 4.000000000000000000 ) ;
#70241=CARTESIAN_POINT ( 'NONE',  ( -8.352564102564102200, -7.500000000000000000, 29.75000000000000355 ) ) ;
#70255=CIRCLE ( 'NONE', #31432, 4.000000000000000000 ) ;
#70273=PLANE ( 'NONE',  #26168 ) ;
#70309=DIRECTION ( 'NONE',  ( -1.000000000000000000, -0.000000000000000000, -0.000000000000000000 ) ) ;
#70323=AXIS2_PLACEMENT_3D ( 'NONE', #50917, #9954, #8193 ) ;
#70325=AXIS2_PLACEMENT_3D ( 'NONE', #7037, #26434, #75494 ) ;
#70328=AXIS2_PLACEMENT_3D ( 'NONE', #51075, #43016, #30825 ) ;
#70345=EDGE_CURVE ( 'NONE', #54542, #24890, #39678, .T. ) ;
#70355=CARTESIAN_POINT ( 'NONE',  ( -19.50000000000000000, -3.499999999999999556, 29.75000000000000355 ) ) ;
#70373=DIRECTION ( 'NONE',  ( 1.000000000000000000, 0.000000000000000000, 0.000000000000000000 ) ) ;
#70374=ORIENTED_EDGE ( 'NONE', *, *, #393, .T. ) ;
#70381=AXIS2_PLACEMENT_3D ( 'NONE', #58832, #18302, #41126 ) ;
#70386=CARTESIAN_POINT ( 'NONE',  ( 0.6089743589743582541, -7.500000000000000000, 29.75000000000000355 ) ) ;
#70395=VECTOR ( 'NONE', #28430, 1000.000000000000000 ) ;
#70414=DIRECTION ( 'NONE',  ( 0.000000000000000000, 0.000000000000000000, -1.000000000000000000 ) ) ;
#70417=CARTESIAN_POINT ( 'NONE',  ( -19.50000000000000000, -11.50000000000000000, 29.75000000000000355 ) ) ;
#70427=CARTESIAN_POINT ( 'NONE',  ( -14.16025641025641058, -7.500000000000000000, 33.75000000000000000 ) ) ;
#70428=ORIENTED_EDGE ( 'NONE', *, *, #82243, .T. ) ;
#70437=LINE ( 'NONE', #7408, #76550 ) ;
#70451=VECTOR ( 'NONE', #66965, 1000.000000000000000 ) ;
#70452=VECTOR ( 'NONE', #18510, 1000.000000000000000 ) ;
#70453=ORIENTED_EDGE ( 'NONE', *, *, #38274, .F. ) ;
#70460=DIRECTION ( 'NONE',  ( -0.000000000000000000, 1.000000000000000000, -0.000000000000000000 ) ) ;
#70465=VERTEX_POINT ( 'NONE', #56239 ) ;
#70467=CARTESIAN_POINT ( 'NONE',  ( 9.320512820512821150, -3.499999999999999556, 29.75000000000000355 ) ) ;
#70508=ORIENTED_EDGE ( 'NONE', *, *, #28048, .F. ) ;
#70511=ORIENTED_EDGE ( 'NONE', *, *, #54079, .T. ) ;
#70522=( GEOMETRIC_REPRESENTATION_CONTEXT ( 3 ) GLOBAL_UNCERTAINTY_ASSIGNED_CONTEXT ( ( #49200 ) ) GLOBAL_UNIT_ASSIGNED_CONTEXT ( ( #55033, #27561, #61324 ) ) REPRESENTATION_CONTEXT ( 'NONE', 'WORKASPACE' ) );
#70525=LINE ( 'NONE', #21448, #11822 ) ;
#70541=ORIENTED_EDGE ( 'NONE', *, *, #80765, .F. ) ;
#70569=ORIENTED_EDGE ( 'NONE', *, *, #26104, .T. ) ;
#70577=DIRECTION ( 'NONE',  ( -0.000000000000000000, 1.000000000000000000, -0.000000000000000000 ) ) ;
#70589=DIRECTION ( 'NONE',  ( 0.000000000000000000, 0.000000000000000000, -1.000000000000000000 ) ) ;
#70597=CARTESIAN_POINT ( 'NONE',  ( 0.000000000000000000, -11.00000000000000000, 29.75000000000000355 ) ) ;
#70602=FACE_OUTER_BOUND ( 'NONE', #32986, .T. ) ;
#70608=ORIENTED_EDGE ( 'NONE', *, *, #10844, .T. ) ;
#70626=CARTESIAN_POINT ( 'NONE',  ( -19.50000000000000000, -3.499999999999999556, 29.75000000000000355 ) ) ;
#70631=AXIS2_PLACEMENT_3D ( 'NONE', #74906, #21269, #75344 ) ;
#70649=PLANE ( 'NONE',  #71000 ) ;
#70650=CARTESIAN_POINT ( 'NONE',  ( 5.448717948717947124, -3.499999999999999556, 29.75000000000000355 ) ) ;
#70661=EDGE_CURVE ( 'NONE', #43749, #78293, #35973, .T. ) ;
#70671=ADVANCED_FACE ( 'NONE', ( #1734 ), #51667, .T. ) ;
#70688=CARTESIAN_POINT ( 'NONE',  ( 13.19230769230769340, -7.500000000000000000, 29.75000000000000355 ) ) ;
#70724=CARTESIAN_POINT ( 'NONE',  ( 4.230769230769229061, -3.499999999999999556, 29.75000000000000355 ) ) ;
#70729=VERTEX_POINT ( 'NONE', #60665 ) ;
#70755=VERTEX_POINT ( 'NONE', #86391 ) ;
#70762=AXIS2_PLACEMENT_3D ( 'NONE', #86681, #24947, #77671 ) ;
#70771=CIRCLE ( 'NONE', #16115, 4.000000000000000000 ) ;
#70775=EDGE_CURVE ( 'NONE', #26164, #79365, #78538, .T. ) ;
#70794=LINE ( 'NONE', #58585, #17475 ) ;
#70806=EDGE_LOOP ( 'NONE', ( #50250, #32371, #84755, #14657 ) ) ;
#70828=CIRCLE ( 'NONE', #67929, 4.000000000000000000 ) ;
#70842=CARTESIAN_POINT ( 'NONE',  ( -15.84615384615384670, -7.500000000000000000, 29.75000000000000355 ) ) ;
#70851=PLANE ( 'NONE',  #4740 ) ;
#70858=ORIENTED_EDGE ( 'NONE', *, *, #45840, .T. ) ;
#70867=AXIS2_PLACEMENT_3D ( 'NONE', #85804, #59985, #51092 ) ;
#70898=ORIENTED_EDGE ( 'NONE', *, *, #55465, .F. ) ;
#70908=ORIENTED_EDGE ( 'NONE', *, *, #87789, .T. ) ;
#70911=EDGE_LOOP ( 'NONE', ( #43955, #57177, #65461, #4561, #14862 ) ) ;
#70919=EDGE_CURVE ( 'NONE', #21459, #82878, #36743, .T. ) ;
#70920=ORIENTED_EDGE ( 'NONE', *, *, #42726, .T. ) ;
#70927=CARTESIAN_POINT ( 'NONE',  ( 0.3589743589743586982, -3.499999999999999556, 29.75000000000000355 ) ) ;
#70930=CARTESIAN_POINT ( 'NONE',  ( 9.320512820512821150, -4.000000000000000000, 29.75000000000000355 ) ) ;
#70946=AXIS2_PLACEMENT_3D ( 'NONE', #80912, #59285, #11554 ) ;
#70949=VECTOR ( 'NONE', #47960, 1000.000000000000000 ) ;
#70952=CARTESIAN_POINT ( 'NONE',  ( 14.16025641025641235, -3.499999999999999556, 29.75000000000000355 ) ) ;
#70967=DIRECTION ( 'NONE',  ( -0.000000000000000000, 1.000000000000000000, -0.000000000000000000 ) ) ;
#70971=EDGE_CURVE ( 'NONE', #87104, #17208, #58784, .T. ) ;
#70979=CARTESIAN_POINT ( 'NONE',  ( -17.78205128205128105, -7.500000000000000000, 33.75000000000000000 ) ) ;
#70986=ORIENTED_EDGE ( 'NONE', *, *, #51166, .T. ) ;
#70999=PLANE ( 'NONE',  #37959 ) ;
#71000=AXIS2_PLACEMENT_3D ( 'NONE', #3060, #30101, #9826 ) ;
#71001=AXIS2_PLACEMENT_3D ( 'NONE', #48077, #34576, #26050 ) ;
#71005=EDGE_LOOP ( 'NONE', ( #66351, #35462, #21270, #5979 ) ) ;
#71010=ORIENTED_EDGE ( 'NONE', *, *, #76518, .F. ) ;
#71012=CARTESIAN_POINT ( 'NONE',  ( 4.480769230769229061, -3.499999999999999556, 29.75000000000000355 ) ) ;
#71026=DIRECTION ( 'NONE',  ( -1.000000000000000000, -0.000000000000000000, -0.000000000000000000 ) ) ;
#71027=ORIENTED_EDGE ( 'NONE', *, *, #83072, .T. ) ;
#71028=PLANE ( 'NONE',  #76297 ) ;
#71054=DIRECTION ( 'NONE',  ( 1.000000000000000000, 0.000000000000000000, 0.000000000000000000 ) ) ;
#71061=EDGE_CURVE ( 'NONE', #23619, #17400, #39428, .T. ) ;
#71062=VECTOR ( 'NONE', #65905, 1000.000000000000000 ) ;
#71063=LINE ( 'NONE', #76500, #4540 ) ;
#71069=VECTOR ( 'NONE', #59909, 1000.000000000000000 ) ;
#71088=PLANE ( 'NONE',  #74546 ) ;
#71093=VERTEX_POINT ( 'NONE', #59232 ) ;
#71110=EDGE_LOOP ( 'NONE', ( #8666, #51391, #16912, #80900 ) ) ;
#71122=DIRECTION ( 'NONE',  ( -1.000000000000000000, -0.000000000000000000, -0.000000000000000000 ) ) ;
#71128=ORIENTED_EDGE ( 'NONE', *, *, #13316, .F. ) ;
#71130=CARTESIAN_POINT ( 'NONE',  ( -6.166666666666667851, -3.499999999999999556, 29.75000000000000355 ) ) ;
#71145=ORIENTED_EDGE ( 'NONE', *, *, #51318, .F. ) ;
#71147=EDGE_CURVE ( 'NONE', #33955, #22635, #7405, .T. ) ;
#71153=DIRECTION ( 'NONE',  ( 1.000000000000000000, 0.000000000000000000, 0.000000000000000000 ) ) ;
#71175=DIRECTION ( 'NONE',  ( 1.000000000000000000, 0.000000000000000000, 0.000000000000000000 ) ) ;
#71190=AXIS2_PLACEMENT_3D ( 'NONE', #75835, #20886, #6501 ) ;
#71211=VECTOR ( 'NONE', #64732, 1000.000000000000000 ) ;
#71221=DIRECTION ( 'NONE',  ( -1.000000000000000000, -0.000000000000000000, 0.000000000000000000 ) ) ;
#71230=LINE ( 'NONE', #64464, #21636 ) ;
#71231=CARTESIAN_POINT ( 'NONE',  ( -11.25641025641025550, -3.499999999999999556, 29.75000000000000355 ) ) ;
#71240=ADVANCED_FACE ( 'NONE', ( #47041 ), #41629, .F. ) ;
#71250=DIRECTION ( 'NONE',  ( -1.000000000000000000, -0.000000000000000000, 0.000000000000000000 ) ) ;
#71270=CARTESIAN_POINT ( 'NONE',  ( 11.25641025641025550, -3.499999999999999556, 29.75000000000000355 ) ) ;
#71272=EDGE_CURVE ( 'NONE', #34255, #30233, #74529, .T. ) ;
#71274=ORIENTED_EDGE ( 'NONE', *, *, #48086, .T. ) ;
#71275=EDGE_CURVE ( 'NONE', #75229, #34232, #40309, .T. ) ;
#71288=LINE ( 'NONE', #75508, #3819 ) ;
#71305=EDGE_CURVE ( 'NONE', #5154, #5809, #15932, .T. ) ;
#71306=AXIS2_PLACEMENT_3D ( 'NONE', #24626, #51181, #52092 ) ;
#71321=ORIENTED_EDGE ( 'NONE', *, *, #24672, .F. ) ;
#71339=LINE ( 'NONE', #9641, #66191 ) ;
#71359=DIRECTION ( 'NONE',  ( 0.000000000000000000, 0.000000000000000000, -1.000000000000000000 ) ) ;
#71368=DIRECTION ( 'NONE',  ( 1.000000000000000000, 0.000000000000000000, 0.000000000000000000 ) ) ;
#71388=LINE ( 'NONE', #9694, #2913 ) ;
#71390=LINE ( 'NONE', #65074, #34567 ) ;
#71393=EDGE_CURVE ( 'NONE', #34447, #30367, #57791, .T. ) ;
#71397=EDGE_CURVE ( 'NONE', #80799, #30362, #15369, .T. ) ;
#71410=LINE ( 'NONE', #9719, #22798 ) ;
#71420=ADVANCED_FACE ( 'NONE', ( #85276 ), #16367, .T. ) ;
#71424=ORIENTED_EDGE ( 'NONE', *, *, #7584, .T. ) ;
#71425=ADVANCED_FACE ( 'NONE', ( #23996 ), #10501, .F. ) ;
#71428=LINE ( 'NONE', #50709, #40230 ) ;
#71435=VERTEX_POINT ( 'NONE', #25341 ) ;
#71455=LINE ( 'NONE', #10215, #69908 ) ;
#71459=VERTEX_POINT ( 'NONE', #10045 ) ;
#71460=CARTESIAN_POINT ( 'NONE',  ( 4.230769230769229061, -11.00000000000000000, 29.75000000000000355 ) ) ;
#71462=EDGE_LOOP ( 'NONE', ( #75455, #85680, #12939, #21692 ) ) ;
#71466=DIRECTION ( 'NONE',  ( 0.000000000000000000, 0.000000000000000000, -1.000000000000000000 ) ) ;
#71477=DIRECTION ( 'NONE',  ( -0.000000000000000000, 1.000000000000000000, -0.000000000000000000 ) ) ;
#71495=ADVANCED_FACE ( 'NONE', ( #59565 ), #86619, .T. ) ;
#71496=CIRCLE ( 'NONE', #70017, 4.000000000000000000 ) ;
#71499=EDGE_LOOP ( 'NONE', ( #53934, #72120, #47879, #48320 ) ) ;
#71502=AXIS2_PLACEMENT_3D ( 'NONE', #77927, #36936, #23420 ) ;
#71510=DIRECTION ( 'NONE',  ( 1.000000000000000000, 0.000000000000000000, 0.000000000000000000 ) ) ;
#71523=CARTESIAN_POINT ( 'NONE',  ( 6.166666666666664298, -3.499999999999999556, 29.75000000000000355 ) ) ;
#71532=DIRECTION ( 'NONE',  ( 0.000000000000000000, 0.000000000000000000, -1.000000000000000000 ) ) ;
#71534=ORIENTED_EDGE ( 'NONE', *, *, #83641, .F. ) ;
#71552=LINE ( 'NONE', #66129, #67619 ) ;
#71555=VECTOR ( 'NONE', #57719, 1000.000000000000000 ) ;
#71579=CARTESIAN_POINT ( 'NONE',  ( 12.94230769230769340, -3.499999999999999556, 29.75000000000000355 ) ) ;
#71592=CARTESIAN_POINT ( 'NONE',  ( -16.81410256410256565, -4.000000000000000000, 29.75000000000000355 ) ) ;
#71620=DIRECTION ( 'NONE',  ( 1.000000000000000000, 0.000000000000000000, 0.000000000000000000 ) ) ;
#71629=CIRCLE ( 'NONE', #14099, 4.000000000000000000 ) ;
#71633=CARTESIAN_POINT ( 'NONE',  ( -10.28846153846153832, -7.500000000000000000, 33.75000000000000000 ) ) ;
#71637=CARTESIAN_POINT ( 'NONE',  ( -19.50000000000000000, -3.499999999999999556, 29.75000000000000355 ) ) ;
#71650=VECTOR ( 'NONE', #3894, 1000.000000000000000 ) ;
#71666=ADVANCED_FACE ( 'NONE', ( #20799 ), #13602, .F. ) ;
#71669=EDGE_CURVE ( 'NONE', #30978, #5298, #32991, .T. ) ;
#71687=LINE ( 'NONE', #22186, #5619 ) ;
#71701=ORIENTED_EDGE ( 'NONE', *, *, #84771, .T. ) ;
#71704=PLANE ( 'NONE',  #25198 ) ;
#71724=CARTESIAN_POINT ( 'NONE',  ( 18.03205128205128105, -3.499999999999999556, 29.75000000000000355 ) ) ;
#71733=LINE ( 'NONE', #62861, #81510 ) ;
#71736=CARTESIAN_POINT ( 'NONE',  ( 0.000000000000000000, -11.00000000000000000, 29.75000000000000355 ) ) ;
#71741=CARTESIAN_POINT ( 'NONE',  ( -19.50000000000000000, -3.499999999999999556, 29.75000000000000355 ) ) ;
#71743=EDGE_LOOP ( 'NONE', ( #7269, #69227, #32339, #36574 ) ) ;
#71745=DIRECTION ( 'NONE',  ( 0.000000000000000000, 0.000000000000000000, -1.000000000000000000 ) ) ;
#71746=FACE_OUTER_BOUND ( 'NONE', #43530, .T. ) ;
#71758=DIRECTION ( 'NONE',  ( -1.000000000000000000, -0.000000000000000000, -0.000000000000000000 ) ) ;
#71767=DIRECTION ( 'NONE',  ( -0.000000000000000000, 1.000000000000000000, -0.000000000000000000 ) ) ;
#71778=CARTESIAN_POINT ( 'NONE',  ( -19.50000000000000000, -11.50000000000000000, 29.75000000000000355 ) ) ;
#71779=ORIENTED_EDGE ( 'NONE', *, *, #84038, .F. ) ;
#71780=VERTEX_POINT ( 'NONE', #72528 ) ;
#71782=VECTOR ( 'NONE', #29485, 1000.000000000000000 ) ;
#71783=DIRECTION ( 'NONE',  ( -0.000000000000000000, 1.000000000000000000, -0.000000000000000000 ) ) ;
#71791=ORIENTED_EDGE ( 'NONE', *, *, #21616, .F. ) ;
#71829=CARTESIAN_POINT ( 'NONE',  ( 20.00000000000000000, -4.000000000000000000, 29.75000000000000355 ) ) ;
#71851=CARTESIAN_POINT ( 'NONE',  ( -19.50000000000000000, -3.499999999999999556, 29.75000000000000355 ) ) ;
#71861=VERTEX_POINT ( 'NONE', #71633 ) ;
#71864=EDGE_LOOP ( 'NONE', ( #44677, #33783, #16608, #8367 ) ) ;
#71894=LINE ( 'NONE', #87656, #81150 ) ;
#71903=VECTOR ( 'NONE', #49877, 1000.000000000000000 ) ;
#71916=CYLINDRICAL_SURFACE ( 'NONE', #42941, 4.000000000000000000 ) ;
#71923=LINE ( 'NONE', #86804, #4084 ) ;
#71965=EDGE_CURVE ( 'NONE', #79365, #47433, #80475, .T. ) ;
#71971=AXIS2_PLACEMENT_3D ( 'NONE', #59728, #60607, #26391 ) ;
#71995=EDGE_CURVE ( 'NONE', #36536, #3856, #80039, .T. ) ;
#71999=DIRECTION ( 'NONE',  ( -0.000000000000000000, 1.000000000000000000, -0.000000000000000000 ) ) ;
#72023=CARTESIAN_POINT ( 'NONE',  ( -11.25641025641025550, -3.499999999999999556, 29.75000000000000355 ) ) ;
#72043=PRODUCT_DEFINITION_FORMATION_WITH_SPECIFIED_SOURCE ( 'ANY', '', #88677, .NOT_KNOWN. ) ;
#72047=LINE ( 'NONE', #79707, #12332 ) ;
#72054=DIRECTION ( 'NONE',  ( 0.000000000000000000, 1.000000000000000000, 0.000000000000000000 ) ) ;
#72056=ORIENTED_EDGE ( 'NONE', *, *, #28727, .T. ) ;
#72058=DIRECTION ( 'NONE',  ( 0.000000000000000000, 0.000000000000000000, 1.000000000000000000 ) ) ;
#72074=EDGE_CURVE ( 'NONE', #856, #8541, #55469, .T. ) ;
#72107=EDGE_LOOP ( 'NONE', ( #33996, #41969, #81017, #76783, #20129 ) ) ;
#72120=ORIENTED_EDGE ( 'NONE', *, *, #27938, .F. ) ;
#72130=DIRECTION ( 'NONE',  ( -0.000000000000000000, 1.000000000000000000, -0.000000000000000000 ) ) ;
#72136=ORIENTED_EDGE ( 'NONE', *, *, #59719, .F. ) ;
#72142=VERTEX_POINT ( 'NONE', #69059 ) ;
#72145=FACE_OUTER_BOUND ( 'NONE', #34539, .T. ) ;
#72149=VERTEX_POINT ( 'NONE', #88913 ) ;
#72168=CARTESIAN_POINT ( 'NONE',  ( -16.81410256410256565, -11.00000000000000000, 29.75000000000000355 ) ) ;
#72174=CARTESIAN_POINT ( 'NONE',  ( 11.25641025641025550, -3.499999999999999556, 29.75000000000000355 ) ) ;
#72180=EDGE_CURVE ( 'NONE', #11602, #1493, #28073, .T. ) ;
#72185=ORIENTED_EDGE ( 'NONE', *, *, #82932, .T. ) ;
#72193=DIRECTION ( 'NONE',  ( -0.000000000000000000, 1.000000000000000000, -0.000000000000000000 ) ) ;
#72194=CARTESIAN_POINT ( 'NONE',  ( 0.000000000000000000, -11.00000000000000000, 29.75000000000000355 ) ) ;
#72199=DIRECTION ( 'NONE',  ( 0.000000000000000000, 0.000000000000000000, -1.000000000000000000 ) ) ;
#72212=CIRCLE ( 'NONE', #46312, 4.000000000000000000 ) ;
#72219=AXIS2_PLACEMENT_3D ( 'NONE', #21076, #76027, #61178 ) ;
#72221=VECTOR ( 'NONE', #5749, 1000.000000000000000 ) ;
#72229=ORIENTED_EDGE ( 'NONE', *, *, #38918, .T. ) ;
#72235=LINE ( 'NONE', #38463, #69624 ) ;
#72237=ORIENTED_EDGE ( 'NONE', *, *, #42303, .T. ) ;
#72244=VERTEX_POINT ( 'NONE', #79020 ) ;
#72259=DIRECTION ( 'NONE',  ( -0.000000000000000000, 1.000000000000000000, -0.000000000000000000 ) ) ;
#72288=CARTESIAN_POINT ( 'NONE',  ( 3.512820512820510555, -11.00000000000000000, 29.75000000000000355 ) ) ;
#72293=VERTEX_POINT ( 'NONE', #31732 ) ;
#72301=CARTESIAN_POINT ( 'NONE',  ( -13.91025641025641058, -3.499999999999999556, 29.75000000000000355 ) ) ;
#72302=VECTOR ( 'NONE', #1861, 1000.000000000000000 ) ;
#72308=ORIENTED_EDGE ( 'NONE', *, *, #15824, .F. ) ;
#72318=ADVANCED_FACE ( 'NONE', ( #37135 ), #57858, .T. ) ;
#72328=ORIENTED_EDGE ( 'NONE', *, *, #82751, .T. ) ;
#72332=ORIENTED_EDGE ( 'NONE', *, *, #24288, .F. ) ;
#72342=LINE ( 'NONE', #77774, #6963 ) ;
#72346=CARTESIAN_POINT ( 'NONE',  ( -2.294871794871794712, -7.500000000000000000, 29.75000000000000355 ) ) ;
#72354=EDGE_CURVE ( 'NONE', #50277, #34333, #68616, .T. ) ;
#72355=EDGE_LOOP ( 'NONE', ( #31561, #35216, #53786, #50488 ) ) ;
#72358=CARTESIAN_POINT ( 'NONE',  ( -19.00000000000000000, -4.000000000000000000, 29.75000000000000355 ) ) ;
#72389=LINE ( 'NONE', #16126, #57079 ) ;
#72398=CARTESIAN_POINT ( 'NONE',  ( 3.512820512820510555, -3.499999999999999556, 29.75000000000000355 ) ) ;
#72404=DIRECTION ( 'NONE',  ( 0.000000000000000000, 0.000000000000000000, -1.000000000000000000 ) ) ;
#72406=ORIENTED_EDGE ( 'NONE', *, *, #83353, .T. ) ;
#72411=ORIENTED_EDGE ( 'NONE', *, *, #47371, .T. ) ;
#72421=EDGE_CURVE ( 'NONE', #72293, #63049, #8257, .T. ) ;
#72434=EDGE_CURVE ( 'NONE', #48052, #5565, #42486, .T. ) ;
#72437=LINE ( 'NONE', #4891, #55979 ) ;
#72440=DIRECTION ( 'NONE',  ( -1.000000000000000000, -0.000000000000000000, -0.000000000000000000 ) ) ;
#72483=DIRECTION ( 'NONE',  ( 0.000000000000000000, 1.000000000000000000, 0.000000000000000000 ) ) ;
#72487=DIRECTION ( 'NONE',  ( 0.000000000000000000, 0.000000000000000000, -1.000000000000000000 ) ) ;
#72492=VERTEX_POINT ( 'NONE', #48338 ) ;
#72501=DIRECTION ( 'NONE',  ( 0.000000000000000000, 0.000000000000000000, -1.000000000000000000 ) ) ;
#72514=VECTOR ( 'NONE', #63948, 1000.000000000000000 ) ;
#72528=CARTESIAN_POINT ( 'NONE',  ( -7.384615384615385025, -7.500000000000000000, 33.75000000000000000 ) ) ;
#72532=DIRECTION ( 'NONE',  ( 0.000000000000000000, 0.000000000000000000, -1.000000000000000000 ) ) ;
#72534=EDGE_CURVE ( 'NONE', #30751, #15288, #45566, .T. ) ;
#72553=EDGE_CURVE ( 'NONE', #52150, #54472, #16766, .T. ) ;
#72560=CARTESIAN_POINT ( 'NONE',  ( -0.6089743589743589203, -11.50000000000000000, 29.75000000000000355 ) ) ;
#72564=VERTEX_POINT ( 'NONE', #86131 ) ;
#72565=LINE ( 'NONE', #7883, #69026 ) ;
#72571=LINE ( 'NONE', #58161, #57798 ) ;
#72577=ADVANCED_FACE ( 'NONE', ( #12686 ), #13567, .T. ) ;
#72590=ORIENTED_EDGE ( 'NONE', *, *, #7677, .T. ) ;
#72597=CARTESIAN_POINT ( 'NONE',  ( -19.50000000000000000, -3.499999999999999556, 29.75000000000000355 ) ) ;
#72608=EDGE_LOOP ( 'NONE', ( #81870, #52827, #28538, #34789 ) ) ;
#72639=AXIS2_PLACEMENT_3D ( 'NONE', #83765, #22054, #43641 ) ;
#72647=DIRECTION ( 'NONE',  ( -1.000000000000000000, 0.000000000000000000, -0.000000000000000000 ) ) ;
#72650=FACE_OUTER_BOUND ( 'NONE', #37754, .T. ) ;
#72659=AXIS2_PLACEMENT_3D ( 'NONE', #37012, #70373, #7784 ) ;
#72670=ORIENTED_EDGE ( 'NONE', *, *, #16437, .F. ) ;
#72677=LINE ( 'NONE', #10988, #44575 ) ;
#72685=ORIENTED_EDGE ( 'NONE', *, *, #72877, .T. ) ;
#72694=PLANE ( 'NONE',  #44710 ) ;
#72701=DIRECTION ( 'NONE',  ( -1.000000000000000000, 0.000000000000000000, -0.000000000000000000 ) ) ;
#72716=PLANE ( 'NONE',  #67781 ) ;
#72727=CARTESIAN_POINT ( 'NONE',  ( 2.544871794871792936, -3.499999999999999556, 29.75000000000000355 ) ) ;
#72740=FACE_OUTER_BOUND ( 'NONE', #86789, .T. ) ;
#72749=ORIENTED_EDGE ( 'NONE', *, *, #43835, .F. ) ;
#72755=ADVANCED_FACE ( 'NONE', ( #49125 ), #14009, .T. ) ;
#72758=AXIS2_PLACEMENT_3D ( 'NONE', #49912, #23761, #51214 ) ;
#72764=LINE ( 'NONE', #66003, #87691 ) ;
#72766=CARTESIAN_POINT ( 'NONE',  ( 20.00000000000000000, -4.000000000000000000, 29.75000000000000355 ) ) ;
#72770=ORIENTED_EDGE ( 'NONE', *, *, #35171, .F. ) ;
#72777=VECTOR ( 'NONE', #40272, 1000.000000000000000 ) ;
#72794=CYLINDRICAL_SURFACE ( 'NONE', #27446, 4.000000000000000000 ) ;
#72842=LINE ( 'NONE', #39533, #74706 ) ;
#72858=EDGE_CURVE ( 'NONE', #48029, #45953, #72047, .T. ) ;
#72877=EDGE_CURVE ( 'NONE', #44505, #32252, #67183, .T. ) ;
#72890=DIRECTION ( 'NONE',  ( 0.000000000000000000, 0.000000000000000000, -1.000000000000000000 ) ) ;
#72917=DIRECTION ( 'NONE',  ( 0.000000000000000000, 0.000000000000000000, -1.000000000000000000 ) ) ;
#72920=LINE ( 'NONE', #67508, #31546 ) ;
#72924=FACE_OUTER_BOUND ( 'NONE', #56448, .T. ) ;
#72930=FACE_OUTER_BOUND ( 'NONE', #35365, .T. ) ;
#72932=AXIS2_PLACEMENT_3D ( 'NONE', #45225, #51074, #72701 ) ;
#72952=CYLINDRICAL_SURFACE ( 'NONE', #31230, 4.000000000000000000 ) ;
#72963=DIRECTION ( 'NONE',  ( -0.000000000000000000, -1.000000000000000000, -0.000000000000000000 ) ) ;
#72972=CIRCLE ( 'NONE', #36953, 4.000000000000000000 ) ;
#72975=DIRECTION ( 'NONE',  ( -1.000000000000000000, -0.000000000000000000, -0.000000000000000000 ) ) ;
#72976=ORIENTED_EDGE ( 'NONE', *, *, #8495, .F. ) ;
#72994=VECTOR ( 'NONE', #78082, 1000.000000000000000 ) ;
#73010=ADVANCED_FACE ( 'NONE', ( #80152 ), #26093, .T. ) ;
#73012=LINE ( 'NONE', #18073, #28061 ) ;
#73021=VECTOR ( 'NONE', #62081, 1000.000000000000000 ) ;
#73026=DIRECTION ( 'NONE',  ( 0.000000000000000000, 0.000000000000000000, -1.000000000000000000 ) ) ;
#73027=CARTESIAN_POINT ( 'NONE',  ( 5.198717948717946236, -7.500000000000000000, 33.75000000000000000 ) ) ;
#73028=DIRECTION ( 'NONE',  ( -0.000000000000000000, 1.000000000000000000, -0.000000000000000000 ) ) ;
#73046=CARTESIAN_POINT ( 'NONE',  ( -8.102564102564102200, -3.499999999999999556, 29.75000000000000355 ) ) ;
#73070=EDGE_CURVE ( 'NONE', #13635, #33955, #48323, .T. ) ;
#73078=ORIENTED_EDGE ( 'NONE', *, *, #53955, .T. ) ;
#73098=CARTESIAN_POINT ( 'NONE',  ( -16.81410256410256565, -7.500000000000000000, 33.75000000000000000 ) ) ;
#73105=CARTESIAN_POINT ( 'NONE',  ( -10.03846153846153832, -11.50000000000000000, 29.75000000000000355 ) ) ;
#73112=LINE ( 'NONE', #10526, #63174 ) ;
#73118=ADVANCED_FACE ( 'NONE', ( #28759 ), #41831, .T. ) ;
#73120=DIRECTION ( 'NONE',  ( 0.000000000000000000, 0.000000000000000000, -1.000000000000000000 ) ) ;
#73121=LINE ( 'NONE', #30357, #71062 ) ;
#73130=EDGE_CURVE ( 'NONE', #46484, #29630, #15246, .T. ) ;
#73153=VECTOR ( 'NONE', #5203, 1000.000000000000000 ) ;
#73177=EDGE_CURVE ( 'NONE', #17849, #87793, #69736, .T. ) ;
#73194=CARTESIAN_POINT ( 'NONE',  ( 0.000000000000000000, -11.00000000000000000, 29.75000000000000355 ) ) ;
#73202=CARTESIAN_POINT ( 'NONE',  ( -19.50000000000000000, -3.499999999999999556, 29.75000000000000355 ) ) ;
#73223=CARTESIAN_POINT ( 'NONE',  ( -16.09615384615384670, -3.499999999999999556, 29.75000000000000355 ) ) ;
#73224=CARTESIAN_POINT ( 'NONE',  ( -8.102564102564102200, -3.499999999999999556, 29.75000000000000355 ) ) ;
#73242=CARTESIAN_POINT ( 'NONE',  ( -19.50000000000000000, -3.499999999999999556, 29.75000000000000355 ) ) ;
#73249=CARTESIAN_POINT ( 'NONE',  ( -11.00641025641025550, -7.500000000000000000, 29.75000000000000355 ) ) ;
#73274=CARTESIAN_POINT ( 'NONE',  ( 20.00000000000000000, -3.499999999999999556, 28.25000000000000000 ) ) ;
#73275=CARTESIAN_POINT ( 'NONE',  ( 12.22435897435897267, -11.50000000000000000, 29.75000000000000355 ) ) ;
#73302=ORIENTED_EDGE ( 'NONE', *, *, #75181, .F. ) ;
#73325=ORIENTED_EDGE ( 'NONE', *, *, #76405, .T. ) ;
#73336=ORIENTED_EDGE ( 'NONE', *, *, #48944, .F. ) ;
#73348=FACE_OUTER_BOUND ( 'NONE', #78295, .T. ) ;
#73353=CARTESIAN_POINT ( 'NONE',  ( -9.320512820512821150, -7.500000000000000000, 29.75000000000000355 ) ) ;
#73355=ORIENTED_EDGE ( 'NONE', *, *, #38599, .T. ) ;
#73366=VERTEX_POINT ( 'NONE', #57541 ) ;
#73380=EDGE_CURVE ( 'NONE', #57194, #53391, #66978, .T. ) ;
#73388=CARTESIAN_POINT ( 'NONE',  ( -6.166666666666667851, -3.499999999999999556, 29.75000000000000355 ) ) ;
#73391=FACE_OUTER_BOUND ( 'NONE', #50319, .T. ) ;
#73394=DIRECTION ( 'NONE',  ( 1.000000000000000000, 0.000000000000000000, 0.000000000000000000 ) ) ;
#73395=CARTESIAN_POINT ( 'NONE',  ( 11.00641025641025550, -3.499999999999999556, 29.75000000000000355 ) ) ;
#73427=EDGE_CURVE ( 'NONE', #45168, #71435, #39071, .T. ) ;
#73448=VERTEX_POINT ( 'NONE', #45356 ) ;
#73459=VECTOR ( 'NONE', #14996, 1000.000000000000000 ) ;
#73467=VECTOR ( 'NONE', #52004, 1000.000000000000000 ) ;
#73468=VECTOR ( 'NONE', #62170, 1000.000000000000000 ) ;
#73475=CARTESIAN_POINT ( 'NONE',  ( 20.00000000000000000, -11.50000000000000000, 29.75000000000000355 ) ) ;
#73478=ADVANCED_FACE ( 'NONE', ( #21443 ), #75496, .F. ) ;
#73521=LINE ( 'NONE', #45140, #57027 ) ;
#73524=DIRECTION ( 'NONE',  ( -1.000000000000000000, -0.000000000000000000, 0.000000000000000000 ) ) ;
#73531=VECTOR ( 'NONE', #20873, 1000.000000000000000 ) ;
#73542=CARTESIAN_POINT ( 'NONE',  ( -19.50000000000000000, -3.499999999999999556, 29.75000000000000355 ) ) ;
#73543=DIRECTION ( 'NONE',  ( 0.000000000000000000, 0.000000000000000000, 1.000000000000000000 ) ) ;
#73551=EDGE_CURVE ( 'NONE', #66461, #18250, #33633, .T. ) ;
#73561=DIRECTION ( 'NONE',  ( 0.000000000000000000, 0.000000000000000000, -1.000000000000000000 ) ) ;
#73566=ORIENTED_EDGE ( 'NONE', *, *, #47248, .F. ) ;
#73570=ORIENTED_EDGE ( 'NONE', *, *, #69586, .F. ) ;
#73574=CYLINDRICAL_SURFACE ( 'NONE', #76097, 4.000000000000000000 ) ;
#73602=VECTOR ( 'NONE', #35023, 1000.000000000000000 ) ;
#73607=LINE ( 'NONE', #85778, #37834 ) ;
#73659=CARTESIAN_POINT ( 'NONE',  ( -12.94230769230769162, -3.499999999999999556, 29.75000000000000355 ) ) ;
#73664=ORIENTED_EDGE ( 'NONE', *, *, #19488, .T. ) ;
#73670=CARTESIAN_POINT ( 'NONE',  ( -19.50000000000000000, -3.499999999999999556, 29.75000000000000355 ) ) ;
#73675=EDGE_CURVE ( 'NONE', #33780, #81906, #28204, .T. ) ;
#73679=DIRECTION ( 'NONE',  ( -1.000000000000000000, -0.000000000000000000, -0.000000000000000000 ) ) ;
#73695=ORIENTED_EDGE ( 'NONE', *, *, #52463, .F. ) ;
#73697=VECTOR ( 'NONE', #8620, 1000.000000000000000 ) ;
#73705=PLANE ( 'NONE',  #81433 ) ;
#73712=ORIENTED_EDGE ( 'NONE', *, *, #50612, .F. ) ;
#73714=LINE ( 'NONE', #86796, #65574 ) ;
#73718=EDGE_CURVE ( 'NONE', #11602, #4346, #74858, .T. ) ;
#73730=VECTOR ( 'NONE', #61855, 1000.000000000000000 ) ;
#73741=VECTOR ( 'NONE', #58786, 1000.000000000000000 ) ;
#73751=LINE ( 'NONE', #74178, #5370 ) ;
#73760=DIRECTION ( 'NONE',  ( 1.000000000000000000, 0.000000000000000000, 0.000000000000000000 ) ) ;
#73790=VERTEX_POINT ( 'NONE', #61755 ) ;
#73796=ORIENTED_EDGE ( 'NONE', *, *, #20585, .F. ) ;
#73798=CARTESIAN_POINT ( 'NONE',  ( 7.384615384615385025, -7.500000000000000000, 29.75000000000000355 ) ) ;
#73809=DIRECTION ( 'NONE',  ( 1.000000000000000000, 0.000000000000000000, 0.000000000000000000 ) ) ;
#73811=ORIENTED_EDGE ( 'NONE', *, *, #10635, .T. ) ;
#73816=FACE_OUTER_BOUND ( 'NONE', #26374, .T. ) ;
#73817=CIRCLE ( 'NONE', #13374, 4.000000000000000000 ) ;
#73819=CARTESIAN_POINT ( 'NONE',  ( -1.326923076923076872, -3.499999999999999556, 29.75000000000000355 ) ) ;
#73824=EDGE_CURVE ( 'NONE', #57207, #42406, #19454, .T. ) ;
#73832=CARTESIAN_POINT ( 'NONE',  ( 9.070512820512819374, -3.499999999999999556, 29.75000000000000355 ) ) ;
#73850=CARTESIAN_POINT ( 'NONE',  ( 11.00641025641025550, -11.00000000000000000, 29.75000000000000355 ) ) ;
#73852=VERTEX_POINT ( 'NONE', #62643 ) ;
#73862=VERTEX_POINT ( 'NONE', #77499 ) ;
#73885=ORIENTED_EDGE ( 'NONE', *, *, #65459, .F. ) ;
#73923=LINE ( 'NONE', #39702, #19918 ) ;
#73941=CARTESIAN_POINT ( 'NONE',  ( -3.512820512820513663, -7.500000000000000000, 29.75000000000000355 ) ) ;
#73967=PLANE ( 'NONE',  #34163 ) ;
#73985=CARTESIAN_POINT ( 'NONE',  ( -9.070512820512819374, -3.499999999999999556, 29.75000000000000355 ) ) ;
#73988=PLANE ( 'NONE',  #52353 ) ;
#73992=ORIENTED_EDGE ( 'NONE', *, *, #46965, .F. ) ;
#73997=PLANE ( 'NONE',  #36434 ) ;
#73998=CARTESIAN_POINT ( 'NONE',  ( 12.94230769230769340, -11.00000000000000000, 29.75000000000000355 ) ) ;
#73999=EDGE_CURVE ( 'NONE', #47713, #52415, #79282, .T. ) ;
#74013=DIRECTION ( 'NONE',  ( 0.000000000000000000, 0.000000000000000000, -1.000000000000000000 ) ) ;
#74017=DIRECTION ( 'NONE',  ( 0.000000000000000000, 0.000000000000000000, -1.000000000000000000 ) ) ;
#74021=VERTEX_POINT ( 'NONE', #58108 ) ;
#74023=ORIENTED_EDGE ( 'NONE', *, *, #58420, .T. ) ;
#74030=AXIS2_PLACEMENT_3D ( 'NONE', #30146, #9431, #29712 ) ;
#74038=LINE ( 'NONE', #46114, #11614 ) ;
#74072=ORIENTED_EDGE ( 'NONE', *, *, #65459, .T. ) ;
#74082=ADVANCED_FACE ( 'NONE', ( #12160 ), #80173, .F. ) ;
#74088=EDGE_LOOP ( 'NONE', ( #46455, #75121, #15546, #74197 ) ) ;
#74093=CARTESIAN_POINT ( 'NONE',  ( -19.50000000000000000, -3.499999999999999556, 29.75000000000000355 ) ) ;
#74094=CARTESIAN_POINT ( 'NONE',  ( -15.12820512820512953, -4.000000000000000000, 29.75000000000000355 ) ) ;
#74096=ADVANCED_FACE ( 'NONE', ( #26561 ), #4958, .T. ) ;
#74097=VECTOR ( 'NONE', #5804, 1000.000000000000000 ) ;
#74103=CARTESIAN_POINT ( 'NONE',  ( 16.09615384615384670, -7.500000000000000000, 29.75000000000000355 ) ) ;
#74120=AXIS2_PLACEMENT_3D ( 'NONE', #50389, #8543, #84212 ) ;
#74126=ORIENTED_EDGE ( 'NONE', *, *, #57736, .T. ) ;
#74141=ORIENTED_EDGE ( 'NONE', *, *, #1103, .F. ) ;
#74162=ORIENTED_EDGE ( 'NONE', *, *, #30671, .F. ) ;
#74165=CARTESIAN_POINT ( 'NONE',  ( -11.25641025641025550, -7.500000000000000000, 33.75000000000000000 ) ) ;
#74175=CARTESIAN_POINT ( 'NONE',  ( 3.512820512820510555, -11.50000000000000000, 29.75000000000000355 ) ) ;
#74178=CARTESIAN_POINT ( 'NONE',  ( 19.00000000000000000, -3.499999999999999556, 29.75000000000000355 ) ) ;
#74179=VERTEX_POINT ( 'NONE', #82838 ) ;
#74197=ORIENTED_EDGE ( 'NONE', *, *, #32593, .F. ) ;
#74233=CARTESIAN_POINT ( 'NONE',  ( -12.22435897435897623, -4.000000000000000000, 29.75000000000000355 ) ) ;
#74245=AXIS2_PLACEMENT_3D ( 'NONE', #57652, #10802, #10356 ) ;
#74249=FACE_OUTER_BOUND ( 'NONE', #78888, .T. ) ;
#74258=LINE ( 'NONE', #59405, #5892 ) ;
#74271=PLANE ( 'NONE',  #21922 ) ;
#74280=CARTESIAN_POINT ( 'NONE',  ( 0.000000000000000000, -4.000000000000000000, 29.25000000000000000 ) ) ;
#74302=AXIS2_PLACEMENT_3D ( 'NONE', #11146, #10706, #30525 ) ;
#74315=FACE_OUTER_BOUND ( 'NONE', #28178, .T. ) ;
#74323=CARTESIAN_POINT ( 'NONE',  ( -1.326923076923076206, -4.000000000000000000, 29.75000000000000355 ) ) ;
#74340=ORIENTED_EDGE ( 'NONE', *, *, #9325, .T. ) ;
#74351=PLANE ( 'NONE',  #81240 ) ;
#74365=EDGE_LOOP ( 'NONE', ( #76897, #85311, #8779, #65605, #6877 ) ) ;
#74380=CYLINDRICAL_SURFACE ( 'NONE', #27291, 4.000000000000000000 ) ;
#74386=DIRECTION ( 'NONE',  ( 0.000000000000000000, 0.000000000000000000, -1.000000000000000000 ) ) ;
#74406=CARTESIAN_POINT ( 'NONE',  ( -2.294871794871793824, -4.000000000000000000, 29.75000000000000355 ) ) ;
#74407=ORIENTED_EDGE ( 'NONE', *, *, #16294, .T. ) ;
#74433=ADVANCED_FACE ( 'NONE', ( #5729 ), #81403, .T. ) ;
#74444=CARTESIAN_POINT ( 'NONE',  ( 8.352564102564102200, -7.500000000000000000, 29.75000000000000355 ) ) ;
#74455=DIRECTION ( 'NONE',  ( 0.000000000000000000, -1.000000000000000000, 0.000000000000000000 ) ) ;
#74495=DIRECTION ( 'NONE',  ( -0.000000000000000000, 1.000000000000000000, -0.000000000000000000 ) ) ;
#74507=ORIENTED_EDGE ( 'NONE', *, *, #6580, .T. ) ;
#74516=DIRECTION ( 'NONE',  ( -1.000000000000000000, -0.000000000000000000, 0.000000000000000000 ) ) ;
#74520=VECTOR ( 'NONE', #11835, 1000.000000000000000 ) ;
#74529=LINE ( 'NONE', #68216, #41145 ) ;
#74532=FACE_OUTER_BOUND ( 'NONE', #10623, .T. ) ;
#74539=VECTOR ( 'NONE', #80237, 1000.000000000000000 ) ;
#74546=AXIS2_PLACEMENT_3D ( 'NONE', #17035, #64764, #58019 ) ;
#74556=DIRECTION ( 'NONE',  ( 0.000000000000000000, 0.000000000000000000, -1.000000000000000000 ) ) ;
#74558=VECTOR ( 'NONE', #6912, 1000.000000000000000 ) ;
#74565=AXIS2_PLACEMENT_3D ( 'NONE', #69334, #84188, #49930 ) ;
#74574=CIRCLE ( 'NONE', #75980, 4.000000000000000000 ) ;
#74582=CYLINDRICAL_SURFACE ( 'NONE', #57770, 4.000000000000000000 ) ;
#74596=PLANE ( 'NONE',  #23114 ) ;
#74609=DIRECTION ( 'NONE',  ( 1.000000000000000000, 0.000000000000000000, 0.000000000000000000 ) ) ;
#74615=EDGE_CURVE ( 'NONE', #27642, #52479, #29553, .T. ) ;
#74633=VERTEX_POINT ( 'NONE', #43060 ) ;
#74634=LINE ( 'NONE', #67872, #50011 ) ;
#74652=VERTEX_POINT ( 'NONE', #65540 ) ;
#74673=CARTESIAN_POINT ( 'NONE',  ( 7.384615384615385025, -7.500000000000000000, 29.75000000000000355 ) ) ;
#74675=ORIENTED_EDGE ( 'NONE', *, *, #29458, .F. ) ;
#74694=CARTESIAN_POINT ( 'NONE',  ( -18.75000000000000000, -11.00000000000000000, 29.75000000000000355 ) ) ;
#74697=DIRECTION ( 'NONE',  ( -1.000000000000000000, -0.000000000000000000, -0.000000000000000000 ) ) ;
#74702=ORIENTED_EDGE ( 'NONE', *, *, #72858, .T. ) ;
#74704=CARTESIAN_POINT ( 'NONE',  ( 6.166666666666664298, -7.500000000000000000, 29.75000000000000355 ) ) ;
#74706=VECTOR ( 'NONE', #53009, 1000.000000000000000 ) ;
#74713=EDGE_CURVE ( 'NONE', #79996, #76951, #80863, .T. ) ;
#74737=ADVANCED_FACE ( 'NONE', ( #72740 ), #80410, .F. ) ;
#74740=CARTESIAN_POINT ( 'NONE',  ( 7.134615384615385025, -11.00000000000000000, 29.75000000000000355 ) ) ;
#74747=CARTESIAN_POINT ( 'NONE',  ( -9.320512820512821150, -11.00000000000000000, 28.25000000000000000 ) ) ;
#74760=ORIENTED_EDGE ( 'NONE', *, *, #79079, .T. ) ;
#74774=AXIS2_PLACEMENT_3D ( 'NONE', #67848, #40390, #19222 ) ;
#74809=DIRECTION ( 'NONE',  ( -1.000000000000000000, -0.000000000000000000, -0.000000000000000000 ) ) ;
#74811=DIRECTION ( 'NONE',  ( -1.000000000000000000, -0.000000000000000000, -0.000000000000000000 ) ) ;
#74824=VECTOR ( 'NONE', #4936, 1000.000000000000000 ) ;
#74848=DIRECTION ( 'NONE',  ( -0.000000000000000000, 1.000000000000000000, -0.000000000000000000 ) ) ;
#74851=VERTEX_POINT ( 'NONE', #54243 ) ;
#74856=ORIENTED_EDGE ( 'NONE', *, *, #84704, .T. ) ;
#74858=LINE ( 'NONE', #11820, #58403 ) ;
#74867=VECTOR ( 'NONE', #82500, 1000.000000000000000 ) ;
#74875=LINE ( 'NONE', #73985, #59143 ) ;
#74877=CARTESIAN_POINT ( 'NONE',  ( 5.198717948717946236, -11.50000000000000000, 29.75000000000000355 ) ) ;
#74879=CARTESIAN_POINT ( 'NONE',  ( 11.00641025641025550, -11.50000000000000000, 29.75000000000000355 ) ) ;
#74887=CARTESIAN_POINT ( 'NONE',  ( -15.84615384615384670, -7.500000000000000000, 29.75000000000000355 ) ) ;
#74893=ORIENTED_EDGE ( 'NONE', *, *, #23999, .F. ) ;
#74898=CARTESIAN_POINT ( 'NONE',  ( -7.384615384615385025, -3.499999999999999556, 29.75000000000000355 ) ) ;
#74906=CARTESIAN_POINT ( 'NONE',  ( -11.25641025641025550, -7.500000000000000000, 29.75000000000000355 ) ) ;
#74913=CARTESIAN_POINT ( 'NONE',  ( -10.03846153846153832, -3.499999999999999556, 29.75000000000000355 ) ) ;
#74941=ORIENTED_EDGE ( 'NONE', *, *, #67812, .F. ) ;
#74950=CARTESIAN_POINT ( 'NONE',  ( -19.50000000000000000, -11.50000000000000000, 29.75000000000000355 ) ) ;
#74951=FACE_OUTER_BOUND ( 'NONE', #34264, .T. ) ;
#74984=VECTOR ( 'NONE', #66217, 1000.000000000000000 ) ;
#74999=ORIENTED_EDGE ( 'NONE', *, *, #38209, .F. ) ;
#75009=LINE ( 'NONE', #25923, #12001 ) ;
#75015=ORIENTED_EDGE ( 'NONE', *, *, #69496, .T. ) ;
#75032=CARTESIAN_POINT ( 'NONE',  ( 14.87820512820512953, -3.499999999999999556, 29.75000000000000355 ) ) ;
#75080=VERTEX_POINT ( 'NONE', #87513 ) ;
#75084=EDGE_LOOP ( 'NONE', ( #33458, #61548, #15828, #63464 ) ) ;
#75087=VECTOR ( 'NONE', #70967, 1000.000000000000000 ) ;
#75093=ORIENTED_EDGE ( 'NONE', *, *, #87924, .T. ) ;
#75094=EDGE_LOOP ( 'NONE', ( #18619, #16314, #8970, #6707 ) ) ;
#75095=VERTEX_POINT ( 'NONE', #52359 ) ;
#75121=ORIENTED_EDGE ( 'NONE', *, *, #63219, .T. ) ;
#75128=ORIENTED_EDGE ( 'NONE', *, *, #15460, .F. ) ;
#75136=AXIS2_PLACEMENT_3D ( 'NONE', #56974, #16003, #35377 ) ;
#75143=ORIENTED_EDGE ( 'NONE', *, *, #28727, .F. ) ;
#75181=EDGE_CURVE ( 'NONE', #9891, #67129, #7010, .T. ) ;
#75186=FACE_OUTER_BOUND ( 'NONE', #17727, .T. ) ;
#75198=LINE ( 'NONE', #61661, #8957 ) ;
#75220=FACE_OUTER_BOUND ( 'NONE', #15298, .T. ) ;
#75221=ORIENTED_EDGE ( 'NONE', *, *, #39651, .T. ) ;
#75224=ORIENTED_EDGE ( 'NONE', *, *, #84059, .F. ) ;
#75228=VECTOR ( 'NONE', #29545, 1000.000000000000000 ) ;
#75229=VERTEX_POINT ( 'NONE', #67830 ) ;
#75231=ORIENTED_EDGE ( 'NONE', *, *, #79981, .T. ) ;
#75250=CARTESIAN_POINT ( 'NONE',  ( -2.544871794871794268, -11.00000000000000000, 29.75000000000000355 ) ) ;
#75251=CARTESIAN_POINT ( 'NONE',  ( -11.97435897435897267, -7.500000000000000000, 33.75000000000000000 ) ) ;
#75258=ORIENTED_EDGE ( 'NONE', *, *, #51565, .T. ) ;
#75263=AXIS2_PLACEMENT_3D ( 'NONE', #47178, #82317, #61135 ) ;
#75266=ORIENTED_EDGE ( 'NONE', *, *, #2608, .T. ) ;
#75267=CARTESIAN_POINT ( 'NONE',  ( -0.3589743589743593088, -7.500000000000000000, 29.75000000000000355 ) ) ;
#75271=FACE_OUTER_BOUND ( 'NONE', #1057, .T. ) ;
#75273=ADVANCED_FACE ( 'NONE', ( #36268 ), #84022, .F. ) ;
#75277=DIRECTION ( 'NONE',  ( 1.000000000000000000, 0.000000000000000000, 0.000000000000000000 ) ) ;
#75283=DIRECTION ( 'NONE',  ( -1.000000000000000000, 0.000000000000000000, 0.000000000000000000 ) ) ;
#75291=EDGE_LOOP ( 'NONE', ( #23572, #5630, #17791, #49916 ) ) ;
#75295=AXIS2_PLACEMENT_3D ( 'NONE', #3004, #23282, #57070 ) ;
#75317=ADVANCED_FACE ( 'NONE', ( #63280 ), #63721, .T. ) ;
#75323=AXIS2_PLACEMENT_3D ( 'NONE', #25375, #66808, #73120 ) ;
#75324=CYLINDRICAL_SURFACE ( 'NONE', #84736, 4.000000000000000000 ) ;
#75325=CARTESIAN_POINT ( 'NONE',  ( 19.00000000000000000, -7.500000000000000000, 29.75000000000000355 ) ) ;
#75327=ADVANCED_FACE ( 'NONE', ( #69161 ), #50195, .F. ) ;
#75344=DIRECTION ( 'NONE',  ( 0.000000000000000000, 0.000000000000000000, -1.000000000000000000 ) ) ;
#75345=VERTEX_POINT ( 'NONE', #31576 ) ;
#75352=DIRECTION ( 'NONE',  ( -0.000000000000000000, 1.000000000000000000, -0.000000000000000000 ) ) ;
#75357=FACE_OUTER_BOUND ( 'NONE', #63484, .T. ) ;
#75358=DIRECTION ( 'NONE',  ( 1.000000000000000000, 0.000000000000000000, 0.000000000000000000 ) ) ;
#75376=CARTESIAN_POINT ( 'NONE',  ( 19.00000000000000000, -3.499999999999999556, 29.75000000000000355 ) ) ;
#75383=CYLINDRICAL_SURFACE ( 'NONE', #21766, 4.000000000000000000 ) ;
#75384=AXIS2_PLACEMENT_3D ( 'NONE', #88104, #74556, #13736 ) ;
#75406=CARTESIAN_POINT ( 'NONE',  ( 2.544871794871792936, -11.00000000000000000, 29.75000000000000355 ) ) ;
#75410=VERTEX_POINT ( 'NONE', #65359 ) ;
#75415=ADVANCED_FACE ( 'NONE', ( #58593 ), #25268, .F. ) ;
#75417=DIRECTION ( 'NONE',  ( -0.000000000000000000, 0.000000000000000000, 1.000000000000000000 ) ) ;
#75418=DIRECTION ( 'NONE',  ( -1.000000000000000000, -0.000000000000000000, 0.000000000000000000 ) ) ;
#75432=ORIENTED_EDGE ( 'NONE', *, *, #27657, .T. ) ;
#75440=AXIS2_PLACEMENT_3D ( 'NONE', #13941, #41420, #81979 ) ;
#75441=VECTOR ( 'NONE', #33947, 1000.000000000000000 ) ;
#75455=ORIENTED_EDGE ( 'NONE', *, *, #85238, .F. ) ;
#75456=LINE ( 'NONE', #6998, #6792 ) ;
#75460=ORIENTED_EDGE ( 'NONE', *, *, #80765, .T. ) ;
#75465=VECTOR ( 'NONE', #63639, 1000.000000000000000 ) ;
#75494=DIRECTION ( 'NONE',  ( 0.000000000000000000, 0.000000000000000000, -1.000000000000000000 ) ) ;
#75496=PLANE ( 'NONE',  #87189 ) ;
#75497=ADVANCED_FACE ( 'NONE', ( #86087 ), #66699, .T. ) ;
#75500=DIRECTION ( 'NONE',  ( 1.000000000000000000, 0.000000000000000000, 0.000000000000000000 ) ) ;
#75503=CARTESIAN_POINT ( 'NONE',  ( -19.50000000000000000, -3.499999999999999556, 29.75000000000000355 ) ) ;
#75508=CARTESIAN_POINT ( 'NONE',  ( -15.84615384615384670, -11.50000000000000000, 29.75000000000000355 ) ) ;
#75531=EDGE_CURVE ( 'NONE', #75080, #81881, #69364, .T. ) ;
#75532=ORIENTED_EDGE ( 'NONE', *, *, #28478, .T. ) ;
#75539=EDGE_CURVE ( 'NONE', #18250, #44505, #12646, .T. ) ;
#75546=CARTESIAN_POINT ( 'NONE',  ( -17.06410256410256565, -7.500000000000000000, 29.75000000000000355 ) ) ;
#75558=DIRECTION ( 'NONE',  ( -1.000000000000000000, -0.000000000000000000, -0.000000000000000000 ) ) ;
#75561=DIRECTION ( 'NONE',  ( -1.000000000000000000, -0.000000000000000000, 0.000000000000000000 ) ) ;
#75596=CARTESIAN_POINT ( 'NONE',  ( -6.166666666666667851, -3.499999999999999556, 29.75000000000000355 ) ) ;
#75597=DIRECTION ( 'NONE',  ( -1.000000000000000000, 0.000000000000000000, -0.000000000000000000 ) ) ;
#75604=PLANE ( 'NONE',  #48907 ) ;
#75617=DIRECTION ( 'NONE',  ( 1.000000000000000000, 0.000000000000000000, 0.000000000000000000 ) ) ;
#75621=PLANE ( 'NONE',  #88277 ) ;
#75622=VECTOR ( 'NONE', #77756, 1000.000000000000000 ) ;
#75640=VERTEX_POINT ( 'NONE', #9862 ) ;
#75643=VERTEX_POINT ( 'NONE', #2212 ) ;
#75646=EDGE_LOOP ( 'NONE', ( #79656, #42670, #79414, #28419 ) ) ;
#75648=ADVANCED_FACE ( 'NONE', ( #63021 ), #84656, .F. ) ;
#75655=CYLINDRICAL_SURFACE ( 'NONE', #81357, 4.000000000000000000 ) ;
#75661=ADVANCED_FACE ( 'NONE', ( #85530 ), #28826, .F. ) ;
#75669=LINE ( 'NONE', #77010, #35191 ) ;
#75682=VECTOR ( 'NONE', #19439, 1000.000000000000000 ) ;
#75690=ORIENTED_EDGE ( 'NONE', *, *, #11400, .F. ) ;
#75691=EDGE_CURVE ( 'NONE', #61882, #6628, #66133, .T. ) ;
#75699=EDGE_CURVE ( 'NONE', #87211, #53945, #51257, .T. ) ;
#75709=PLANE ( 'NONE',  #54804 ) ;
#75718=EDGE_LOOP ( 'NONE', ( #27765, #84171, #9959, #885 ) ) ;
#75727=ORIENTED_EDGE ( 'NONE', *, *, #43683, .F. ) ;
#75744=AXIS2_PLACEMENT_3D ( 'NONE', #39740, #61754, #19893 ) ;
#75745=ADVANCED_FACE ( 'NONE', ( #24251 ), #25155, .T. ) ;
#75750=ADVANCED_FACE ( 'NONE', ( #73348 ), #17963, .F. ) ;
#75765=PLANE ( 'NONE',  #33904 ) ;
#75770=AXIS2_PLACEMENT_3D ( 'NONE', #73202, #38981, #31775 ) ;
#75778=LINE ( 'NONE', #573, #45948 ) ;
#75781=CARTESIAN_POINT ( 'NONE',  ( 19.00000000000000000, -11.50000000000000000, 29.75000000000000355 ) ) ;
#75785=EDGE_LOOP ( 'NONE', ( #77210, #49453, #36548, #11960 ) ) ;
#75800=CARTESIAN_POINT ( 'NONE',  ( -16.09615384615384670, -7.500000000000000000, 29.75000000000000355 ) ) ;
#75814=LINE ( 'NONE', #12348, #74558 ) ;
#75823=VERTEX_POINT ( 'NONE', #82778 ) ;
#75824=VECTOR ( 'NONE', #34006, 1000.000000000000000 ) ;
#75835=CARTESIAN_POINT ( 'NONE',  ( 16.09615384615384670, -7.500000000000000000, 29.75000000000000355 ) ) ;
#75843=EDGE_CURVE ( 'NONE', #31043, #23382, #88223, .T. ) ;
#75863=DIRECTION ( 'NONE',  ( 1.000000000000000000, 0.000000000000000000, 0.000000000000000000 ) ) ;
#75884=CARTESIAN_POINT ( 'NONE',  ( -18.75000000000000000, -3.499999999999999556, 29.75000000000000355 ) ) ;
#75895=ORIENTED_EDGE ( 'NONE', *, *, #73380, .T. ) ;
#75898=DIRECTION ( 'NONE',  ( -0.000000000000000000, 1.000000000000000000, -0.000000000000000000 ) ) ;
#75930=DIRECTION ( 'NONE',  ( -0.000000000000000000, 1.000000000000000000, -0.000000000000000000 ) ) ;
#75945=DIRECTION ( 'NONE',  ( 1.000000000000000000, 0.000000000000000000, 0.000000000000000000 ) ) ;
#75955=DIRECTION ( 'NONE',  ( 0.000000000000000000, 0.000000000000000000, -1.000000000000000000 ) ) ;
#75963=AXIS2_PLACEMENT_3D ( 'NONE', #56683, #75617, #55350 ) ;
#75968=ORIENTED_EDGE ( 'NONE', *, *, #15358, .T. ) ;
#75972=DIRECTION ( 'NONE',  ( -1.000000000000000000, -0.000000000000000000, -0.000000000000000000 ) ) ;
#75980=AXIS2_PLACEMENT_3D ( 'NONE', #80692, #39253, #13542 ) ;
#75983=ORIENTED_EDGE ( 'NONE', *, *, #55445, .F. ) ;
#75989=ORIENTED_EDGE ( 'NONE', *, *, #26894, .F. ) ;
#75992=FACE_OUTER_BOUND ( 'NONE', #13953, .T. ) ;
#75993=LINE ( 'NONE', #26042, #54562 ) ;
#76010=CARTESIAN_POINT ( 'NONE',  ( 2.544871794871792936, -7.500000000000000000, 33.75000000000000000 ) ) ;
#76013=PRESENTATION_STYLE_ASSIGNMENT (( #48530 ) ) ;
#76027=DIRECTION ( 'NONE',  ( 1.000000000000000000, 0.000000000000000000, 0.000000000000000000 ) ) ;
#76043=DIRECTION ( 'NONE',  ( 0.000000000000000000, 0.000000000000000000, -1.000000000000000000 ) ) ;
#76050=PLANE ( 'NONE',  #2513 ) ;
#76057=CYLINDRICAL_SURFACE ( 'NONE', #58888, 4.000000000000000000 ) ;
#76073=ORIENTED_EDGE ( 'NONE', *, *, #69946, .F. ) ;
#76079=DIRECTION ( 'NONE',  ( 0.000000000000000000, 0.000000000000000000, -1.000000000000000000 ) ) ;
#76097=AXIS2_PLACEMENT_3D ( 'NONE', #74444, #60922, #39344 ) ;
#76104=VECTOR ( 'NONE', #36823, 1000.000000000000000 ) ;
#76117=EDGE_CURVE ( 'NONE', #79307, #7973, #32694, .T. ) ;
#76127=DIRECTION ( 'NONE',  ( -1.000000000000000000, -0.000000000000000000, -0.000000000000000000 ) ) ;
#76135=EDGE_CURVE ( 'NONE', #18077, #24532, #45765, .T. ) ;
#76139=DIRECTION ( 'NONE',  ( 1.000000000000000000, 0.000000000000000000, 0.000000000000000000 ) ) ;
#76143=ORIENTED_EDGE ( 'NONE', *, *, #23648, .F. ) ;
#76155=ADVANCED_FACE ( 'NONE', ( #31365 ), #58828, .F. ) ;
#76166=ORIENTED_EDGE ( 'NONE', *, *, #14653, .F. ) ;
#76176=CARTESIAN_POINT ( 'NONE',  ( -18.75000000000000000, -7.500000000000000000, 29.75000000000000355 ) ) ;
#76179=CARTESIAN_POINT ( 'NONE',  ( 11.25641025641025550, -3.499999999999999556, 29.75000000000000355 ) ) ;
#76189=EDGE_CURVE ( 'NONE', #20882, #31226, #53855, .T. ) ;
#76194=EDGE_CURVE ( 'NONE', #38776, #18719, #88119, .T. ) ;
#76199=DIRECTION ( 'NONE',  ( 0.000000000000000000, 0.000000000000000000, -1.000000000000000000 ) ) ;
#76230=DIRECTION ( 'NONE',  ( -0.000000000000000000, 1.000000000000000000, -0.000000000000000000 ) ) ;
#76240=ORIENTED_EDGE ( 'NONE', *, *, #34738, .F. ) ;
#76248=DIRECTION ( 'NONE',  ( -0.000000000000000000, 1.000000000000000000, -0.000000000000000000 ) ) ;
#76266=EDGE_CURVE ( 'NONE', #67618, #27341, #75456, .T. ) ;
#76267=ORIENTED_EDGE ( 'NONE', *, *, #83652, .F. ) ;
#76269=EDGE_CURVE ( 'NONE', #86305, #43735, #82674, .T. ) ;
#76275=CARTESIAN_POINT ( 'NONE',  ( -9.070512820512819374, -11.00000000000000000, 29.75000000000000355 ) ) ;
#76297=AXIS2_PLACEMENT_3D ( 'NONE', #78221, #37681, #70589 ) ;
#76321=DIRECTION ( 'NONE',  ( -1.000000000000000000, -0.000000000000000000, -0.000000000000000000 ) ) ;
#76322=CARTESIAN_POINT ( 'NONE',  ( 0.000000000000000000, -11.00000000000000000, 29.75000000000000355 ) ) ;
#76327=DIRECTION ( 'NONE',  ( -1.000000000000000000, 0.000000000000000000, -0.000000000000000000 ) ) ;
#76338=EDGE_LOOP ( 'NONE', ( #40790, #44650, #29683, #50273 ) ) ;
#76341=CIRCLE ( 'NONE', #24585, 4.000000000000000000 ) ;
#76343=EDGE_LOOP ( 'NONE', ( #53914, #68793, #6794, #66894 ) ) ;
#76344=DIRECTION ( 'NONE',  ( 1.000000000000000000, 0.000000000000000000, 0.000000000000000000 ) ) ;
#76355=LINE ( 'NONE', #2027, #58729 ) ;
#76371=ORIENTED_EDGE ( 'NONE', *, *, #6990, .T. ) ;
#76379=CARTESIAN_POINT ( 'NONE',  ( 20.00000000000000000, -4.000000000000000000, 29.75000000000000355 ) ) ;
#76391=VECTOR ( 'NONE', #28053, 1000.000000000000000 ) ;
#76393=LINE ( 'NONE', #28656, #83856 ) ;
#76405=EDGE_CURVE ( 'NONE', #83780, #67446, #47163, .T. ) ;
#76413=ORIENTED_EDGE ( 'NONE', *, *, #50357, .F. ) ;
#76420=DIRECTION ( 'NONE',  ( -1.000000000000000000, 0.000000000000000000, -0.000000000000000000 ) ) ;
#76424=ORIENTED_EDGE ( 'NONE', *, *, #8813, .F. ) ;
#76440=ORIENTED_EDGE ( 'NONE', *, *, #81198, .T. ) ;
#76441=CYLINDRICAL_SURFACE ( 'NONE', #24584, 4.000000000000000000 ) ;
#76446=VECTOR ( 'NONE', #74809, 1000.000000000000000 ) ;
#76453=CARTESIAN_POINT ( 'NONE',  ( -1.576923076923076872, -3.499999999999999556, 29.75000000000000355 ) ) ;
#76454=LINE ( 'NONE', #63367, #56919 ) ;
#76484=VECTOR ( 'NONE', #686, 1000.000000000000000 ) ;
#76486=DIRECTION ( 'NONE',  ( 1.000000000000000000, 0.000000000000000000, 0.000000000000000000 ) ) ;
#76500=CARTESIAN_POINT ( 'NONE',  ( -11.00641025641025550, -3.499999999999999556, 29.75000000000000355 ) ) ;
#76518=EDGE_CURVE ( 'NONE', #50090, #79307, #23605, .T. ) ;
#76525=AXIS2_PLACEMENT_3D ( 'NONE', #70075, #75500, #43049 ) ;
#76526=ORIENTED_EDGE ( 'NONE', *, *, #77177, .T. ) ;
#76550=VECTOR ( 'NONE', #15494, 1000.000000000000000 ) ;
#76565=CARTESIAN_POINT ( 'NONE',  ( -14.16025641025641058, -11.50000000000000000, 29.75000000000000355 ) ) ;
#76572=DIRECTION ( 'NONE',  ( -0.000000000000000000, 1.000000000000000000, -0.000000000000000000 ) ) ;
#76573=CARTESIAN_POINT ( 'NONE',  ( -19.50000000000000000, -3.499999999999999556, 29.75000000000000355 ) ) ;
#76587=LINE ( 'NONE', #13224, #85353 ) ;
#76592=ORIENTED_EDGE ( 'NONE', *, *, #3302, .F. ) ;
#76602=ORIENTED_EDGE ( 'NONE', *, *, #48944, .T. ) ;
#76636=ORIENTED_EDGE ( 'NONE', *, *, #67795, .T. ) ;
#76637=EDGE_CURVE ( 'NONE', #49175, #83716, #68158, .T. ) ;
#76651=CARTESIAN_POINT ( 'NONE',  ( 20.00000000000000000, -3.499999999999999556, 29.75000000000000355 ) ) ;
#76666=AXIS2_PLACEMENT_3D ( 'NONE', #21850, #63715, #49758 ) ;
#76667=CARTESIAN_POINT ( 'NONE',  ( -10.03846153846153832, -4.000000000000000000, 29.75000000000000355 ) ) ;
#76670=EDGE_CURVE ( 'NONE', #38958, #27134, #83904, .T. ) ;
#76673=ORIENTED_EDGE ( 'NONE', *, *, #68415, .T. ) ;
#76678=DIRECTION ( 'NONE',  ( 1.000000000000000000, 0.000000000000000000, 0.000000000000000000 ) ) ;
#76681=CARTESIAN_POINT ( 'NONE',  ( -14.87820512820512953, -11.00000000000000000, 29.75000000000000355 ) ) ;
#76686=LINE ( 'NONE', #28958, #54555 ) ;
#76696=VERTEX_POINT ( 'NONE', #28503 ) ;
#76710=DIRECTION ( 'NONE',  ( -1.000000000000000000, -0.000000000000000000, 0.000000000000000000 ) ) ;
#76715=DIRECTION ( 'NONE',  ( 1.000000000000000000, 0.000000000000000000, 0.000000000000000000 ) ) ;
#76719=DIRECTION ( 'NONE',  ( -1.000000000000000000, 0.000000000000000000, -0.000000000000000000 ) ) ;
#76734=VECTOR ( 'NONE', #20920, 1000.000000000000000 ) ;
#76738=VECTOR ( 'NONE', #6402, 1000.000000000000000 ) ;
#76742=EDGE_LOOP ( 'NONE', ( #63085, #24039, #4568, #77216, #34400 ) ) ;
#76762=EDGE_CURVE ( 'NONE', #30312, #3756, #12557, .T. ) ;
#76769=ADVANCED_FACE ( 'NONE', ( #12121 ), #26070, .F. ) ;
#76772=DIRECTION ( 'NONE',  ( -1.000000000000000000, -0.000000000000000000, -0.000000000000000000 ) ) ;
#76783=ORIENTED_EDGE ( 'NONE', *, *, #65454, .T. ) ;
#76785=DIRECTION ( 'NONE',  ( 1.000000000000000000, 0.000000000000000000, 0.000000000000000000 ) ) ;
#76791=ADVANCED_FACE ( 'NONE', ( #38691 ), #4456, .F. ) ;
#76800=ORIENTED_EDGE ( 'NONE', *, *, #6773, .T. ) ;
#76801=EDGE_CURVE ( 'NONE', #51205, #30150, #40043, .T. ) ;
#76816=DIRECTION ( 'NONE',  ( 1.000000000000000000, 0.000000000000000000, 0.000000000000000000 ) ) ;
#76817=CARTESIAN_POINT ( 'NONE',  ( -1.326923076923076872, -11.50000000000000000, 29.75000000000000355 ) ) ;
#76840=LINE ( 'NONE', #52008, #35806 ) ;
#76844=DIRECTION ( 'NONE',  ( -0.000000000000000000, 1.000000000000000000, -0.000000000000000000 ) ) ;
#76846=CARTESIAN_POINT ( 'NONE',  ( 9.320512820512821150, -11.00000000000000000, 29.25000000000000000 ) ) ;
#76854=EDGE_CURVE ( 'NONE', #33955, #85035, #39602, .T. ) ;
#76858=LINE ( 'NONE', #86175, #45155 ) ;
#76860=ORIENTED_EDGE ( 'NONE', *, *, #45447, .T. ) ;
#76861=ORIENTED_EDGE ( 'NONE', *, *, #30271, .T. ) ;
#76863=VECTOR ( 'NONE', #73394, 1000.000000000000000 ) ;
#76866=CARTESIAN_POINT ( 'NONE',  ( 16.09615384615384670, -7.500000000000000000, 33.75000000000000000 ) ) ;
#76872=ORIENTED_EDGE ( 'NONE', *, *, #61975, .F. ) ;
#76875=ORIENTED_EDGE ( 'NONE', *, *, #56827, .F. ) ;
#76880=LINE ( 'NONE', #23586, #41063 ) ;
#76884=AXIS2_PLACEMENT_3D ( 'NONE', #82706, #54769, #1944 ) ;
#76891=DIRECTION ( 'NONE',  ( 0.000000000000000000, 0.000000000000000000, -1.000000000000000000 ) ) ;
#76897=ORIENTED_EDGE ( 'NONE', *, *, #25064, .T. ) ;
#76913=ORIENTED_EDGE ( 'NONE', *, *, #13634, .T. ) ;
#76919=LINE ( 'NONE', #78687, #27301 ) ;
#76927=VERTEX_POINT ( 'NONE', #28274 ) ;
#76951=VERTEX_POINT ( 'NONE', #61169 ) ;
#76961=AXIS2_PLACEMENT_3D ( 'NONE', #73798, #72440, #18844 ) ;
#76973=ORIENTED_EDGE ( 'NONE', *, *, #79424, .F. ) ;
#77003=EDGE_CURVE ( 'NONE', #12230, #35283, #35480, .T. ) ;
#77010=CARTESIAN_POINT ( 'NONE',  ( 0.000000000000000000, -11.00000000000000000, 29.75000000000000355 ) ) ;
#77014=ORIENTED_EDGE ( 'NONE', *, *, #51244, .F. ) ;
#77023=CARTESIAN_POINT ( 'NONE',  ( 20.00000000000000000, -4.000000000000000000, 29.75000000000000355 ) ) ;
#77040=CARTESIAN_POINT ( 'NONE',  ( -16.81410256410256565, -7.500000000000000000, 29.75000000000000355 ) ) ;
#77043=CARTESIAN_POINT ( 'NONE',  ( 8.352564102564102200, -3.499999999999999556, 29.75000000000000355 ) ) ;
#77053=AXIS2_PLACEMENT_3D ( 'NONE', #64714, #85010, #79583 ) ;
#77058=CARTESIAN_POINT ( 'NONE',  ( -13.91025641025641058, -7.500000000000000000, 33.75000000000000000 ) ) ;
#77065=CIRCLE ( 'NONE', #18105, 4.000000000000000000 ) ;
#77066=ORIENTED_EDGE ( 'NONE', *, *, #76117, .T. ) ;
#77070=CARTESIAN_POINT ( 'NONE',  ( 8.102564102564102200, -3.499999999999999556, 29.75000000000000355 ) ) ;
#77071=ADVANCED_FACE ( 'NONE', ( #58389 ), #17427, .F. ) ;
#77075=ORIENTED_EDGE ( 'NONE', *, *, #1553, .F. ) ;
#77077=ORIENTED_EDGE ( 'NONE', *, *, #80762, .F. ) ;
#77078=CARTESIAN_POINT ( 'NONE',  ( -19.50000000000000000, -3.499999999999999556, 29.75000000000000355 ) ) ;
#77088=VERTEX_POINT ( 'NONE', #24621 ) ;
#77095=DIRECTION ( 'NONE',  ( 0.000000000000000000, 0.000000000000000000, 1.000000000000000000 ) ) ;
#77101=CIRCLE ( 'NONE', #25349, 4.000000000000000000 ) ;
#77120=LINE ( 'NONE', #43335, #9202 ) ;
#77139=CYLINDRICAL_SURFACE ( 'NONE', #53683, 4.000000000000000000 ) ;
#77142=DIRECTION ( 'NONE',  ( 0.000000000000000000, 1.000000000000000000, 0.000000000000000000 ) ) ;
#77146=ORIENTED_EDGE ( 'NONE', *, *, #54841, .T. ) ;
#77154=DIRECTION ( 'NONE',  ( 1.000000000000000000, 0.000000000000000000, 0.000000000000000000 ) ) ;
#77163=ORIENTED_EDGE ( 'NONE', *, *, #51180, .T. ) ;
#77171=VECTOR ( 'NONE', #64507, 1000.000000000000000 ) ;
#77177=EDGE_CURVE ( 'NONE', #77909, #30104, #11109, .T. ) ;
#77179=ORIENTED_EDGE ( 'NONE', *, *, #34553, .T. ) ;
#77180=EDGE_CURVE ( 'NONE', #75643, #53841, #31380, .T. ) ;
#77200=ORIENTED_EDGE ( 'NONE', *, *, #63159, .F. ) ;
#77201=ADVANCED_FACE ( 'NONE', ( #18315 ), #71916, .T. ) ;
#77206=CARTESIAN_POINT ( 'NONE',  ( -13.19230769230769162, -3.499999999999999556, 29.75000000000000355 ) ) ;
#77209=CARTESIAN_POINT ( 'NONE',  ( 8.102564102564102200, -3.499999999999999556, 29.75000000000000355 ) ) ;
#77210=ORIENTED_EDGE ( 'NONE', *, *, #22463, .F. ) ;
#77216=ORIENTED_EDGE ( 'NONE', *, *, #11928, .T. ) ;
#77219=CIRCLE ( 'NONE', #57101, 4.000000000000000000 ) ;
#77224=VECTOR ( 'NONE', #63336, 1000.000000000000000 ) ;
#77225=ORIENTED_EDGE ( 'NONE', *, *, #3448, .T. ) ;
#77227=CARTESIAN_POINT ( 'NONE',  ( 20.00000000000000000, -4.000000000000000000, 29.75000000000000355 ) ) ;
#77230=ORIENTED_EDGE ( 'NONE', *, *, #1614, .F. ) ;
#77243=DIRECTION ( 'NONE',  ( 0.000000000000000000, 0.000000000000000000, 1.000000000000000000 ) ) ;
#77262=EDGE_CURVE ( 'NONE', #15822, #37401, #61562, .T. ) ;
#77290=PLANE ( 'NONE',  #4641 ) ;
#77291=CIRCLE ( 'NONE', #16919, 4.000000000000000000 ) ;
#77299=VECTOR ( 'NONE', #4157, 1000.000000000000000 ) ;
#77305=ORIENTED_EDGE ( 'NONE', *, *, #69845, .T. ) ;
#77309=ORIENTED_EDGE ( 'NONE', *, *, #45497, .F. ) ;
#77310=DIRECTION ( 'NONE',  ( 0.000000000000000000, 0.000000000000000000, -1.000000000000000000 ) ) ;
#77316=CYLINDRICAL_SURFACE ( 'NONE', #23429, 4.000000000000000000 ) ;
#77328=ORIENTED_EDGE ( 'NONE', *, *, #33865, .T. ) ;
#77331=DIRECTION ( 'NONE',  ( 1.000000000000000000, 0.000000000000000000, 0.000000000000000000 ) ) ;
#77335=DIRECTION ( 'NONE',  ( -1.000000000000000000, -0.000000000000000000, -0.000000000000000000 ) ) ;
#77340=CARTESIAN_POINT ( 'NONE',  ( -19.50000000000000000, -11.50000000000000000, 29.75000000000000355 ) ) ;
#77346=ADVANCED_FACE ( 'NONE', ( #64600 ), #16432, .F. ) ;
#77348=LINE ( 'NONE', #43126, #78942 ) ;
#77350=DIRECTION ( 'NONE',  ( -1.000000000000000000, -0.000000000000000000, -0.000000000000000000 ) ) ;
#77380=FACE_OUTER_BOUND ( 'NONE', #28341, .T. ) ;
#77381=EDGE_LOOP ( 'NONE', ( #9435, #15380, #36565, #65536, #2530 ) ) ;
#77382=CARTESIAN_POINT ( 'NONE',  ( -1.576923076923076872, -7.500000000000000000, 29.75000000000000355 ) ) ;
#77385=ADVANCED_FACE ( 'NONE', ( #28624 ), #64157, .T. ) ;
#77399=CARTESIAN_POINT ( 'NONE',  ( 0.000000000000000000, -11.00000000000000000, 29.75000000000000355 ) ) ;
#77403=CARTESIAN_POINT ( 'NONE',  ( -8.102564102564102200, -11.50000000000000000, 29.75000000000000355 ) ) ;
#77405=CARTESIAN_POINT ( 'NONE',  ( -19.50000000000000000, -3.499999999999999556, 29.75000000000000355 ) ) ;
#77412=EDGE_CURVE ( 'NONE', #81637, #19931, #76355, .T. ) ;
#77416=VERTEX_POINT ( 'NONE', #9244 ) ;
#77417=ORIENTED_EDGE ( 'NONE', *, *, #84948, .F. ) ;
#77423=ORIENTED_EDGE ( 'NONE', *, *, #45232, .T. ) ;
#77434=EDGE_CURVE ( 'NONE', #34293, #77956, #84606, .T. ) ;
#77463=VECTOR ( 'NONE', #59507, 1000.000000000000000 ) ;
#77467=CARTESIAN_POINT ( 'NONE',  ( -17.78205128205128105, -7.500000000000000000, 29.75000000000000355 ) ) ;
#77470=ORIENTED_EDGE ( 'NONE', *, *, #30990, .F. ) ;
#77499=CARTESIAN_POINT ( 'NONE',  ( 17.78205128205128105, -7.500000000000000000, 33.75000000000000000 ) ) ;
#77500=EDGE_CURVE ( 'NONE', #50957, #64220, #44779, .T. ) ;
#77521=AXIS2_PLACEMENT_3D ( 'NONE', #67574, #54040, #26584 ) ;
#77534=DIRECTION ( 'NONE',  ( 0.000000000000000000, -0.000000000000000000, 1.000000000000000000 ) ) ;
#77540=EDGE_LOOP ( 'NONE', ( #2828, #85846, #4230, #57250 ) ) ;
#77541=CARTESIAN_POINT ( 'NONE',  ( 0.3589743589743586982, -4.000000000000000000, 29.75000000000000355 ) ) ;
#77565=EDGE_CURVE ( 'NONE', #81234, #73790, #75814, .T. ) ;
#77567=LINE ( 'NONE', #63154, #63001 ) ;
#77575=ORIENTED_EDGE ( 'NONE', *, *, #22949, .F. ) ;
#77591=FACE_OUTER_BOUND ( 'NONE', #70059, .T. ) ;
#77604=ORIENTED_EDGE ( 'NONE', *, *, #4959, .T. ) ;
#77610=DIRECTION ( 'NONE',  ( 1.000000000000000000, 0.000000000000000000, 0.000000000000000000 ) ) ;
#77619=VECTOR ( 'NONE', #82800, 1000.000000000000000 ) ;
#77636=AXIS2_PLACEMENT_3D ( 'NONE', #29190, #811, #47670 ) ;
#77670=EDGE_CURVE ( 'NONE', #7880, #77757, #15902, .T. ) ;
#77671=DIRECTION ( 'NONE',  ( 0.000000000000000000, 0.000000000000000000, -1.000000000000000000 ) ) ;
#77682=CARTESIAN_POINT ( 'NONE',  ( 0.000000000000000000, -11.50000000000000000, 29.25000000000000000 ) ) ;
#77688=AXIS2_PLACEMENT_3D ( 'NONE', #84555, #43111, #22393 ) ;
#77712=PLANE ( 'NONE',  #51577 ) ;
#77734=VECTOR ( 'NONE', #86822, 1000.000000000000000 ) ;
#77747=CIRCLE ( 'NONE', #46140, 4.000000000000000000 ) ;
#77751=CARTESIAN_POINT ( 'NONE',  ( -1.326923076923076872, -7.500000000000000000, 29.75000000000000355 ) ) ;
#77752=AXIS2_PLACEMENT_3D ( 'NONE', #75546, #28700, #29587 ) ;
#77756=DIRECTION ( 'NONE',  ( -1.000000000000000000, -0.000000000000000000, -0.000000000000000000 ) ) ;
#77757=VERTEX_POINT ( 'NONE', #22640 ) ;
#77771=EDGE_LOOP ( 'NONE', ( #12401, #43936, #54485, #31189, #29339 ) ) ;
#77774=CARTESIAN_POINT ( 'NONE',  ( -2.294871794871794712, -3.499999999999999556, 29.75000000000000355 ) ) ;
#77781=ORIENTED_EDGE ( 'NONE', *, *, #14015, .T. ) ;
#77787=CARTESIAN_POINT ( 'NONE',  ( -19.50000000000000000, -11.00000000000000000, 29.25000000000000000 ) ) ;
#77816=AXIS2_PLACEMENT_3D ( 'NONE', #77925, #78361, #51762 ) ;
#77841=PLANE ( 'NONE',  #29800 ) ;
#77873=FACE_OUTER_BOUND ( 'NONE', #71005, .T. ) ;
#77909=VERTEX_POINT ( 'NONE', #51410 ) ;
#77915=CARTESIAN_POINT ( 'NONE',  ( 20.00000000000000000, -4.000000000000000000, 29.75000000000000355 ) ) ;
#77925=CARTESIAN_POINT ( 'NONE',  ( -19.50000000000000000, -7.500000000000000000, 29.75000000000000355 ) ) ;
#77927=CARTESIAN_POINT ( 'NONE',  ( -15.12820512820512953, -7.500000000000000000, 29.75000000000000355 ) ) ;
#77956=VERTEX_POINT ( 'NONE', #66740 ) ;
#77964=CARTESIAN_POINT ( 'NONE',  ( -17.06410256410256565, -3.499999999999999556, 29.75000000000000355 ) ) ;
#77972=CYLINDRICAL_SURFACE ( 'NONE', #70323, 4.000000000000000000 ) ;
#77976=ORIENTED_EDGE ( 'NONE', *, *, #34995, .T. ) ;
#77990=CARTESIAN_POINT ( 'NONE',  ( -4.480769230769230838, -11.50000000000000000, 29.75000000000000355 ) ) ;
#78009=ORIENTED_EDGE ( 'NONE', *, *, #4735, .T. ) ;
#78017=DIRECTION ( 'NONE',  ( -1.000000000000000000, -0.000000000000000000, -0.000000000000000000 ) ) ;
#78024=ORIENTED_EDGE ( 'NONE', *, *, #34995, .F. ) ;
#78025=AXIS2_PLACEMENT_3D ( 'NONE', #12389, #81299, #68218 ) ;
#78032=CARTESIAN_POINT ( 'NONE',  ( 0.000000000000000000, -11.00000000000000000, 29.75000000000000355 ) ) ;
#78041=EDGE_LOOP ( 'NONE', ( #532, #32516, #38562, #63212 ) ) ;
#78047=LINE ( 'NONE', #70417, #25519 ) ;
#78061=DIRECTION ( 'NONE',  ( 1.000000000000000000, 0.000000000000000000, 0.000000000000000000 ) ) ;
#78074=EDGE_CURVE ( 'NONE', #85269, #59590, #34728, .T. ) ;
#78075=ORIENTED_EDGE ( 'NONE', *, *, #8573, .F. ) ;
#78082=DIRECTION ( 'NONE',  ( -0.000000000000000000, 1.000000000000000000, -0.000000000000000000 ) ) ;
#78092=LINE ( 'NONE', #77206, #66694 ) ;
#78101=ORIENTED_EDGE ( 'NONE', *, *, #72354, .F. ) ;
#78107=VECTOR ( 'NONE', #30661, 1000.000000000000000 ) ;
#78121=CARTESIAN_POINT ( 'NONE',  ( 1.326923076923075762, -7.500000000000000000, 29.75000000000000355 ) ) ;
#78124=EDGE_CURVE ( 'NONE', #949, #12463, #86143, .T. ) ;
#78126=DIRECTION ( 'NONE',  ( -1.000000000000000000, -0.000000000000000000, -0.000000000000000000 ) ) ;
#78128=DIRECTION ( 'NONE',  ( 0.000000000000000000, 0.000000000000000000, 1.000000000000000000 ) ) ;
#78142=AXIS2_PLACEMENT_3D ( 'NONE', #23335, #8067, #50358 ) ;
#78145=CARTESIAN_POINT ( 'NONE',  ( 17.06410256410256565, -11.00000000000000000, 29.75000000000000355 ) ) ;
#78150=CARTESIAN_POINT ( 'NONE',  ( -2.294871794871794712, -7.500000000000000000, 29.75000000000000355 ) ) ;
#78164=DIRECTION ( 'NONE',  ( 0.000000000000000000, 0.000000000000000000, 1.000000000000000000 ) ) ;
#78169=ORIENTED_EDGE ( 'NONE', *, *, #37835, .T. ) ;
#78177=CIRCLE ( 'NONE', #525, 4.000000000000000000 ) ;
#78179=ORIENTED_EDGE ( 'NONE', *, *, #22750, .T. ) ;
#78182=EDGE_LOOP ( 'NONE', ( #57392, #61862, #74856, #84601 ) ) ;
#78183=PLANE ( 'NONE',  #19146 ) ;
#78196=DIRECTION ( 'NONE',  ( 1.000000000000000000, 0.000000000000000000, 0.000000000000000000 ) ) ;
#78197=AXIS2_PLACEMENT_3D ( 'NONE', #58677, #37974, #24002 ) ;
#78204=ORIENTED_EDGE ( 'NONE', *, *, #44903, .F. ) ;
#78211=CARTESIAN_POINT ( 'NONE',  ( 17.06410256410256565, -3.499999999999999556, 29.75000000000000355 ) ) ;
#78221=CARTESIAN_POINT ( 'NONE',  ( 7.384615384615385025, -7.500000000000000000, 29.75000000000000355 ) ) ;
#78237=CARTESIAN_POINT ( 'NONE',  ( 18.75000000000000000, -11.50000000000000000, 29.75000000000000355 ) ) ;
#78255=AXIS2_PLACEMENT_3D ( 'NONE', #59047, #51371, #44183 ) ;
#78266=VERTEX_POINT ( 'NONE', #31512 ) ;
#78293=VERTEX_POINT ( 'NONE', #67527 ) ;
#78295=EDGE_LOOP ( 'NONE', ( #65358, #61261, #15249, #37108 ) ) ;
#78301=EDGE_LOOP ( 'NONE', ( #5582, #20631, #70608, #40643, #76371 ) ) ;
#78306=VECTOR ( 'NONE', #36029, 1000.000000000000000 ) ;
#78310=LINE ( 'NONE', #41549, #6284 ) ;
#78321=DIRECTION ( 'NONE',  ( -1.000000000000000000, -0.000000000000000000, -0.000000000000000000 ) ) ;
#78322=ORIENTED_EDGE ( 'NONE', *, *, #282, .T. ) ;
#78324=VERTEX_POINT ( 'NONE', #81494 ) ;
#78344=CARTESIAN_POINT ( 'NONE',  ( -10.28846153846153832, -3.499999999999999556, 29.75000000000000355 ) ) ;
#78353=AXIS2_PLACEMENT_3D ( 'NONE', #57091, #15235, #28750 ) ;
#78355=LINE ( 'NONE', #9033, #32907 ) ;
#78361=DIRECTION ( 'NONE',  ( 1.000000000000000000, 0.000000000000000000, 0.000000000000000000 ) ) ;
#78372=EDGE_CURVE ( 'NONE', #61830, #23542, #61628, .T. ) ;
#78379=ORIENTED_EDGE ( 'NONE', *, *, #52601, .T. ) ;
#78387=ORIENTED_EDGE ( 'NONE', *, *, #11555, .F. ) ;
#78389=VECTOR ( 'NONE', #78905, 1000.000000000000000 ) ;
#78393=ORIENTED_EDGE ( 'NONE', *, *, #71275, .T. ) ;
#78397=CARTESIAN_POINT ( 'NONE',  ( 8.102564102564102200, -3.499999999999999556, 29.75000000000000355 ) ) ;
#78432=CARTESIAN_POINT ( 'NONE',  ( -19.50000000000000000, -3.499999999999999556, 29.75000000000000355 ) ) ;
#78436=CARTESIAN_POINT ( 'NONE',  ( -7.384615384615385025, -3.499999999999999556, 29.75000000000000355 ) ) ;
#78468=DIRECTION ( 'NONE',  ( 1.000000000000000000, 0.000000000000000000, 0.000000000000000000 ) ) ;
#78478=VERTEX_POINT ( 'NONE', #70066 ) ;
#78486=DIRECTION ( 'NONE',  ( -0.000000000000000000, 0.000000000000000000, 1.000000000000000000 ) ) ;
#78495=CARTESIAN_POINT ( 'NONE',  ( -5.448717948717948012, -7.500000000000000000, 29.75000000000000355 ) ) ;
#78503=DIRECTION ( 'NONE',  ( -0.000000000000000000, 0.000000000000000000, 1.000000000000000000 ) ) ;
#78514=ORIENTED_EDGE ( 'NONE', *, *, #35986, .T. ) ;
#78516=CARTESIAN_POINT ( 'NONE',  ( -2.294871794871794712, -7.500000000000000000, 33.75000000000000000 ) ) ;
#78527=CARTESIAN_POINT ( 'NONE',  ( -6.166666666666667851, -3.499999999999999556, 29.75000000000000355 ) ) ;
#78538=CIRCLE ( 'NONE', #39744, 4.000000000000000000 ) ;
#78547=VERTEX_POINT ( 'NONE', #17798 ) ;
#78585=EDGE_LOOP ( 'NONE', ( #80508, #8715, #53381, #64463 ) ) ;
#78607=ORIENTED_EDGE ( 'NONE', *, *, #40740, .T. ) ;
#78616=EDGE_CURVE ( 'NONE', #19254, #49385, #12369, .T. ) ;
#78630=DIRECTION ( 'NONE',  ( 0.000000000000000000, 0.000000000000000000, 1.000000000000000000 ) ) ;
#78632=VECTOR ( 'NONE', #1397, 1000.000000000000000 ) ;
#78640=EDGE_CURVE ( 'NONE', #1333, #27068, #33960, .T. ) ;
#78643=CYLINDRICAL_SURFACE ( 'NONE', #13398, 4.000000000000000000 ) ;
#78647=ORIENTED_EDGE ( 'NONE', *, *, #36986, .T. ) ;
#78650=EDGE_LOOP ( 'NONE', ( #62836, #86591, #7532, #22678 ) ) ;
#78654=DIRECTION ( 'NONE',  ( -1.000000000000000000, -0.000000000000000000, -0.000000000000000000 ) ) ;
#78661=LINE ( 'NONE', #43542, #25602 ) ;
#78665=AXIS2_PLACEMENT_3D ( 'NONE', #29951, #7904, #7465 ) ;
#78670=( NAMED_UNIT ( * ) SI_UNIT ( $, .STERADIAN. ) SOLID_ANGLE_UNIT ( ) );
#78674=AXIS2_PLACEMENT_3D ( 'NONE', #15008, #83921, #6908 ) ;
#78682=EDGE_CURVE ( 'NONE', #75080, #69909, #53377, .T. ) ;
#78687=CARTESIAN_POINT ( 'NONE',  ( 20.00000000000000000, -4.000000000000000000, 29.75000000000000355 ) ) ;
#78691=CARTESIAN_POINT ( 'NONE',  ( 20.00000000000000000, -7.500000000000000000, 29.75000000000000355 ) ) ;
#78711=CARTESIAN_POINT ( 'NONE',  ( 7.134615384615385025, -11.50000000000000000, 29.75000000000000355 ) ) ;
#78715=VECTOR ( 'NONE', #69551, 1000.000000000000000 ) ;
#78732=CARTESIAN_POINT ( 'NONE',  ( 8.352564102564102200, -4.000000000000000000, 29.75000000000000355 ) ) ;
#78741=ORIENTED_EDGE ( 'NONE', *, *, #65420, .F. ) ;
#78753=ORIENTED_EDGE ( 'NONE', *, *, #50357, .T. ) ;
#78755=VECTOR ( 'NONE', #23492, 1000.000000000000000 ) ;
#78762=VECTOR ( 'NONE', #71221, 1000.000000000000000 ) ;
#78789=ORIENTED_EDGE ( 'NONE', *, *, #38287, .T. ) ;
#78792=DIRECTION ( 'NONE',  ( 1.000000000000000000, 0.000000000000000000, 0.000000000000000000 ) ) ;
#78800=ORIENTED_EDGE ( 'NONE', *, *, #59173, .F. ) ;
#78803=ORIENTED_EDGE ( 'NONE', *, *, #67680, .F. ) ;
#78828=CIRCLE ( 'NONE', #68745, 4.000000000000000000 ) ;
#78840=DIRECTION ( 'NONE',  ( -0.000000000000000000, 1.000000000000000000, -0.000000000000000000 ) ) ;
#78848=ORIENTED_EDGE ( 'NONE', *, *, #50813, .T. ) ;
#78856=DIRECTION ( 'NONE',  ( 1.000000000000000000, 0.000000000000000000, 0.000000000000000000 ) ) ;
#78857=ADVANCED_FACE ( 'NONE', ( #13727 ), #82193, .T. ) ;
#78863=VECTOR ( 'NONE', #21423, 1000.000000000000000 ) ;
#78888=EDGE_LOOP ( 'NONE', ( #36591, #34773, #44729, #80527 ) ) ;
#78905=DIRECTION ( 'NONE',  ( -1.000000000000000000, -0.000000000000000000, 0.000000000000000000 ) ) ;
#78914=DIRECTION ( 'NONE',  ( -0.000000000000000000, -1.000000000000000000, -0.000000000000000000 ) ) ;
#78918=FACE_OUTER_BOUND ( 'NONE', #48277, .T. ) ;
#78926=ORIENTED_EDGE ( 'NONE', *, *, #79029, .F. ) ;
#78932=CARTESIAN_POINT ( 'NONE',  ( 18.03205128205128105, -7.500000000000000000, 29.75000000000000355 ) ) ;
#78935=VECTOR ( 'NONE', #11702, 1000.000000000000000 ) ;
#78942=VECTOR ( 'NONE', #27835, 1000.000000000000000 ) ;
#78972=EDGE_LOOP ( 'NONE', ( #48589, #35594, #3724, #67248 ) ) ;
#78993=VECTOR ( 'NONE', #60647, 1000.000000000000000 ) ;
#78996=EDGE_LOOP ( 'NONE', ( #18909, #85129, #15896, #18146 ) ) ;
#79004=CYLINDRICAL_SURFACE ( 'NONE', #41835, 4.000000000000000000 ) ;
#79008=CARTESIAN_POINT ( 'NONE',  ( 20.00000000000000000, -4.000000000000000000, 29.75000000000000355 ) ) ;
#79018=FACE_OUTER_BOUND ( 'NONE', #46331, .T. ) ;
#79020=CARTESIAN_POINT ( 'NONE',  ( -10.03846153846153832, -11.50000000000000000, 29.75000000000000355 ) ) ;
#79029=EDGE_CURVE ( 'NONE', #46953, #52150, #24907, .T. ) ;
#79034=EDGE_LOOP ( 'NONE', ( #62189, #68820, #66436, #60688 ) ) ;
#79043=DIRECTION ( 'NONE',  ( -0.000000000000000000, 1.000000000000000000, -0.000000000000000000 ) ) ;
#79049=ADVANCED_FACE ( 'NONE', ( #17722 ), #66345, .T. ) ;
#79063=AXIS2_PLACEMENT_3D ( 'NONE', #4932, #32841, #40059 ) ;
#79079=EDGE_CURVE ( 'NONE', #33822, #48507, #50164, .T. ) ;
#79081=ADVANCED_FACE ( 'NONE', ( #72650 ), #24013, .T. ) ;
#79086=DIRECTION ( 'NONE',  ( -0.000000000000000000, 1.000000000000000000, -0.000000000000000000 ) ) ;
#79106=EDGE_CURVE ( 'NONE', #38268, #29864, #60273, .T. ) ;
#79118=VECTOR ( 'NONE', #85038, 1000.000000000000000 ) ;
#79121=ADVANCED_FACE ( 'NONE', ( #55046 ), #75324, .T. ) ;
#79123=CYLINDRICAL_SURFACE ( 'NONE', #75295, 4.000000000000000000 ) ;
#79162=DIRECTION ( 'NONE',  ( -1.000000000000000000, -0.000000000000000000, -0.000000000000000000 ) ) ;
#79190=VECTOR ( 'NONE', #82228, 1000.000000000000000 ) ;
#79201=EDGE_CURVE ( 'NONE', #48943, #29630, #35671, .T. ) ;
#79226=CYLINDRICAL_SURFACE ( 'NONE', #41897, 4.000000000000000000 ) ;
#79231=ORIENTED_EDGE ( 'NONE', *, *, #88036, .F. ) ;
#79245=AXIS2_PLACEMENT_3D ( 'NONE', #19068, #74017, #11421 ) ;
#79249=VERTEX_POINT ( 'NONE', #84310 ) ;
#79282=LINE ( 'NONE', #17583, #67120 ) ;
#79292=LINE ( 'NONE', #17594, #23517 ) ;
#79305=ADVANCED_FACE ( 'NONE', ( #36552 ), #7753, .T. ) ;
#79306=EDGE_CURVE ( 'NONE', #11720, #72149, #35213, .T. ) ;
#79307=VERTEX_POINT ( 'NONE', #12956 ) ;
#79308=ORIENTED_EDGE ( 'NONE', *, *, #7479, .F. ) ;
#79322=CARTESIAN_POINT ( 'NONE',  ( 9.070512820512819374, -7.500000000000000000, 29.75000000000000355 ) ) ;
#79332=DIRECTION ( 'NONE',  ( 1.000000000000000000, 0.000000000000000000, -0.000000000000000000 ) ) ;
#79342=ORIENTED_EDGE ( 'NONE', *, *, #10951, .T. ) ;
#79345=DIRECTION ( 'NONE',  ( 1.000000000000000000, 0.000000000000000000, 0.000000000000000000 ) ) ;
#79365=VERTEX_POINT ( 'NONE', #53939 ) ;
#79368=CARTESIAN_POINT ( 'NONE',  ( 0.000000000000000000, -11.00000000000000000, 29.75000000000000355 ) ) ;
#79390=DIRECTION ( 'NONE',  ( -0.000000000000000000, 1.000000000000000000, -0.000000000000000000 ) ) ;
#79393=LINE ( 'NONE', #44694, #60670 ) ;
#79394=ADVANCED_FACE ( 'NONE', ( #87306 ), #31904, .F. ) ;
#79411=CARTESIAN_POINT ( 'NONE',  ( 17.78205128205128105, -11.00000000000000000, 29.75000000000000355 ) ) ;
#79414=ORIENTED_EDGE ( 'NONE', *, *, #47631, .T. ) ;
#79421=DIRECTION ( 'NONE',  ( -1.000000000000000000, -0.000000000000000000, -0.000000000000000000 ) ) ;
#79422=EDGE_CURVE ( 'NONE', #53945, #10355, #32783, .T. ) ;
#79424=EDGE_CURVE ( 'NONE', #51615, #75410, #25136, .T. ) ;
#79430=ORIENTED_EDGE ( 'NONE', *, *, #2502, .F. ) ;
#79469=ADVANCED_FACE ( 'NONE', ( #54825 ), #55266, .F. ) ;
#79472=VECTOR ( 'NONE', #22751, 1000.000000000000000 ) ;
#79478=DIRECTION ( 'NONE',  ( 0.000000000000000000, 0.000000000000000000, -1.000000000000000000 ) ) ;
#79482=DIRECTION ( 'NONE',  ( -1.000000000000000000, 0.000000000000000000, -0.000000000000000000 ) ) ;
#79487=ORIENTED_EDGE ( 'NONE', *, *, #1434, .F. ) ;
#79517=EDGE_CURVE ( 'NONE', #79365, #24740, #56156, .T. ) ;
#79520=CARTESIAN_POINT ( 'NONE',  ( -2.544871794871793824, -3.499999999999999556, 29.75000000000000355 ) ) ;
#79524=ORIENTED_EDGE ( 'NONE', *, *, #71305, .F. ) ;
#79533=DIRECTION ( 'NONE',  ( 1.000000000000000000, 0.000000000000000000, 0.000000000000000000 ) ) ;
#79535=VECTOR ( 'NONE', #32643, 1000.000000000000000 ) ;
#79537=ORIENTED_EDGE ( 'NONE', *, *, #26751, .F. ) ;
#79540=LINE ( 'NONE', #25477, #7112 ) ;
#79545=DIRECTION ( 'NONE',  ( -1.000000000000000000, -0.000000000000000000, -0.000000000000000000 ) ) ;
#79560=EDGE_CURVE ( 'NONE', #9433, #23520, #71428, .T. ) ;
#79568=CARTESIAN_POINT ( 'NONE',  ( 16.81410256410256565, -11.00000000000000000, 29.75000000000000355 ) ) ;
#79574=ADVANCED_FACE ( 'NONE', ( #37649 ), #64224, .F. ) ;
#79583=DIRECTION ( 'NONE',  ( 0.000000000000000000, 0.000000000000000000, -1.000000000000000000 ) ) ;
#79590=CARTESIAN_POINT ( 'NONE',  ( 16.09615384615384670, -11.00000000000000000, 29.75000000000000355 ) ) ;
#79594=DIRECTION ( 'NONE',  ( -0.000000000000000000, -0.000000000000000000, 1.000000000000000000 ) ) ;
#79615=CARTESIAN_POINT ( 'NONE',  ( 0.6089743589743582541, -7.500000000000000000, 29.75000000000000355 ) ) ;
#79617=DIRECTION ( 'NONE',  ( 0.000000000000000000, 0.000000000000000000, -1.000000000000000000 ) ) ;
#79619=DIRECTION ( 'NONE',  ( -1.000000000000000000, -0.000000000000000000, -0.000000000000000000 ) ) ;
#79627=ORIENTED_EDGE ( 'NONE', *, *, #61033, .T. ) ;
#79628=ORIENTED_EDGE ( 'NONE', *, *, #18578, .T. ) ;
#79652=DIRECTION ( 'NONE',  ( -1.000000000000000000, -0.000000000000000000, 0.000000000000000000 ) ) ;
#79655=LINE ( 'NONE', #12531, #56814 ) ;
#79656=ORIENTED_EDGE ( 'NONE', *, *, #82460, .F. ) ;
#79661=EDGE_CURVE ( 'NONE', #17849, #8287, #43522, .T. ) ;
#79662=CARTESIAN_POINT ( 'NONE',  ( 0.000000000000000000, -11.00000000000000000, 29.75000000000000355 ) ) ;
#79684=EDGE_CURVE ( 'NONE', #63745, #88209, #79540, .T. ) ;
#79692=CIRCLE ( 'NONE', #26465, 4.000000000000000000 ) ;
#79707=CARTESIAN_POINT ( 'NONE',  ( -3.262820512820514107, -11.50000000000000000, 29.75000000000000355 ) ) ;
#79709=EDGE_CURVE ( 'NONE', #60898, #40946, #72764, .T. ) ;
#79710=ADVANCED_FACE ( 'NONE', ( #58806 ), #32671, .F. ) ;
#79718=PLANE ( 'NONE',  #64268 ) ;
#79728=ORIENTED_EDGE ( 'NONE', *, *, #45840, .F. ) ;
#79741=EDGE_CURVE ( 'NONE', #29049, #62375, #11076, .T. ) ;
#79754=ORIENTED_EDGE ( 'NONE', *, *, #16615, .T. ) ;
#79779=CARTESIAN_POINT ( 'NONE',  ( 15.84615384615384670, -11.50000000000000000, 29.75000000000000355 ) ) ;
#79802=VERTEX_POINT ( 'NONE', #6101 ) ;
#79852=CARTESIAN_POINT ( 'NONE',  ( -16.09615384615384670, -7.500000000000000000, 29.75000000000000355 ) ) ;
#79854=CARTESIAN_POINT ( 'NONE',  ( 2.294871794871793380, -3.499999999999999556, 29.75000000000000355 ) ) ;
#79881=FACE_OUTER_BOUND ( 'NONE', #66152, .T. ) ;
#79889=DIRECTION ( 'NONE',  ( -1.000000000000000000, -0.000000000000000000, 0.000000000000000000 ) ) ;
#79897=EDGE_LOOP ( 'NONE', ( #50811, #53539, #86843, #2183 ) ) ;
#79908=ORIENTED_EDGE ( 'NONE', *, *, #44846, .F. ) ;
#79909=VECTOR ( 'NONE', #50226, 1000.000000000000000 ) ;
#79932=ORIENTED_EDGE ( 'NONE', *, *, #88080, .F. ) ;
#79953=DIRECTION ( 'NONE',  ( -1.000000000000000000, -0.000000000000000000, 0.000000000000000000 ) ) ;
#79976=EDGE_LOOP ( 'NONE', ( #14378, #29300, #52498, #13430 ) ) ;
#79977=LINE ( 'NONE', #73223, #81847 ) ;
#79981=EDGE_CURVE ( 'NONE', #34673, #8287, #21821, .T. ) ;
#79996=VERTEX_POINT ( 'NONE', #78527 ) ;
#79997=DIRECTION ( 'NONE',  ( -1.000000000000000000, 0.000000000000000000, -0.000000000000000000 ) ) ;
#80001=PLANE ( 'NONE',  #70381 ) ;
#80007=EDGE_CURVE ( 'NONE', #80662, #80137, #84866, .T. ) ;
#80009=CARTESIAN_POINT ( 'NONE',  ( 0.000000000000000000, -11.00000000000000000, 29.75000000000000355 ) ) ;
#80013=DIRECTION ( 'NONE',  ( 1.000000000000000000, 0.000000000000000000, 0.000000000000000000 ) ) ;
#80031=LINE ( 'NONE', #6148, #18196 ) ;
#80039=CIRCLE ( 'NONE', #36875, 4.000000000000000000 ) ;
#80061=ORIENTED_EDGE ( 'NONE', *, *, #21291, .F. ) ;
#80082=VERTEX_POINT ( 'NONE', #51936 ) ;
#80094=VERTEX_POINT ( 'NONE', #68567 ) ;
#80111=FACE_OUTER_BOUND ( 'NONE', #6039, .T. ) ;
#80118=PLANE ( 'NONE',  #7527 ) ;
#80124=CARTESIAN_POINT ( 'NONE',  ( -19.50000000000000000, -3.499999999999999556, 29.75000000000000355 ) ) ;
#80133=AXIS2_PLACEMENT_3D ( 'NONE', #39773, #79421, #52372 ) ;
#80137=VERTEX_POINT ( 'NONE', #55054 ) ;
#80142=CARTESIAN_POINT ( 'NONE',  ( -12.22435897435897267, -3.499999999999999556, 29.75000000000000355 ) ) ;
#80152=FACE_OUTER_BOUND ( 'NONE', #37015, .T. ) ;
#80167=VECTOR ( 'NONE', #5226, 1000.000000000000000 ) ;
#80171=ORIENTED_EDGE ( 'NONE', *, *, #6529, .T. ) ;
#80173=PLANE ( 'NONE',  #68520 ) ;
#80174=ORIENTED_EDGE ( 'NONE', *, *, #70775, .T. ) ;
#80181=ORIENTED_EDGE ( 'NONE', *, *, #3084, .F. ) ;
#80219=CARTESIAN_POINT ( 'NONE',  ( 0.000000000000000000, -11.00000000000000000, 29.75000000000000355 ) ) ;
#80223=FACE_OUTER_BOUND ( 'NONE', #41750, .T. ) ;
#80227=ORIENTED_EDGE ( 'NONE', *, *, #63159, .T. ) ;
#80237=DIRECTION ( 'NONE',  ( -0.000000000000000000, 1.000000000000000000, -0.000000000000000000 ) ) ;
#80238=VECTOR ( 'NONE', #68110, 1000.000000000000000 ) ;
#80247=LINE ( 'NONE', #5025, #20461 ) ;
#80249=EDGE_CURVE ( 'NONE', #13621, #82495, #9096, .T. ) ;
#80254=CARTESIAN_POINT ( 'NONE',  ( -12.94230769230769162, -7.500000000000000000, 29.75000000000000355 ) ) ;
#80255=PLANE ( 'NONE',  #57547 ) ;
#80259=EDGE_LOOP ( 'NONE', ( #66109, #44719, #71424, #37025 ) ) ;
#80260=LINE ( 'NONE', #5491, #85726 ) ;
#80272=DIRECTION ( 'NONE',  ( -1.000000000000000000, -0.000000000000000000, -0.000000000000000000 ) ) ;
#80277=DIRECTION ( 'NONE',  ( -0.000000000000000000, 1.000000000000000000, -0.000000000000000000 ) ) ;
#80286=CARTESIAN_POINT ( 'NONE',  ( 0.000000000000000000, -11.00000000000000000, 29.75000000000000355 ) ) ;
#80293=AXIS2_PLACEMENT_3D ( 'NONE', #80919, #82689, #61504 ) ;
#80296=DIRECTION ( 'NONE',  ( -1.000000000000000000, -0.000000000000000000, -0.000000000000000000 ) ) ;
#80298=ORIENTED_EDGE ( 'NONE', *, *, #83687, .F. ) ;
#80303=VECTOR ( 'NONE', #39552, 1000.000000000000000 ) ;
#80306=EDGE_CURVE ( 'NONE', #77956, #83716, #30202, .T. ) ;
#80325=EDGE_LOOP ( 'NONE', ( #41922, #31040, #44289, #1664, #57324 ) ) ;
#80337=CARTESIAN_POINT ( 'NONE',  ( 18.75000000000000000, -3.499999999999999556, 29.75000000000000355 ) ) ;
#80361=ORIENTED_EDGE ( 'NONE', *, *, #44209, .T. ) ;
#80378=LINE ( 'NONE', #46136, #59169 ) ;
#80385=CARTESIAN_POINT ( 'NONE',  ( -19.50000000000000000, -3.499999999999999556, 29.75000000000000355 ) ) ;
#80387=EDGE_LOOP ( 'NONE', ( #39025, #78514, #76413, #30333 ) ) ;
#80397=CARTESIAN_POINT ( 'NONE',  ( -5.448717948717948012, -3.499999999999999556, 29.75000000000000355 ) ) ;
#80410=PLANE ( 'NONE',  #75770 ) ;
#80446=DIRECTION ( 'NONE',  ( -0.000000000000000000, 1.000000000000000000, -0.000000000000000000 ) ) ;
#80471=DIRECTION ( 'NONE',  ( -1.000000000000000000, -0.000000000000000000, -0.000000000000000000 ) ) ;
#80475=LINE ( 'NONE', #87244, #18185 ) ;
#80484=LINE ( 'NONE', #86816, #70451 ) ;
#80489=CIRCLE ( 'NONE', #12905, 4.000000000000000000 ) ;
#80493=AXIS2_PLACEMENT_3D ( 'NONE', #84876, #50625, #76327 ) ;
#80498=CIRCLE ( 'NONE', #10008, 4.000000000000000000 ) ;
#80502=DIRECTION ( 'NONE',  ( -1.000000000000000000, -0.000000000000000000, -0.000000000000000000 ) ) ;
#80508=ORIENTED_EDGE ( 'NONE', *, *, #26128, .F. ) ;
#80519=DIRECTION ( 'NONE',  ( 1.000000000000000000, 0.000000000000000000, 0.000000000000000000 ) ) ;
#80527=ORIENTED_EDGE ( 'NONE', *, *, #81435, .T. ) ;
#80531=CARTESIAN_POINT ( 'NONE',  ( -9.070512820512819374, -11.50000000000000000, 29.75000000000000355 ) ) ;
#80552=ORIENTED_EDGE ( 'NONE', *, *, #62319, .F. ) ;
#80567=CARTESIAN_POINT ( 'NONE',  ( 9.320512820512821150, -7.500000000000000000, 29.75000000000000355 ) ) ;
#80570=FACE_OUTER_BOUND ( 'NONE', #30663, .T. ) ;
#80574=ORIENTED_EDGE ( 'NONE', *, *, #66414, .T. ) ;
#80582=ORIENTED_EDGE ( 'NONE', *, *, #56615, .T. ) ;
#80590=SURFACE_SIDE_STYLE ('',( #86915 ) ) ;
#80591=CARTESIAN_POINT ( 'NONE',  ( -2.544871794871794268, -7.500000000000000000, 29.75000000000000355 ) ) ;
#80613=CARTESIAN_POINT ( 'NONE',  ( 17.06410256410256565, -11.50000000000000000, 29.75000000000000355 ) ) ;
#80622=VECTOR ( 'NONE', #13100, 1000.000000000000000 ) ;
#80632=EDGE_LOOP ( 'NONE', ( #51855, #55275, #30046, #46662 ) ) ;
#80652=EDGE_CURVE ( 'NONE', #45222, #81743, #18401, .T. ) ;
#80659=EDGE_CURVE ( 'NONE', #19601, #25570, #71552, .T. ) ;
#80662=VERTEX_POINT ( 'NONE', #64787 ) ;
#80686=CIRCLE ( 'NONE', #37519, 4.000000000000000000 ) ;
#80692=CARTESIAN_POINT ( 'NONE',  ( 20.00000000000000000, -7.500000000000000000, 29.75000000000000355 ) ) ;
#80704=EDGE_LOOP ( 'NONE', ( #6836, #32036, #60055, #69823 ) ) ;
#80705=EDGE_CURVE ( 'NONE', #26482, #51615, #69015, .T. ) ;
#80716=FACE_OUTER_BOUND ( 'NONE', #78996, .T. ) ;
#80718=LINE ( 'NONE', #82487, #75682 ) ;
#80719=DIRECTION ( 'NONE',  ( 0.000000000000000000, 0.000000000000000000, -1.000000000000000000 ) ) ;
#80730=VERTEX_POINT ( 'NONE', #58473 ) ;
#80758=CARTESIAN_POINT ( 'NONE',  ( -9.320512820512821150, -11.50000000000000000, 29.75000000000000355 ) ) ;
#80762=EDGE_CURVE ( 'NONE', #61773, #6496, #26492, .T. ) ;
#80765=EDGE_CURVE ( 'NONE', #77416, #52415, #70014, .T. ) ;
#80795=FACE_OUTER_BOUND ( 'NONE', #3310, .T. ) ;
#80799=VERTEX_POINT ( 'NONE', #26048 ) ;
#80804=CARTESIAN_POINT ( 'NONE',  ( 20.00000000000000000, -4.000000000000000000, 29.75000000000000355 ) ) ;
#80809=DIRECTION ( 'NONE',  ( 0.000000000000000000, 0.000000000000000000, -1.000000000000000000 ) ) ;
#80815=ORIENTED_EDGE ( 'NONE', *, *, #73130, .T. ) ;
#80836=ORIENTED_EDGE ( 'NONE', *, *, #88585, .T. ) ;
#80859=EDGE_LOOP ( 'NONE', ( #43591, #6242, #36526, #66271 ) ) ;
#80863=LINE ( 'NONE', #74093, #25450 ) ;
#80866=EDGE_LOOP ( 'NONE', ( #2177, #83991, #24346, #43080 ) ) ;
#80900=ORIENTED_EDGE ( 'NONE', *, *, #84379, .T. ) ;
#80901=VECTOR ( 'NONE', #30214, 1000.000000000000000 ) ;
#80912=CARTESIAN_POINT ( 'NONE',  ( -18.03205128205128105, -7.500000000000000000, 29.75000000000000355 ) ) ;
#80913=EDGE_CURVE ( 'NONE', #22218, #84168, #71339, .T. ) ;
#80919=CARTESIAN_POINT ( 'NONE',  ( 17.06410256410256565, -7.500000000000000000, 29.75000000000000355 ) ) ;
#80932=ORIENTED_EDGE ( 'NONE', *, *, #1980, .F. ) ;
#80938=CARTESIAN_POINT ( 'NONE',  ( -19.50000000000000000, -3.499999999999999556, 29.75000000000000355 ) ) ;
#80946=CYLINDRICAL_SURFACE ( 'NONE', #81851, 4.000000000000000000 ) ;
#80986=DIRECTION ( 'NONE',  ( -0.000000000000000000, 1.000000000000000000, -0.000000000000000000 ) ) ;
#80997=ORIENTED_EDGE ( 'NONE', *, *, #87174, .F. ) ;
#81003=DIRECTION ( 'NONE',  ( 1.000000000000000000, 0.000000000000000000, 0.000000000000000000 ) ) ;
#81014=PLANE ( 'NONE',  #83518 ) ;
#81017=ORIENTED_EDGE ( 'NONE', *, *, #50264, .T. ) ;
#81024=ORIENTED_EDGE ( 'NONE', *, *, #70775, .F. ) ;
#81031=EDGE_CURVE ( 'NONE', #74652, #53825, #72677, .T. ) ;
#81037=EDGE_LOOP ( 'NONE', ( #8096, #50537, #61561, #65278 ) ) ;
#81050=DIRECTION ( 'NONE',  ( 1.000000000000000000, 0.000000000000000000, 0.000000000000000000 ) ) ;
#81053=CIRCLE ( 'NONE', #42208, 4.000000000000000000 ) ;
#81083=DIRECTION ( 'NONE',  ( 1.000000000000000000, 0.000000000000000000, 0.000000000000000000 ) ) ;
#81090=AXIS2_PLACEMENT_3D ( 'NONE', #25728, #74811, #40583 ) ;
#81105=VERTEX_POINT ( 'NONE', #32579 ) ;
#81113=DIRECTION ( 'NONE',  ( -0.000000000000000000, 0.000000000000000000, 1.000000000000000000 ) ) ;
#81143=EDGE_LOOP ( 'NONE', ( #32544, #84072, #60711, #19271 ) ) ;
#81145=FACE_OUTER_BOUND ( 'NONE', #67816, .T. ) ;
#81148=LINE ( 'NONE', #6376, #64685 ) ;
#81150=VECTOR ( 'NONE', #24597, 1000.000000000000000 ) ;
#81151=ORIENTED_EDGE ( 'NONE', *, *, #49700, .F. ) ;
#81154=FACE_OUTER_BOUND ( 'NONE', #26064, .T. ) ;
#81176=CARTESIAN_POINT ( 'NONE',  ( 10.28846153846153832, -7.500000000000000000, 29.75000000000000355 ) ) ;
#81190=LINE ( 'NONE', #5075, #69582 ) ;
#81194=ORIENTED_EDGE ( 'NONE', *, *, #54353, .F. ) ;
#81198=EDGE_CURVE ( 'NONE', #15501, #64772, #7336, .T. ) ;
#81208=ORIENTED_EDGE ( 'NONE', *, *, #24656, .T. ) ;
#81220=ADVANCED_FACE ( 'NONE', ( #48305 ), #7774, .F. ) ;
#81224=VERTEX_POINT ( 'NONE', #1898 ) ;
#81228=DIRECTION ( 'NONE',  ( 0.000000000000000000, 0.000000000000000000, -1.000000000000000000 ) ) ;
#81234=VERTEX_POINT ( 'NONE', #23489 ) ;
#81240=AXIS2_PLACEMENT_3D ( 'NONE', #54060, #5893, #46426 ) ;
#81244=CARTESIAN_POINT ( 'NONE',  ( -10.28846153846153832, -7.500000000000000000, 29.75000000000000355 ) ) ;
#81256=LINE ( 'NONE', #26302, #72777 ) ;
#81264=EDGE_CURVE ( 'NONE', #65753, #1878, #49641, .T. ) ;
#81271=ADVANCED_FACE ( 'NONE', ( #84332 ), #63595, .T. ) ;
#81284=DIRECTION ( 'NONE',  ( 1.000000000000000000, 0.000000000000000000, 0.000000000000000000 ) ) ;
#81285=CARTESIAN_POINT ( 'NONE',  ( 0.000000000000000000, -11.00000000000000000, 29.75000000000000355 ) ) ;
#81299=DIRECTION ( 'NONE',  ( 1.000000000000000000, 0.000000000000000000, 0.000000000000000000 ) ) ;
#81303=CARTESIAN_POINT ( 'NONE',  ( -17.78205128205128105, -7.500000000000000000, 29.75000000000000355 ) ) ;
#81312=VECTOR ( 'NONE', #68348, 1000.000000000000000 ) ;
#81313=DIRECTION ( 'NONE',  ( 0.000000000000000000, 0.000000000000000000, -1.000000000000000000 ) ) ;
#81314=CYLINDRICAL_SURFACE ( 'NONE', #19182, 4.000000000000000000 ) ;
#81321=EDGE_CURVE ( 'NONE', #64220, #1652, #71230, .T. ) ;
#81341=ORIENTED_EDGE ( 'NONE', *, *, #46833, .F. ) ;
#81357=AXIS2_PLACEMENT_3D ( 'NONE', #82437, #13515, #2528 ) ;
#81374=CARTESIAN_POINT ( 'NONE',  ( -19.50000000000000000, -11.50000000000000000, 29.75000000000000355 ) ) ;
#81390=DIRECTION ( 'NONE',  ( -0.000000000000000000, 1.000000000000000000, -0.000000000000000000 ) ) ;
#81403=CYLINDRICAL_SURFACE ( 'NONE', #51239, 4.000000000000000000 ) ;
#81420=CYLINDRICAL_SURFACE ( 'NONE', #48110, 4.000000000000000000 ) ;
#81423=VECTOR ( 'NONE', #12440, 1000.000000000000000 ) ;
#81431=FACE_OUTER_BOUND ( 'NONE', #38755, .T. ) ;
#81432=CARTESIAN_POINT ( 'NONE',  ( 16.09615384615384670, -11.50000000000000000, 29.75000000000000355 ) ) ;
#81433=AXIS2_PLACEMENT_3D ( 'NONE', #13647, #27161, #82117 ) ;
#81435=EDGE_CURVE ( 'NONE', #52641, #63049, #32927, .T. ) ;
#81448=LINE ( 'NONE', #61594, #26392 ) ;
#81459=ORIENTED_EDGE ( 'NONE', *, *, #59881, .F. ) ;
#81465=DIRECTION ( 'NONE',  ( 1.000000000000000000, 0.000000000000000000, 0.000000000000000000 ) ) ;
#81468=ORIENTED_EDGE ( 'NONE', *, *, #42881, .T. ) ;
#81494=CARTESIAN_POINT ( 'NONE',  ( -8.352564102564102200, -11.50000000000000000, 29.75000000000000355 ) ) ;
#81500=LINE ( 'NONE', #53565, #21141 ) ;
#81509=DIRECTION ( 'NONE',  ( -1.000000000000000000, -0.000000000000000000, -0.000000000000000000 ) ) ;
#81510=VECTOR ( 'NONE', #82724, 1000.000000000000000 ) ;
#81518=DIRECTION ( 'NONE',  ( -1.000000000000000000, -0.000000000000000000, 0.000000000000000000 ) ) ;
#81558=CARTESIAN_POINT ( 'NONE',  ( 10.03846153846153832, -4.000000000000000000, 28.25000000000000000 ) ) ;
#81569=CARTESIAN_POINT ( 'NONE',  ( -17.78205128205128105, -3.499999999999999556, 29.75000000000000355 ) ) ;
#81575=DIRECTION ( 'NONE',  ( 1.000000000000000000, 0.000000000000000000, 0.000000000000000000 ) ) ;
#81614=VECTOR ( 'NONE', #41683, 1000.000000000000000 ) ;
#81620=AXIS2_PLACEMENT_3D ( 'NONE', #26261, #12745, #20393 ) ;
#81621=EDGE_CURVE ( 'NONE', #83291, #6970, #22947, .T. ) ;
#81623=DIRECTION ( 'NONE',  ( -1.000000000000000000, -0.000000000000000000, -0.000000000000000000 ) ) ;
#81634=VERTEX_POINT ( 'NONE', #43225 ) ;
#81637=VERTEX_POINT ( 'NONE', #909 ) ;
#81641=VECTOR ( 'NONE', #86458, 1000.000000000000000 ) ;
#81647=ORIENTED_EDGE ( 'NONE', *, *, #38460, .T. ) ;
#81670=AXIS2_PLACEMENT_3D ( 'NONE', #8139, #14447, #61731 ) ;
#81684=ORIENTED_EDGE ( 'NONE', *, *, #59850, .T. ) ;
#81698=CARTESIAN_POINT ( 'NONE',  ( -19.50000000000000000, -3.499999999999999556, 29.75000000000000355 ) ) ;
#81699=DIRECTION ( 'NONE',  ( -1.000000000000000000, -0.000000000000000000, -0.000000000000000000 ) ) ;
#81705=CARTESIAN_POINT ( 'NONE',  ( -18.75000000000000000, -3.499999999999999556, 29.75000000000000355 ) ) ;
#81726=CARTESIAN_POINT ( 'NONE',  ( -12.94230769230769162, -3.499999999999999556, 29.75000000000000355 ) ) ;
#81743=VERTEX_POINT ( 'NONE', #52636 ) ;
#81747=ORIENTED_EDGE ( 'NONE', *, *, #44474, .T. ) ;
#81751=DIRECTION ( 'NONE',  ( 0.000000000000000000, 0.000000000000000000, -1.000000000000000000 ) ) ;
#81752=CARTESIAN_POINT ( 'NONE',  ( 20.00000000000000000, -11.00000000000000000, 28.25000000000000000 ) ) ;
#81769=ORIENTED_EDGE ( 'NONE', *, *, #55807, .F. ) ;
#81771=AXIS2_PLACEMENT_3D ( 'NONE', #21471, #29131, #76420 ) ;
#81786=DIRECTION ( 'NONE',  ( -1.000000000000000000, -0.000000000000000000, -0.000000000000000000 ) ) ;
#81787=ORIENTED_EDGE ( 'NONE', *, *, #86757, .F. ) ;
#81805=CARTESIAN_POINT ( 'NONE',  ( 0.000000000000000000, -11.00000000000000000, 29.75000000000000355 ) ) ;
#81806=DIRECTION ( 'NONE',  ( -0.000000000000000000, 1.000000000000000000, -0.000000000000000000 ) ) ;
#81831=EDGE_CURVE ( 'NONE', #88166, #3856, #57464, .T. ) ;
#81833=DIRECTION ( 'NONE',  ( 0.000000000000000000, 0.000000000000000000, -1.000000000000000000 ) ) ;
#81847=VECTOR ( 'NONE', #11522, 1000.000000000000000 ) ;
#81851=AXIS2_PLACEMENT_3D ( 'NONE', #17897, #46695, #5271 ) ;
#81870=ORIENTED_EDGE ( 'NONE', *, *, #53737, .F. ) ;
#81881=VERTEX_POINT ( 'NONE', #2512 ) ;
#81882=LINE ( 'NONE', #20174, #43242 ) ;
#81898=AXIS2_PLACEMENT_3D ( 'NONE', #68927, #21627, #42362 ) ;
#81899=CARTESIAN_POINT ( 'NONE',  ( -8.352564102564102200, -3.499999999999999556, 29.75000000000000355 ) ) ;
#81906=VERTEX_POINT ( 'NONE', #48311 ) ;
#81908=VECTOR ( 'NONE', #39852, 1000.000000000000000 ) ;
#81911=ORIENTED_EDGE ( 'NONE', *, *, #50806, .F. ) ;
#81921=ORIENTED_EDGE ( 'NONE', *, *, #35687, .F. ) ;
#81968=ORIENTED_EDGE ( 'NONE', *, *, #82254, .F. ) ;
#81972=CIRCLE ( 'NONE', #25893, 4.000000000000000000 ) ;
#81979=DIRECTION ( 'NONE',  ( 0.000000000000000000, 0.000000000000000000, -1.000000000000000000 ) ) ;
#82020=VECTOR ( 'NONE', #34472, 1000.000000000000000 ) ;
#82033=FACE_OUTER_BOUND ( 'NONE', #4873, .T. ) ;
#82045=LINE ( 'NONE', #48679, #60789 ) ;
#82072=PLANE ( 'NONE',  #25581 ) ;
#82085=VECTOR ( 'NONE', #59549, 1000.000000000000000 ) ;
#82091=ORIENTED_EDGE ( 'NONE', *, *, #17674, .T. ) ;
#82108=CARTESIAN_POINT ( 'NONE',  ( 0.000000000000000000, -2.085786437626902856, 28.75000000000000000 ) ) ;
#82117=DIRECTION ( 'NONE',  ( 0.000000000000000000, 0.000000000000000000, -1.000000000000000000 ) ) ;
#82122=DIRECTION ( 'NONE',  ( -1.000000000000000000, -0.000000000000000000, -0.000000000000000000 ) ) ;
#82129=CARTESIAN_POINT ( 'NONE',  ( -16.81410256410256565, -7.500000000000000000, 29.75000000000000355 ) ) ;
#82132=EDGE_CURVE ( 'NONE', #58964, #1652, #19413, .T. ) ;
#82148=CARTESIAN_POINT ( 'NONE',  ( 17.78205128205128105, -11.50000000000000000, 29.75000000000000355 ) ) ;
#82150=EDGE_CURVE ( 'NONE', #85054, #51499, #25730, .T. ) ;
#82175=ORIENTED_EDGE ( 'NONE', *, *, #36677, .T. ) ;
#82184=DIRECTION ( 'NONE',  ( 1.000000000000000000, 0.000000000000000000, 0.000000000000000000 ) ) ;
#82185=VECTOR ( 'NONE', #78840, 1000.000000000000000 ) ;
#82193=CYLINDRICAL_SURFACE ( 'NONE', #64561, 4.000000000000000000 ) ;
#82205=CARTESIAN_POINT ( 'NONE',  ( -19.50000000000000000, -3.499999999999999556, 29.75000000000000355 ) ) ;
#82221=VERTEX_POINT ( 'NONE', #6359 ) ;
#82228=DIRECTION ( 'NONE',  ( -1.000000000000000000, -0.000000000000000000, -0.000000000000000000 ) ) ;
#82243=EDGE_CURVE ( 'NONE', #29224, #30312, #62604, .T. ) ;
#82246=LINE ( 'NONE', #81805, #83752 ) ;
#82247=VECTOR ( 'NONE', #42845, 1000.000000000000000 ) ;
#82250=EDGE_LOOP ( 'NONE', ( #14402, #33329, #73078, #22374 ) ) ;
#82254=EDGE_CURVE ( 'NONE', #4576, #29049, #28382, .T. ) ;
#82256=EDGE_LOOP ( 'NONE', ( #24480, #43829, #11593, #39407 ) ) ;
#82265=CARTESIAN_POINT ( 'NONE',  ( 0.000000000000000000, -11.00000000000000000, 29.75000000000000355 ) ) ;
#82266=CARTESIAN_POINT ( 'NONE',  ( -10.03846153846153832, -1.926643599941765039, 29.65000000000000213 ) ) ;
#82278=EDGE_CURVE ( 'NONE', #29049, #49385, #7235, .T. ) ;
#82279=DIRECTION ( 'NONE',  ( 0.000000000000000000, 0.000000000000000000, -1.000000000000000000 ) ) ;
#82281=CIRCLE ( 'NONE', #88210, 4.000000000000000000 ) ;
#82290=VECTOR ( 'NONE', #13262, 1000.000000000000000 ) ;
#82299=CARTESIAN_POINT ( 'NONE',  ( -12.22435897435897267, -3.499999999999999556, 29.75000000000000355 ) ) ;
#82317=DIRECTION ( 'NONE',  ( 0.000000000000000000, 0.000000000000000000, -1.000000000000000000 ) ) ;
#82327=PLANE ( 'NONE',  #65179 ) ;
#82329=DIRECTION ( 'NONE',  ( 1.000000000000000000, 0.000000000000000000, 0.000000000000000000 ) ) ;
#82330=FACE_OUTER_BOUND ( 'NONE', #80859, .T. ) ;
#82334=CYLINDRICAL_SURFACE ( 'NONE', #41367, 4.000000000000000000 ) ;
#82335=AXIS2_PLACEMENT_3D ( 'NONE', #78691, #32283, #86805 ) ;
#82342=ORIENTED_EDGE ( 'NONE', *, *, #56793, .F. ) ;
#82349=CARTESIAN_POINT ( 'NONE',  ( -3.262820512820514107, -7.500000000000000000, 29.75000000000000355 ) ) ;
#82364=ORIENTED_EDGE ( 'NONE', *, *, #17840, .T. ) ;
#82374=CARTESIAN_POINT ( 'NONE',  ( 6.166666666666664298, -7.500000000000000000, 33.75000000000000000 ) ) ;
#82375=CARTESIAN_POINT ( 'NONE',  ( 0.000000000000000000, -11.00000000000000000, 29.75000000000000355 ) ) ;
#82377=VECTOR ( 'NONE', #23735, 1000.000000000000000 ) ;
#82402=CARTESIAN_POINT ( 'NONE',  ( 0.000000000000000000, -11.00000000000000000, 29.75000000000000355 ) ) ;
#82404=FACE_OUTER_BOUND ( 'NONE', #55262, .T. ) ;
#82419=AXIS2_PLACEMENT_3D ( 'NONE', #71637, #72532, #57252 ) ;
#82422=VERTEX_POINT ( 'NONE', #40041 ) ;
#82436=ORIENTED_EDGE ( 'NONE', *, *, #68330, .F. ) ;
#82437=CARTESIAN_POINT ( 'NONE',  ( -11.97435897435897267, -7.500000000000000000, 29.75000000000000355 ) ) ;
#82438=EDGE_LOOP ( 'NONE', ( #29399, #82651, #3074, #15367, #65023 ) ) ;
#82450=DIRECTION ( 'NONE',  ( 1.000000000000000000, 0.000000000000000000, 0.000000000000000000 ) ) ;
#82453=ORIENTED_EDGE ( 'NONE', *, *, #2448, .T. ) ;
#82460=EDGE_CURVE ( 'NONE', #81906, #87922, #74258, .T. ) ;
#82487=CARTESIAN_POINT ( 'NONE',  ( 2.544871794871792936, -11.50000000000000000, 29.75000000000000355 ) ) ;
#82492=DIRECTION ( 'NONE',  ( 1.000000000000000000, 0.000000000000000000, 0.000000000000000000 ) ) ;
#82493=CARTESIAN_POINT ( 'NONE',  ( -19.50000000000000000, -7.500000000000000000, 29.75000000000000355 ) ) ;
#82495=VERTEX_POINT ( 'NONE', #25174 ) ;
#82500=DIRECTION ( 'NONE',  ( -0.000000000000000000, 1.000000000000000000, -0.000000000000000000 ) ) ;
#82505=DIRECTION ( 'NONE',  ( -0.000000000000000000, 1.000000000000000000, -0.000000000000000000 ) ) ;
#82525=EDGE_CURVE ( 'NONE', #31713, #15081, #17982, .T. ) ;
#82529=AXIS2_PLACEMENT_3D ( 'NONE', #20350, #51774, #58105 ) ;
#82534=DIRECTION ( 'NONE',  ( 1.000000000000000000, 0.000000000000000000, 0.000000000000000000 ) ) ;
#82583=EDGE_LOOP ( 'NONE', ( #41652, #55156, #75895, #41068, #9663 ) ) ;
#82590=LINE ( 'NONE', #156, #42736 ) ;
#82594=CARTESIAN_POINT ( 'NONE',  ( 20.00000000000000000, -4.000000000000000000, 29.75000000000000355 ) ) ;
#82607=VECTOR ( 'NONE', #19256, 1000.000000000000000 ) ;
#82608=CARTESIAN_POINT ( 'NONE',  ( 0.000000000000000000, -11.00000000000000000, 29.75000000000000355 ) ) ;
#82637=LINE ( 'NONE', #54693, #550 ) ;
#82638=VERTEX_POINT ( 'NONE', #14319 ) ;
#82642=CARTESIAN_POINT ( 'NONE',  ( -13.91025641025641058, -11.50000000000000000, 29.75000000000000355 ) ) ;
#82643=ADVANCED_FACE ( 'NONE', ( #14772 ), #41353, .T. ) ;
#82651=ORIENTED_EDGE ( 'NONE', *, *, #76762, .F. ) ;
#82656=FACE_OUTER_BOUND ( 'NONE', #23830, .T. ) ;
#82671=ADVANCED_FACE ( 'NONE', ( #34145 ), #27395, .T. ) ;
#82673=ORIENTED_EDGE ( 'NONE', *, *, #85238, .T. ) ;
#82674=LINE ( 'NONE', #60603, #64320 ) ;
#82683=LINE ( 'NONE', #53863, #36576 ) ;
#82685=VECTOR ( 'NONE', #66522, 1000.000000000000000 ) ;
#82689=DIRECTION ( 'NONE',  ( 1.000000000000000000, 0.000000000000000000, 0.000000000000000000 ) ) ;
#82695=DIRECTION ( 'NONE',  ( -1.000000000000000000, -0.000000000000000000, -0.000000000000000000 ) ) ;
#82706=CARTESIAN_POINT ( 'NONE',  ( -19.50000000000000000, -3.499999999999999556, 29.75000000000000355 ) ) ;
#82724=DIRECTION ( 'NONE',  ( -1.000000000000000000, -0.000000000000000000, -0.000000000000000000 ) ) ;
#82727=DIRECTION ( 'NONE',  ( 0.000000000000000000, 0.000000000000000000, -1.000000000000000000 ) ) ;
#82737=ORIENTED_EDGE ( 'NONE', *, *, #67452, .T. ) ;
#82751=EDGE_CURVE ( 'NONE', #14834, #80094, #76341, .T. ) ;
#82755=CARTESIAN_POINT ( 'NONE',  ( 0.6089743589743582541, -11.50000000000000000, 29.75000000000000355 ) ) ;
#82778=CARTESIAN_POINT ( 'NONE',  ( -11.00641025641025550, -7.500000000000000000, 33.75000000000000000 ) ) ;
#82783=EDGE_CURVE ( 'NONE', #5809, #29827, #15217, .T. ) ;
#82788=PLANE ( 'NONE',  #64768 ) ;
#82789=VECTOR ( 'NONE', #56721, 1000.000000000000000 ) ;
#82793=EDGE_LOOP ( 'NONE', ( #55782, #77179, #39001, #83365 ) ) ;
#82800=DIRECTION ( 'NONE',  ( -0.000000000000000000, 1.000000000000000000, -0.000000000000000000 ) ) ;
#82808=ORIENTED_EDGE ( 'NONE', *, *, #20892, .F. ) ;
#82838=CARTESIAN_POINT ( 'NONE',  ( -16.09615384615384670, -11.00000000000000000, 29.75000000000000355 ) ) ;
#82850=EDGE_LOOP ( 'NONE', ( #47284, #1456, #2441, #62680 ) ) ;
#82853=CARTESIAN_POINT ( 'NONE',  ( 17.78205128205128105, -3.499999999999999556, 29.75000000000000355 ) ) ;
#82876=CARTESIAN_POINT ( 'NONE',  ( 18.03205128205128105, -3.499999999999999556, 29.75000000000000355 ) ) ;
#82878=VERTEX_POINT ( 'NONE', #47890 ) ;
#82889=CARTESIAN_POINT ( 'NONE',  ( 20.00000000000000000, -4.000000000000000000, 29.75000000000000355 ) ) ;
#82893=ORIENTED_EDGE ( 'NONE', *, *, #46833, .T. ) ;
#82901=LINE ( 'NONE', #28384, #41428 ) ;
#82932=EDGE_CURVE ( 'NONE', #66461, #48943, #63172, .T. ) ;
#82937=DIRECTION ( 'NONE',  ( 0.000000000000000000, 0.000000000000000000, -1.000000000000000000 ) ) ;
#82952=CARTESIAN_POINT ( 'NONE',  ( -15.84615384615384670, -3.499999999999999556, 29.75000000000000355 ) ) ;
#82954=EDGE_LOOP ( 'NONE', ( #26400, #6147, #40925, #65784, #44472 ) ) ;
#82955=DIRECTION ( 'NONE',  ( 1.000000000000000000, 0.000000000000000000, 0.000000000000000000 ) ) ;
#82959=ADVANCED_FACE ( 'NONE', ( #55977 ), #21751, .T. ) ;
#82961=LINE ( 'NONE', #32998, #18163 ) ;
#82966=AXIS2_PLACEMENT_3D ( 'NONE', #74103, #11065, #45279 ) ;
#82972=ORIENTED_EDGE ( 'NONE', *, *, #36241, .F. ) ;
#82983=CARTESIAN_POINT ( 'NONE',  ( 20.00000000000000000, -4.000000000000000000, 29.75000000000000355 ) ) ;
#83010=DIRECTION ( 'NONE',  ( 0.000000000000000000, 0.000000000000000000, 1.000000000000000000 ) ) ;
#83072=EDGE_CURVE ( 'NONE', #25462, #79249, #64485, .T. ) ;
#83076=ORIENTED_EDGE ( 'NONE', *, *, #13667, .T. ) ;
#83078=CARTESIAN_POINT ( 'NONE',  ( -4.230769230769230838, -3.499999999999999556, 29.75000000000000355 ) ) ;
#83079=CARTESIAN_POINT ( 'NONE',  ( 0.3589743589743582541, -7.500000000000000000, 29.75000000000000355 ) ) ;
#83095=CIRCLE ( 'NONE', #11208, 4.000000000000000000 ) ;
#83102=DIRECTION ( 'NONE',  ( 1.000000000000000000, 0.000000000000000000, 0.000000000000000000 ) ) ;
#83112=DIRECTION ( 'NONE',  ( 1.000000000000000000, 0.000000000000000000, 0.000000000000000000 ) ) ;
#83117=CARTESIAN_POINT ( 'NONE',  ( 8.352564102564102200, -3.499999999999999556, 29.75000000000000355 ) ) ;
#83129=AXIS2_PLACEMENT_3D ( 'NONE', #26124, #53592, #81083 ) ;
#83145=DIRECTION ( 'NONE',  ( -1.000000000000000000, 0.000000000000000000, -0.000000000000000000 ) ) ;
#83154=AXIS2_PLACEMENT_3D ( 'NONE', #35157, #76139, #22092 ) ;
#83159=PLANE ( 'NONE',  #48464 ) ;
#83162=CARTESIAN_POINT ( 'NONE',  ( 6.416666666666664298, -4.000000000000000000, 29.75000000000000355 ) ) ;
#83170=AXIS2_PLACEMENT_3D ( 'NONE', #6957, #82184, #13272 ) ;
#83202=ORIENTED_EDGE ( 'NONE', *, *, #48136, .F. ) ;
#83204=CARTESIAN_POINT ( 'NONE',  ( 0.000000000000000000, -11.00000000000000000, 29.75000000000000355 ) ) ;
#83214=ORIENTED_EDGE ( 'NONE', *, *, #24576, .F. ) ;
#83231=VERTEX_POINT ( 'NONE', #46896 ) ;
#83250=EDGE_CURVE ( 'NONE', #40554, #60613, #81148, .T. ) ;
#83255=VECTOR ( 'NONE', #7972, 1000.000000000000000 ) ;
#83257=PLANE ( 'NONE',  #24268 ) ;
#83282=LINE ( 'NONE', #82402, #3208 ) ;
#83284=ADVANCED_FACE ( 'NONE', ( #82033 ), #74380, .T. ) ;
#83291=VERTEX_POINT ( 'NONE', #53209 ) ;
#83299=DIRECTION ( 'NONE',  ( -1.000000000000000000, 0.000000000000000000, -0.000000000000000000 ) ) ;
#83300=DIRECTION ( 'NONE',  ( -1.000000000000000000, -0.000000000000000000, -0.000000000000000000 ) ) ;
#83308=VECTOR ( 'NONE', #11039, 1000.000000000000000 ) ;
#83320=ADVANCED_FACE ( 'NONE', ( #1374 ), #55872, .T. ) ;
#83328=DIRECTION ( 'NONE',  ( 0.000000000000000000, 0.000000000000000000, -1.000000000000000000 ) ) ;
#83353=EDGE_CURVE ( 'NONE', #21038, #18719, #61733, .T. ) ;
#83360=DIRECTION ( 'NONE',  ( -1.000000000000000000, -0.000000000000000000, -0.000000000000000000 ) ) ;
#83365=ORIENTED_EDGE ( 'NONE', *, *, #3398, .T. ) ;
#83370=CARTESIAN_POINT ( 'NONE',  ( -20.00000000000000000, -7.500000000000000000, 29.75000000000000355 ) ) ;
#83381=CARTESIAN_POINT ( 'NONE',  ( -0.3589743589743593088, -3.499999999999999556, 29.75000000000000355 ) ) ;
#83391=VECTOR ( 'NONE', #33646, 1000.000000000000000 ) ;
#83396=CARTESIAN_POINT ( 'NONE',  ( -18.75000000000000000, -3.499999999999999556, 29.75000000000000355 ) ) ;
#83410=EDGE_LOOP ( 'NONE', ( #23496, #13426, #38238, #67205, #5023 ) ) ;
#83422=ORIENTED_EDGE ( 'NONE', *, *, #56615, .F. ) ;
#83448=AXIS2_PLACEMENT_3D ( 'NONE', #62763, #83959, #35307 ) ;
#83457=CARTESIAN_POINT ( 'NONE',  ( 0.000000000000000000, -11.00000000000000000, 29.75000000000000355 ) ) ;
#83459=DIRECTION ( 'NONE',  ( 1.000000000000000000, 0.000000000000000000, 0.000000000000000000 ) ) ;
#83469=ADVANCED_FACE ( 'NONE', ( #42888 ), #48743, .F. ) ;
#83471=VERTEX_POINT ( 'NONE', #77990 ) ;
#83489=ORIENTED_EDGE ( 'NONE', *, *, #56829, .F. ) ;
#83502=AXIS2_PLACEMENT_3D ( 'NONE', #23808, #86443, #36892 ) ;
#83506=AXIS2_PLACEMENT_3D ( 'NONE', #49678, #77154, #36612 ) ;
#83514=ADVANCED_FACE ( 'NONE', ( #16293 ), #64457, .T. ) ;
#83518=AXIS2_PLACEMENT_3D ( 'NONE', #67049, #17972, #45425 ) ;
#83523=ORIENTED_EDGE ( 'NONE', *, *, #28553, .T. ) ;
#83530=DIRECTION ( 'NONE',  ( 1.000000000000000000, 0.000000000000000000, 0.000000000000000000 ) ) ;
#83540=LINE ( 'NONE', #43426, #36480 ) ;
#83554=LINE ( 'NONE', #78432, #30210 ) ;
#83572=DIRECTION ( 'NONE',  ( 0.000000000000000000, 0.000000000000000000, -1.000000000000000000 ) ) ;
#83579=DIRECTION ( 'NONE',  ( 1.000000000000000000, 0.000000000000000000, 0.000000000000000000 ) ) ;
#83595=CARTESIAN_POINT ( 'NONE',  ( -12.94230769230769162, -3.499999999999999556, 29.75000000000000355 ) ) ;
#83608=FACE_OUTER_BOUND ( 'NONE', #13446, .T. ) ;
#83611=FACE_OUTER_BOUND ( 'NONE', #88018, .T. ) ;
#83628=CARTESIAN_POINT ( 'NONE',  ( 3.512820512820510555, -7.500000000000000000, 29.75000000000000355 ) ) ;
#83639=LINE ( 'NONE', #29134, #50984 ) ;
#83641=EDGE_CURVE ( 'NONE', #15081, #18944, #25718, .T. ) ;
#83643=ORIENTED_EDGE ( 'NONE', *, *, #11768, .F. ) ;
#83649=DIRECTION ( 'NONE',  ( -1.000000000000000000, -0.000000000000000000, -0.000000000000000000 ) ) ;
#83652=EDGE_CURVE ( 'NONE', #9891, #50957, #34242, .T. ) ;
#83654=ORIENTED_EDGE ( 'NONE', *, *, #24522, .F. ) ;
#83655=EDGE_CURVE ( 'NONE', #81224, #235, #19401, .T. ) ;
#83682=CARTESIAN_POINT ( 'NONE',  ( -1.326923076923076872, -3.499999999999999556, 29.75000000000000355 ) ) ;
#83687=EDGE_CURVE ( 'NONE', #54838, #53642, #47758, .T. ) ;
#83690=DIRECTION ( 'NONE',  ( 0.000000000000000000, 0.000000000000000000, -1.000000000000000000 ) ) ;
#83698=AXIS2_PLACEMENT_3D ( 'NONE', #37679, #18306, #86341 ) ;
#83704=CARTESIAN_POINT ( 'NONE',  ( 20.00000000000000000, -11.50000000000000000, 29.75000000000000355 ) ) ;
#83711=PLANE ( 'NONE',  #5076 ) ;
#83716=VERTEX_POINT ( 'NONE', #54061 ) ;
#83726=LINE ( 'NONE', #851, #34091 ) ;
#83734=DIRECTION ( 'NONE',  ( 0.000000000000000000, 0.000000000000000000, -1.000000000000000000 ) ) ;
#83735=CARTESIAN_POINT ( 'NONE',  ( 14.16025641025641235, -7.500000000000000000, 29.75000000000000355 ) ) ;
#83736=VERTEX_POINT ( 'NONE', #81558 ) ;
#83745=CARTESIAN_POINT ( 'NONE',  ( -4.480769230769230838, -3.499999999999999556, 29.75000000000000355 ) ) ;
#83752=VECTOR ( 'NONE', #40378, 1000.000000000000000 ) ;
#83758=ORIENTED_EDGE ( 'NONE', *, *, #89019, .F. ) ;
#83765=CARTESIAN_POINT ( 'NONE',  ( -17.78205128205128105, -7.500000000000000000, 29.75000000000000355 ) ) ;
#83770=APPLICATION_CONTEXT ( 'automotive_design' ) ;
#83776=CARTESIAN_POINT ( 'NONE',  ( 12.22435897435897267, -7.500000000000000000, 33.75000000000000000 ) ) ;
#83780=VERTEX_POINT ( 'NONE', #26159 ) ;
#83786=VECTOR ( 'NONE', #87692, 1000.000000000000000 ) ;
#83803=EDGE_CURVE ( 'NONE', #5644, #29224, #56729, .T. ) ;
#83824=CARTESIAN_POINT ( 'NONE',  ( -13.19230769230769162, -7.500000000000000000, 33.75000000000000000 ) ) ;
#83831=DIRECTION ( 'NONE',  ( -0.000000000000000000, 0.000000000000000000, 1.000000000000000000 ) ) ;
#83848=VERTEX_POINT ( 'NONE', #76565 ) ;
#83855=EDGE_CURVE ( 'NONE', #51499, #46953, #69090, .T. ) ;
#83856=VECTOR ( 'NONE', #7939, 1000.000000000000000 ) ;
#83860=ORIENTED_EDGE ( 'NONE', *, *, #24427, .T. ) ;
#83862=EDGE_LOOP ( 'NONE', ( #31463, #49748, #54718, #78848, #79754 ) ) ;
#83864=EDGE_CURVE ( 'NONE', #30312, #88550, #14872, .T. ) ;
#83869=EDGE_LOOP ( 'NONE', ( #22100, #52467, #21715, #78101, #7487 ) ) ;
#83904=LINE ( 'NONE', #56849, #25572 ) ;
#83907=CARTESIAN_POINT ( 'NONE',  ( 18.75000000000000000, -3.499999999999999556, 29.75000000000000355 ) ) ;
#83913=FACE_OUTER_BOUND ( 'NONE', #39710, .T. ) ;
#83921=DIRECTION ( 'NONE',  ( 1.000000000000000000, 0.000000000000000000, 0.000000000000000000 ) ) ;
#83923=ORIENTED_EDGE ( 'NONE', *, *, #62968, .T. ) ;
#83928=FACE_OUTER_BOUND ( 'NONE', #9640, .T. ) ;
#83937=DIRECTION ( 'NONE',  ( -1.000000000000000000, -0.000000000000000000, -0.000000000000000000 ) ) ;
#83941=DIRECTION ( 'NONE',  ( -0.000000000000000000, 1.000000000000000000, -0.000000000000000000 ) ) ;
#83953=VECTOR ( 'NONE', #35084, 1000.000000000000000 ) ;
#83955=VECTOR ( 'NONE', #54163, 1000.000000000000000 ) ;
#83959=DIRECTION ( 'NONE',  ( 0.000000000000000000, 0.000000000000000000, 1.000000000000000000 ) ) ;
#83966=ADVANCED_FACE ( 'NONE', ( #86892 ), #58480, .F. ) ;
#83980=AXIS2_PLACEMENT_3D ( 'NONE', #45546, #58164, #17643 ) ;
#83982=ORIENTED_EDGE ( 'NONE', *, *, #54826, .T. ) ;
#83991=ORIENTED_EDGE ( 'NONE', *, *, #35036, .T. ) ;
#84004=VECTOR ( 'NONE', #11843, 1000.000000000000000 ) ;
#84009=VECTOR ( 'NONE', #63372, 1000.000000000000000 ) ;
#84022=PLANE ( 'NONE',  #78665 ) ;
#84035=LINE ( 'NONE', #83595, #7348 ) ;
#84036=ORIENTED_EDGE ( 'NONE', *, *, #71397, .T. ) ;
#84038=EDGE_CURVE ( 'NONE', #84195, #74179, #11658, .T. ) ;
#84059=EDGE_CURVE ( 'NONE', #40946, #24532, #17327, .T. ) ;
#84068=ADVANCED_FACE ( 'NONE', ( #80570 ), #61603, .T. ) ;
#84072=ORIENTED_EDGE ( 'NONE', *, *, #71397, .F. ) ;
#84076=AXIS2_PLACEMENT_3D ( 'NONE', #23270, #36358, #29601 ) ;
#84102=LINE ( 'NONE', #84541, #60414 ) ;
#84106=DIRECTION ( 'NONE',  ( -0.000000000000000000, 0.000000000000000000, 1.000000000000000000 ) ) ;
#84139=ADVANCED_FACE ( 'NONE', ( #62479 ), #35020, .T. ) ;
#84168=VERTEX_POINT ( 'NONE', #1682 ) ;
#84171=ORIENTED_EDGE ( 'NONE', *, *, #81621, .F. ) ;
#84188=DIRECTION ( 'NONE',  ( 1.000000000000000000, 0.000000000000000000, 0.000000000000000000 ) ) ;
#84195=VERTEX_POINT ( 'NONE', #9333 ) ;
#84196=ORIENTED_EDGE ( 'NONE', *, *, #21548, .F. ) ;
#84212=DIRECTION ( 'NONE',  ( 0.000000000000000000, 0.000000000000000000, 1.000000000000000000 ) ) ;
#84223=CARTESIAN_POINT ( 'NONE',  ( 4.230769230769229061, -7.500000000000000000, 29.75000000000000355 ) ) ;
#84230=ORIENTED_EDGE ( 'NONE', *, *, #30968, .F. ) ;
#84247=ORIENTED_EDGE ( 'NONE', *, *, #47127, .T. ) ;
#84257=CARTESIAN_POINT ( 'NONE',  ( 11.25641025641025550, -11.00000000000000000, 29.75000000000000355 ) ) ;
#84285=LINE ( 'NONE', #77070, #73697 ) ;
#84310=CARTESIAN_POINT ( 'NONE',  ( 10.28846153846153832, -11.00000000000000000, 29.75000000000000355 ) ) ;
#84316=ORIENTED_EDGE ( 'NONE', *, *, #76269, .F. ) ;
#84322=LINE ( 'NONE', #22596, #61568 ) ;
#84328=DIRECTION ( 'NONE',  ( -1.000000000000000000, -0.000000000000000000, -0.000000000000000000 ) ) ;
#84332=FACE_OUTER_BOUND ( 'NONE', #76338, .T. ) ;
#84368=DIRECTION ( 'NONE',  ( 1.000000000000000000, 0.000000000000000000, 0.000000000000000000 ) ) ;
#84379=EDGE_CURVE ( 'NONE', #82422, #85209, #87828, .T. ) ;
#84384=CARTESIAN_POINT ( 'NONE',  ( -19.50000000000000000, -3.499999999999999556, 29.75000000000000355 ) ) ;
#84390=CYLINDRICAL_SURFACE ( 'NONE', #43582, 4.000000000000000000 ) ;
#84391=LINE ( 'NONE', #10041, #28302 ) ;
#84394=ORIENTED_EDGE ( 'NONE', *, *, #43390, .T. ) ;
#84407=EDGE_CURVE ( 'NONE', #4690, #23070, #52958, .T. ) ;
#84442=VERTEX_POINT ( 'NONE', #6562 ) ;
#84454=CARTESIAN_POINT ( 'NONE',  ( -0.6089743589743589203, -3.499999999999999556, 29.75000000000000355 ) ) ;
#84473=ORIENTED_EDGE ( 'NONE', *, *, #42263, .F. ) ;
#84474=DIRECTION ( 'NONE',  ( 1.000000000000000000, 0.000000000000000000, 0.000000000000000000 ) ) ;
#84506=VECTOR ( 'NONE', #27599, 1000.000000000000000 ) ;
#84530=EDGE_CURVE ( 'NONE', #67129, #64220, #41678, .T. ) ;
#84541=CARTESIAN_POINT ( 'NONE',  ( 13.19230769230769340, -11.50000000000000000, 29.75000000000000355 ) ) ;
#84545=CIRCLE ( 'NONE', #57143, 4.000000000000000000 ) ;
#84555=CARTESIAN_POINT ( 'NONE',  ( 13.19230769230769340, -7.500000000000000000, 29.75000000000000355 ) ) ;
#84590=ADVANCED_FACE ( 'NONE', ( #30374 ), #79004, .T. ) ;
#84601=ORIENTED_EDGE ( 'NONE', *, *, #70111, .T. ) ;
#84606=CIRCLE ( 'NONE', #6925, 4.000000000000000000 ) ;
#84607=DIRECTION ( 'NONE',  ( -1.000000000000000000, -0.000000000000000000, -0.000000000000000000 ) ) ;
#84616=VECTOR ( 'NONE', #75972, 1000.000000000000000 ) ;
#84632=EDGE_CURVE ( 'NONE', #29049, #26482, #43236, .T. ) ;
#84656=PLANE ( 'NONE',  #36994 ) ;
#84669=EDGE_LOOP ( 'NONE', ( #49819, #31541, #13843, #70508 ) ) ;
#84685=CARTESIAN_POINT ( 'NONE',  ( 17.78205128205128105, -3.499999999999999556, 29.75000000000000355 ) ) ;
#84687=ORIENTED_EDGE ( 'NONE', *, *, #48185, .T. ) ;
#84699=DIRECTION ( 'NONE',  ( 1.000000000000000000, 0.000000000000000000, 0.000000000000000000 ) ) ;
#84704=EDGE_CURVE ( 'NONE', #27134, #4346, #74038, .T. ) ;
#84714=CIRCLE ( 'NONE', #63079, 4.000000000000000000 ) ;
#84727=ORIENTED_EDGE ( 'NONE', *, *, #15028, .F. ) ;
#84728=CARTESIAN_POINT ( 'NONE',  ( -0.3589743589743593088, -3.499999999999999556, 29.75000000000000355 ) ) ;
#84732=ORIENTED_EDGE ( 'NONE', *, *, #73675, .F. ) ;
#84736=AXIS2_PLACEMENT_3D ( 'NONE', #74887, #40657, #13615 ) ;
#84755=ORIENTED_EDGE ( 'NONE', *, *, #50557, .T. ) ;
#84771=EDGE_CURVE ( 'NONE', #53967, #72293, #26725, .T. ) ;
#84774=ORIENTED_EDGE ( 'NONE', *, *, #86278, .F. ) ;
#84792=CARTESIAN_POINT ( 'NONE',  ( 7.384615384615385025, -11.00000000000000000, 29.75000000000000355 ) ) ;
#84793=CIRCLE ( 'NONE', #77636, 4.000000000000000000 ) ;
#84806=CIRCLE ( 'NONE', #68971, 4.000000000000000000 ) ;
#84809=VECTOR ( 'NONE', #88616, 1000.000000000000000 ) ;
#84818=DIRECTION ( 'NONE',  ( 1.000000000000000000, 0.000000000000000000, 0.000000000000000000 ) ) ;
#84829=CYLINDRICAL_SURFACE ( 'NONE', #88866, 4.000000000000000000 ) ;
#84839=DIRECTION ( 'NONE',  ( -0.000000000000000000, 1.000000000000000000, -0.000000000000000000 ) ) ;
#84866=LINE ( 'NONE', #16390, #2781 ) ;
#84869=EDGE_CURVE ( 'NONE', #4346, #31713, #68161, .T. ) ;
#84873=EDGE_CURVE ( 'NONE', #11880, #75229, #34365, .T. ) ;
#84875=VERTEX_POINT ( 'NONE', #6464 ) ;
#84876=CARTESIAN_POINT ( 'NONE',  ( -19.50000000000000000, -3.499999999999999556, 29.75000000000000355 ) ) ;
#84892=FACE_OUTER_BOUND ( 'NONE', #27916, .T. ) ;
#84895=DIRECTION ( 'NONE',  ( 1.000000000000000000, 0.000000000000000000, 0.000000000000000000 ) ) ;
#84910=LINE ( 'NONE', #706, #78863 ) ;
#84913=CARTESIAN_POINT ( 'NONE',  ( 19.50000000000000000, -7.500000000000000000, 29.75000000000000355 ) ) ;
#84920=ADVANCED_FACE ( 'NONE', ( #55084 ), #55525, .T. ) ;
#84948=EDGE_CURVE ( 'NONE', #7446, #49729, #21294, .T. ) ;
#84949=ORIENTED_EDGE ( 'NONE', *, *, #61964, .T. ) ;
#84953=CARTESIAN_POINT ( 'NONE',  ( -8.102564102564102200, -4.000000000000000000, 29.75000000000000355 ) ) ;
#84966=VECTOR ( 'NONE', #43815, 1000.000000000000000 ) ;
#84968=FACE_OUTER_BOUND ( 'NONE', #46120, .T. ) ;
#84970=ORIENTED_EDGE ( 'NONE', *, *, #33865, .F. ) ;
#84972=ORIENTED_EDGE ( 'NONE', *, *, #60288, .T. ) ;
#84979=CARTESIAN_POINT ( 'NONE',  ( 6.166666666666664298, -7.500000000000000000, 29.75000000000000355 ) ) ;
#84991=EDGE_CURVE ( 'NONE', #64401, #83471, #65705, .T. ) ;
#84994=EDGE_LOOP ( 'NONE', ( #78741, #26608, #53150, #16270 ) ) ;
#84999=ORIENTED_EDGE ( 'NONE', *, *, #7318, .T. ) ;
#85006=ADVANCED_FACE ( 'NONE', ( #39156 ), #18428, .F. ) ;
#85010=DIRECTION ( 'NONE',  ( 1.000000000000000000, 0.000000000000000000, 0.000000000000000000 ) ) ;
#85013=AXIS2_PLACEMENT_3D ( 'NONE', #47562, #88587, #61079 ) ;
#85016=ORIENTED_EDGE ( 'NONE', *, *, #88848, .T. ) ;
#85035=VERTEX_POINT ( 'NONE', #84792 ) ;
#85038=DIRECTION ( 'NONE',  ( -0.000000000000000000, 1.000000000000000000, -0.000000000000000000 ) ) ;
#85044=ORIENTED_EDGE ( 'NONE', *, *, #45385, .F. ) ;
#85054=VERTEX_POINT ( 'NONE', #59851 ) ;
#85065=LINE ( 'NONE', #52144, #28545 ) ;
#85073=ORIENTED_EDGE ( 'NONE', *, *, #8520, .F. ) ;
#85082=ORIENTED_EDGE ( 'NONE', *, *, #85121, .T. ) ;
#85090=CARTESIAN_POINT ( 'NONE',  ( 18.03205128205128105, -3.499999999999999556, 29.75000000000000355 ) ) ;
#85105=CARTESIAN_POINT ( 'NONE',  ( 16.81410256410256565, -7.500000000000000000, 29.75000000000000355 ) ) ;
#85110=CARTESIAN_POINT ( 'NONE',  ( 9.070512820512819374, -3.499999999999999556, 29.75000000000000355 ) ) ;
#85120=CARTESIAN_POINT ( 'NONE',  ( 9.320512820512821150, -3.499999999999999556, 29.75000000000000355 ) ) ;
#85121=EDGE_CURVE ( 'NONE', #63997, #38268, #62065, .T. ) ;
#85128=CARTESIAN_POINT ( 'NONE',  ( 9.320512820512821150, -11.00000000000000000, 29.75000000000000355 ) ) ;
#85129=ORIENTED_EDGE ( 'NONE', *, *, #86712, .T. ) ;
#85131=DIRECTION ( 'NONE',  ( 0.000000000000000000, 0.000000000000000000, -1.000000000000000000 ) ) ;
#85139=FACE_OUTER_BOUND ( 'NONE', #38660, .T. ) ;
#85155=LINE ( 'NONE', #57675, #82247 ) ;
#85156=CARTESIAN_POINT ( 'NONE',  ( -4.230769230769230838, -11.50000000000000000, 29.75000000000000355 ) ) ;
#85165=PLANE ( 'NONE',  #87455 ) ;
#85172=DIRECTION ( 'NONE',  ( -0.000000000000000000, 1.000000000000000000, -0.000000000000000000 ) ) ;
#85176=DIRECTION ( 'NONE',  ( 0.000000000000000000, 0.000000000000000000, -1.000000000000000000 ) ) ;
#85189=CARTESIAN_POINT ( 'NONE',  ( 6.416666666666664298, -3.499999999999999556, 29.75000000000000355 ) ) ;
#85191=AXIS2_PLACEMENT_3D ( 'NONE', #74704, #81465, #39596 ) ;
#85198=EDGE_CURVE ( 'NONE', #31226, #75640, #77747, .T. ) ;
#85209=VERTEX_POINT ( 'NONE', #42254 ) ;
#85211=DIRECTION ( 'NONE',  ( -0.000000000000000000, 1.000000000000000000, -0.000000000000000000 ) ) ;
#85217=CARTESIAN_POINT ( 'NONE',  ( 15.12820512820512953, -3.499999999999999556, 29.75000000000000355 ) ) ;
#85225=CIRCLE ( 'NONE', #23353, 4.000000000000000000 ) ;
#85228=ORIENTED_EDGE ( 'NONE', *, *, #35449, .F. ) ;
#85236=DIRECTION ( 'NONE',  ( 1.000000000000000000, 0.000000000000000000, 0.000000000000000000 ) ) ;
#85238=EDGE_CURVE ( 'NONE', #1493, #31713, #63390, .T. ) ;
#85265=LINE ( 'NONE', #56891, #24693 ) ;
#85269=VERTEX_POINT ( 'NONE', #23724 ) ;
#85276=FACE_OUTER_BOUND ( 'NONE', #81037, .T. ) ;
#85281=DIRECTION ( 'NONE',  ( -1.000000000000000000, -0.000000000000000000, -0.000000000000000000 ) ) ;
#85287=ORIENTED_EDGE ( 'NONE', *, *, #50256, .F. ) ;
#85290=CARTESIAN_POINT ( 'NONE',  ( 13.91025641025641235, -4.000000000000000000, 29.75000000000000355 ) ) ;
#85292=CARTESIAN_POINT ( 'NONE',  ( 16.81410256410256565, -7.500000000000000000, 29.75000000000000355 ) ) ;
#85299=ORIENTED_EDGE ( 'NONE', *, *, #26876, .T. ) ;
#85311=ORIENTED_EDGE ( 'NONE', *, *, #15271, .T. ) ;
#85352=ORIENTED_EDGE ( 'NONE', *, *, #68714, .T. ) ;
#85353=VECTOR ( 'NONE', #46561, 1000.000000000000000 ) ;
#85357=CARTESIAN_POINT ( 'NONE',  ( -10.03846153846153832, -3.499999999999999556, 29.75000000000000355 ) ) ;
#85379=CARTESIAN_POINT ( 'NONE',  ( 20.00000000000000000, -7.500000000000000000, 29.75000000000000355 ) ) ;
#85399=ADVANCED_FACE ( 'NONE', ( #67834 ), #74596, .T. ) ;
#85405=LINE ( 'NONE', #35894, #9173 ) ;
#85407=AXIS2_PLACEMENT_3D ( 'NONE', #56028, #22684, #42527 ) ;
#85416=ORIENTED_EDGE ( 'NONE', *, *, #21877, .F. ) ;
#85428=CARTESIAN_POINT ( 'NONE',  ( 7.134615384615385025, -4.000000000000000000, 29.75000000000000355 ) ) ;
#85437=LINE ( 'NONE', #77787, #60231 ) ;
#85439=DIRECTION ( 'NONE',  ( 0.000000000000000000, 0.000000000000000000, -1.000000000000000000 ) ) ;
#85447=DIRECTION ( 'NONE',  ( -0.000000000000000000, 1.000000000000000000, -0.000000000000000000 ) ) ;
#85467=VECTOR ( 'NONE', #63252, 1000.000000000000000 ) ;
#85505=EDGE_LOOP ( 'NONE', ( #15493, #48871, #66216, #18297 ) ) ;
#85529=VECTOR ( 'NONE', #19052, 1000.000000000000000 ) ;
#85530=FACE_OUTER_BOUND ( 'NONE', #3647, .T. ) ;
#85537=VERTEX_POINT ( 'NONE', #15554 ) ;
#85544=LINE ( 'NONE', #80009, #52378 ) ;
#85552=DIRECTION ( 'NONE',  ( -0.000000000000000000, 1.000000000000000000, -0.000000000000000000 ) ) ;
#85581=ORIENTED_EDGE ( 'NONE', *, *, #30593, .F. ) ;
#85582=FACE_OUTER_BOUND ( 'NONE', #69617, .T. ) ;
#85597=AXIS2_PLACEMENT_3D ( 'NONE', #5362, #53083, #32388 ) ;
#85602=CARTESIAN_POINT ( 'NONE',  ( -1.326923076923076872, -7.500000000000000000, 29.75000000000000355 ) ) ;
#85603=EDGE_LOOP ( 'NONE', ( #51089, #88401, #49034, #9032 ) ) ;
#85610=CARTESIAN_POINT ( 'NONE',  ( 10.03846153846153832, -11.00000000000000000, 28.25000000000000000 ) ) ;
#85614=EDGE_CURVE ( 'NONE', #5068, #7446, #40489, .T. ) ;
#85618=ORIENTED_EDGE ( 'NONE', *, *, #36958, .F. ) ;
#85624=CARTESIAN_POINT ( 'NONE',  ( 19.00000000000000000, -3.499999999999999556, 29.75000000000000355 ) ) ;
#85652=DIRECTION ( 'NONE',  ( 1.000000000000000000, 0.000000000000000000, 0.000000000000000000 ) ) ;
#85658=LINE ( 'NONE', #52303, #68804 ) ;
#85669=ORIENTED_EDGE ( 'NONE', *, *, #11489, .F. ) ;
#85677=ORIENTED_EDGE ( 'NONE', *, *, #7391, .F. ) ;
#85679=FACE_OUTER_BOUND ( 'NONE', #49737, .T. ) ;
#85680=ORIENTED_EDGE ( 'NONE', *, *, #72180, .F. ) ;
#85712=FACE_OUTER_BOUND ( 'NONE', #65677, .T. ) ;
#85726=VECTOR ( 'NONE', #27527, 1000.000000000000000 ) ;
#85733=DIRECTION ( 'NONE',  ( 0.000000000000000000, 0.000000000000000000, -1.000000000000000000 ) ) ;
#85742=ORIENTED_EDGE ( 'NONE', *, *, #14727, .T. ) ;
#85750=EDGE_CURVE ( 'NONE', #31128, #68727, #80378, .T. ) ;
#85751=VECTOR ( 'NONE', #42278, 1000.000000000000000 ) ;
#85758=ADVANCED_FACE ( 'NONE', ( #74951 ), #6486, .F. ) ;
#85774=ORIENTED_EDGE ( 'NONE', *, *, #35036, .F. ) ;
#85778=CARTESIAN_POINT ( 'NONE',  ( -18.75000000000000000, -7.500000000000000000, 33.75000000000000000 ) ) ;
#85779=VERTEX_POINT ( 'NONE', #82148 ) ;
#85794=CARTESIAN_POINT ( 'NONE',  ( 20.00000000000000000, -4.000000000000000000, 29.75000000000000355 ) ) ;
#85796=ADVANCED_FACE ( 'NONE', ( #83928 ), #75383, .T. ) ;
#85804=CARTESIAN_POINT ( 'NONE',  ( -6.416666666666667851, -7.500000000000000000, 29.75000000000000355 ) ) ;
#85811=EDGE_CURVE ( 'NONE', #18370, #49385, #47903, .T. ) ;
#85840=CARTESIAN_POINT ( 'NONE',  ( 20.00000000000000000, -4.000000000000000000, 29.75000000000000355 ) ) ;
#85844=ORIENTED_EDGE ( 'NONE', *, *, #40067, .F. ) ;
#85846=ORIENTED_EDGE ( 'NONE', *, *, #79106, .F. ) ;
#85880=AXIS2_PLACEMENT_3D ( 'NONE', #31623, #58191, #3692 ) ;
#85884=LINE ( 'NONE', #10668, #48364 ) ;
#85890=ADVANCED_FACE ( 'NONE', ( #29423 ), #86134, .F. ) ;
#85913=ADVANCED_FACE ( 'NONE', ( #78918 ), #30295, .F. ) ;
#85919=LINE ( 'NONE', #24202, #79118 ) ;
#85920=CIRCLE ( 'NONE', #39894, 4.000000000000000000 ) ;
#85924=ORIENTED_EDGE ( 'NONE', *, *, #60230, .F. ) ;
#85929=DIRECTION ( 'NONE',  ( 1.000000000000000000, 0.000000000000000000, 0.000000000000000000 ) ) ;
#85933=LINE ( 'NONE', #77399, #12632 ) ;
#85934=ORIENTED_EDGE ( 'NONE', *, *, #80306, .T. ) ;
#85938=EDGE_LOOP ( 'NONE', ( #4216, #3698, #3438, #49787 ) ) ;
#85943=VECTOR ( 'NONE', #86333, 1000.000000000000000 ) ;
#85952=EDGE_LOOP ( 'NONE', ( #16289, #65792, #22219, #80932 ) ) ;
#85953=CARTESIAN_POINT ( 'NONE',  ( 0.000000000000000000, -11.00000000000000000, 29.75000000000000355 ) ) ;
#85957=ORIENTED_EDGE ( 'NONE', *, *, #7551, .T. ) ;
#85963=ADVANCED_FACE ( 'NONE', ( #44673 ), #2362, .T. ) ;
#85982=VECTOR ( 'NONE', #58007, 1000.000000000000000 ) ;
#85986=EDGE_LOOP ( 'NONE', ( #38094, #46593, #31224, #79430, #52752 ) ) ;
#85991=PLANE ( 'NONE',  #12794 ) ;
#85994=DIRECTION ( 'NONE',  ( 0.000000000000000000, 0.000000000000000000, 1.000000000000000000 ) ) ;
#86047=EDGE_LOOP ( 'NONE', ( #30346, #61966, #84687, #53918 ) ) ;
#86057=CARTESIAN_POINT ( 'NONE',  ( -5.198717948717948012, -3.499999999999999556, 29.75000000000000355 ) ) ;
#86066=ORIENTED_EDGE ( 'NONE', *, *, #17958, .F. ) ;
#86073=ORIENTED_EDGE ( 'NONE', *, *, #23648, .T. ) ;
#86081=DIRECTION ( 'NONE',  ( -1.000000000000000000, -0.000000000000000000, -0.000000000000000000 ) ) ;
#86082=VECTOR ( 'NONE', #60392, 1000.000000000000000 ) ;
#86087=FACE_OUTER_BOUND ( 'NONE', #50633, .T. ) ;
#86092=LINE ( 'NONE', #3215, #18877 ) ;
#86094=LINE ( 'NONE', #58601, #61891 ) ;
#86131=CARTESIAN_POINT ( 'NONE',  ( 18.75000000000000000, -3.499999999999999556, 29.75000000000000355 ) ) ;
#86134=PLANE ( 'NONE',  #5958 ) ;
#86143=CIRCLE ( 'NONE', #64504, 4.000000000000000000 ) ;
#86146=ORIENTED_EDGE ( 'NONE', *, *, #66998, .T. ) ;
#86154=DIRECTION ( 'NONE',  ( 0.000000000000000000, 0.000000000000000000, -1.000000000000000000 ) ) ;
#86172=EDGE_LOOP ( 'NONE', ( #83422, #87205, #32327, #61559, #69803 ) ) ;
#86175=CARTESIAN_POINT ( 'NONE',  ( 20.00000000000000000, -4.000000000000000000, 29.75000000000000355 ) ) ;
#86183=AXIS2_PLACEMENT_3D ( 'NONE', #26621, #19862, #81575 ) ;
#86193=ADVANCED_FACE ( 'NONE', ( #48235 ), #75709, .F. ) ;
#86196=EDGE_LOOP ( 'NONE', ( #36899, #5989, #61241, #67887 ) ) ;
#86198=ORIENTED_EDGE ( 'NONE', *, *, #7318, .F. ) ;
#86199=ORIENTED_EDGE ( 'NONE', *, *, #73824, .T. ) ;
#86214=AXIS2_PLACEMENT_3D ( 'NONE', #25144, #45406, #51705 ) ;
#86223=ORIENTED_EDGE ( 'NONE', *, *, #76637, .T. ) ;
#86224=CARTESIAN_POINT ( 'NONE',  ( -11.97435897435897267, -7.500000000000000000, 29.75000000000000355 ) ) ;
#86237=ORIENTED_EDGE ( 'NONE', *, *, #59448, .F. ) ;
#86239=PLANE ( 'NONE',  #6771 ) ;
#86240=VERTEX_POINT ( 'NONE', #31058 ) ;
#86249=PLANE ( 'NONE',  #1450 ) ;
#86262=ADVANCED_FACE ( 'NONE', ( #50875 ), #23417, .T. ) ;
#86270=DIRECTION ( 'NONE',  ( 1.000000000000000000, 0.000000000000000000, 0.000000000000000000 ) ) ;
#86278=EDGE_CURVE ( 'NONE', #7880, #51834, #57215, .T. ) ;
#86290=CARTESIAN_POINT ( 'NONE',  ( 7.134615384615385025, -3.499999999999999556, 29.75000000000000355 ) ) ;
#86305=VERTEX_POINT ( 'NONE', #64842 ) ;
#86317=ORIENTED_EDGE ( 'NONE', *, *, #61175, .T. ) ;
#86331=ORIENTED_EDGE ( 'NONE', *, *, #19488, .F. ) ;
#86333=DIRECTION ( 'NONE',  ( -1.000000000000000000, -0.000000000000000000, -0.000000000000000000 ) ) ;
#86341=DIRECTION ( 'NONE',  ( -1.000000000000000000, 0.000000000000000000, -0.000000000000000000 ) ) ;
#86346=ORIENTED_EDGE ( 'NONE', *, *, #81435, .F. ) ;
#86362=EDGE_CURVE ( 'NONE', #10355, #33822, #17565, .T. ) ;
#86376=DIRECTION ( 'NONE',  ( -0.000000000000000000, 1.000000000000000000, -0.000000000000000000 ) ) ;
#86383=CARTESIAN_POINT ( 'NONE',  ( -6.166666666666667851, -3.499999999999999556, 29.75000000000000355 ) ) ;
#86391=CARTESIAN_POINT ( 'NONE',  ( -13.19230769230769340, -4.000000000000000000, 29.75000000000000355 ) ) ;
#86407=VECTOR ( 'NONE', #52789, 1000.000000000000000 ) ;
#86408=VECTOR ( 'NONE', #76572, 1000.000000000000000 ) ;
#86414=VECTOR ( 'NONE', #57835, 1000.000000000000000 ) ;
#86419=VERTEX_POINT ( 'NONE', #43566 ) ;
#86424=CARTESIAN_POINT ( 'NONE',  ( -19.50000000000000000, -3.499999999999999556, 29.75000000000000355 ) ) ;
#86438=CARTESIAN_POINT ( 'NONE',  ( 15.12820512820512953, -11.00000000000000000, 29.75000000000000355 ) ) ;
#86440=DIRECTION ( 'NONE',  ( 0.000000000000000000, 0.000000000000000000, 1.000000000000000000 ) ) ;
#86443=DIRECTION ( 'NONE',  ( 1.000000000000000000, 0.000000000000000000, 0.000000000000000000 ) ) ;
#86458=DIRECTION ( 'NONE',  ( -0.000000000000000000, 1.000000000000000000, -0.000000000000000000 ) ) ;
#86467=AXIS2_PLACEMENT_3D ( 'NONE', #30307, #56453, #70414 ) ;
#86468=AXIS2_PLACEMENT_3D ( 'NONE', #82349, #20630, #45672 ) ;
#86483=LINE ( 'NONE', #18454, #76863 ) ;
#86501=ORIENTED_EDGE ( 'NONE', *, *, #11928, .F. ) ;
#86505=ORIENTED_EDGE ( 'NONE', *, *, #39765, .T. ) ;
#86507=ORIENTED_EDGE ( 'NONE', *, *, #33357, .F. ) ;
#86511=EDGE_CURVE ( 'NONE', #13118, #17208, #8467, .T. ) ;
#86550=CARTESIAN_POINT ( 'NONE',  ( 4.230769230769229061, -7.500000000000000000, 33.75000000000000000 ) ) ;
#86555=VECTOR ( 'NONE', #62261, 1000.000000000000000 ) ;
#86558=FACE_OUTER_BOUND ( 'NONE', #39841, .T. ) ;
#86561=FACE_OUTER_BOUND ( 'NONE', #27481, .T. ) ;
#86573=ORIENTED_EDGE ( 'NONE', *, *, #77180, .F. ) ;
#86579=ORIENTED_EDGE ( 'NONE', *, *, #77670, .F. ) ;
#86587=FACE_OUTER_BOUND ( 'NONE', #26474, .T. ) ;
#86591=ORIENTED_EDGE ( 'NONE', *, *, #57052, .T. ) ;
#86601=LINE ( 'NONE', #25327, #82085 ) ;
#86616=EDGE_CURVE ( 'NONE', #63049, #18719, #71923, .T. ) ;
#86619=CYLINDRICAL_SURFACE ( 'NONE', #49866, 4.000000000000000000 ) ;
#86624=DIRECTION ( 'NONE',  ( 1.000000000000000000, 0.000000000000000000, 0.000000000000000000 ) ) ;
#86625=DIRECTION ( 'NONE',  ( 0.000000000000000000, 0.000000000000000000, -1.000000000000000000 ) ) ;
#86638=CYLINDRICAL_SURFACE ( 'NONE', #80133, 4.000000000000000000 ) ;
#86643=ORIENTED_EDGE ( 'NONE', *, *, #32185, .T. ) ;
#86665=VECTOR ( 'NONE', #32220, 1000.000000000000000 ) ;
#86681=CARTESIAN_POINT ( 'NONE',  ( 15.84615384615384670, -7.500000000000000000, 29.75000000000000355 ) ) ;
#86702=CARTESIAN_POINT ( 'NONE',  ( -0.3589743589743593088, -3.499999999999999556, 29.75000000000000355 ) ) ;
#86709=ADVANCED_FACE ( 'NONE', ( #61956 ), #27729, .F. ) ;
#86711=ORIENTED_EDGE ( 'NONE', *, *, #50806, .T. ) ;
#86712=EDGE_CURVE ( 'NONE', #81105, #71780, #67837, .T. ) ;
#86721=PLANE ( 'NONE',  #23095 ) ;
#86731=DIRECTION ( 'NONE',  ( 1.000000000000000000, 0.000000000000000000, 0.000000000000000000 ) ) ;
#86757=EDGE_CURVE ( 'NONE', #68522, #38776, #63731, .T. ) ;
#86789=EDGE_LOOP ( 'NONE', ( #2322, #29462, #25011, #13221 ) ) ;
#86796=CARTESIAN_POINT ( 'NONE',  ( -14.16025641025641058, -3.499999999999999556, 29.75000000000000355 ) ) ;
#86804=CARTESIAN_POINT ( 'NONE',  ( 11.97435897435897267, -3.499999999999999556, 29.75000000000000355 ) ) ;
#86805=DIRECTION ( 'NONE',  ( 0.000000000000000000, 0.000000000000000000, -1.000000000000000000 ) ) ;
#86809=EDGE_CURVE ( 'NONE', #26695, #5068, #84910, .T. ) ;
#86814=CARTESIAN_POINT ( 'NONE',  ( 16.09615384615384670, -3.499999999999999556, 29.75000000000000355 ) ) ;
#86816=CARTESIAN_POINT ( 'NONE',  ( 13.19230769230769340, -3.499999999999999556, 29.75000000000000355 ) ) ;
#86822=DIRECTION ( 'NONE',  ( 1.000000000000000000, 0.000000000000000000, 0.000000000000000000 ) ) ;
#86829=VECTOR ( 'NONE', #81313, 1000.000000000000000 ) ;
#86843=ORIENTED_EDGE ( 'NONE', *, *, #20827, .T. ) ;
#86856=ORIENTED_EDGE ( 'NONE', *, *, #14428, .F. ) ;
#86857=VECTOR ( 'NONE', #44691, 1000.000000000000000 ) ;
#86858=ORIENTED_EDGE ( 'NONE', *, *, #17783, .F. ) ;
#86861=DIRECTION ( 'NONE',  ( -0.000000000000000000, 1.000000000000000000, -0.000000000000000000 ) ) ;
#86868=DIRECTION ( 'NONE',  ( -0.000000000000000000, 1.000000000000000000, -0.000000000000000000 ) ) ;
#86883=ORIENTED_EDGE ( 'NONE', *, *, #4103, .F. ) ;
#86889=CARTESIAN_POINT ( 'NONE',  ( 19.50000000000000000, -3.499999999999999556, 29.75000000000000355 ) ) ;
#86892=FACE_OUTER_BOUND ( 'NONE', #82438, .T. ) ;
#86910=VECTOR ( 'NONE', #26702, 1000.000000000000000 ) ;
#86914=CARTESIAN_POINT ( 'NONE',  ( 17.78205128205128105, -3.499999999999999556, 29.75000000000000355 ) ) ;
#86915=SURFACE_STYLE_FILL_AREA ( #5522 ) ;
#86936=DIRECTION ( 'NONE',  ( 0.000000000000000000, 0.000000000000000000, -1.000000000000000000 ) ) ;
#86944=FACE_OUTER_BOUND ( 'NONE', #88608, .T. ) ;
#86948=LINE ( 'NONE', #38288, #47512 ) ;
#86968=EDGE_CURVE ( 'NONE', #27448, #60033, #70255, .T. ) ;
#86970=VERTEX_POINT ( 'NONE', #48227 ) ;
#86982=VECTOR ( 'NONE', #47619, 1000.000000000000000 ) ;
#87013=ORIENTED_EDGE ( 'NONE', *, *, #24551, .T. ) ;
#87052=VECTOR ( 'NONE', #78856, 1000.000000000000000 ) ;
#87067=EDGE_CURVE ( 'NONE', #48938, #82422, #13563, .T. ) ;
#87069=DIRECTION ( 'NONE',  ( 0.000000000000000000, 0.000000000000000000, 1.000000000000000000 ) ) ;
#87074=DIRECTION ( 'NONE',  ( 0.000000000000000000, 0.000000000000000000, -1.000000000000000000 ) ) ;
#87078=EDGE_LOOP ( 'NONE', ( #46413, #87092, #39748, #60506 ) ) ;
#87092=ORIENTED_EDGE ( 'NONE', *, *, #65454, .F. ) ;
#87096=CARTESIAN_POINT ( 'NONE',  ( -15.84615384615384670, -4.000000000000000000, 29.75000000000000355 ) ) ;
#87104=VERTEX_POINT ( 'NONE', #2248 ) ;
#87110=LINE ( 'NONE', #52847, #31897 ) ;
#87116=ORIENTED_EDGE ( 'NONE', *, *, #44833, .T. ) ;
#87125=CARTESIAN_POINT ( 'NONE',  ( 4.230769230769229061, -7.500000000000000000, 29.75000000000000355 ) ) ;
#87143=LINE ( 'NONE', #47010, #30201 ) ;
#87148=ORIENTED_EDGE ( 'NONE', *, *, #49926, .T. ) ;
#87174=EDGE_CURVE ( 'NONE', #235, #45953, #35754, .T. ) ;
#87187=DIRECTION ( 'NONE',  ( 0.000000000000000000, 0.000000000000000000, -1.000000000000000000 ) ) ;
#87189=AXIS2_PLACEMENT_3D ( 'NONE', #20988, #48459, #75945 ) ;
#87197=EDGE_CURVE ( 'NONE', #84168, #29224, #78355, .T. ) ;
#87205=ORIENTED_EDGE ( 'NONE', *, *, #76266, .F. ) ;
#87207=ORIENTED_EDGE ( 'NONE', *, *, #31768, .T. ) ;
#87211=VERTEX_POINT ( 'NONE', #84257 ) ;
#87221=DIRECTION ( 'NONE',  ( 0.000000000000000000, 0.000000000000000000, -1.000000000000000000 ) ) ;
#87244=CARTESIAN_POINT ( 'NONE',  ( 0.6089743589743582541, -3.499999999999999556, 29.75000000000000355 ) ) ;
#87253=DIRECTION ( 'NONE',  ( -1.000000000000000000, 0.000000000000000000, -0.000000000000000000 ) ) ;
#87286=CARTESIAN_POINT ( 'NONE',  ( 20.00000000000000000, -4.000000000000000000, 29.75000000000000355 ) ) ;
#87290=ORIENTED_EDGE ( 'NONE', *, *, #20273, .F. ) ;
#87297=VECTOR ( 'NONE', #81518, 1000.000000000000000 ) ;
#87305=ORIENTED_EDGE ( 'NONE', *, *, #12405, .F. ) ;
#87306=FACE_OUTER_BOUND ( 'NONE', #14642, .T. ) ;
#87313=EDGE_LOOP ( 'NONE', ( #59267, #33040, #11985, #67260 ) ) ;
#87314=ORIENTED_EDGE ( 'NONE', *, *, #56342, .T. ) ;
#87322=ADVANCED_FACE ( 'NONE', ( #20225 ), #83257, .F. ) ;
#87325=CARTESIAN_POINT ( 'NONE',  ( -19.50000000000000000, -11.50000000000000000, 29.75000000000000355 ) ) ;
#87334=FACE_OUTER_BOUND ( 'NONE', #12706, .T. ) ;
#87340=ORIENTED_EDGE ( 'NONE', *, *, #61453, .T. ) ;
#87341=LINE ( 'NONE', #53073, #49179 ) ;
#87397=ORIENTED_EDGE ( 'NONE', *, *, #88872, .F. ) ;
#87411=ORIENTED_EDGE ( 'NONE', *, *, #53523, .T. ) ;
#87423=VERTEX_POINT ( 'NONE', #82374 ) ;
#87427=ADVANCED_FACE ( 'NONE', ( #20658 ), #48123, .F. ) ;
#87446=CARTESIAN_POINT ( 'NONE',  ( 17.06410256410256565, -7.500000000000000000, 33.75000000000000000 ) ) ;
#87455=AXIS2_PLACEMENT_3D ( 'NONE', #77078, #64873, #22133 ) ;
#87461=VERTEX_POINT ( 'NONE', #50768 ) ;
#87471=FACE_OUTER_BOUND ( 'NONE', #499, .T. ) ;
#87473=CARTESIAN_POINT ( 'NONE',  ( -7.134615384615385025, -7.500000000000000000, 29.75000000000000355 ) ) ;
#87486=DIRECTION ( 'NONE',  ( -0.000000000000000000, 1.000000000000000000, -0.000000000000000000 ) ) ;
#87488=EDGE_CURVE ( 'NONE', #60033, #21562, #19979, .T. ) ;
#87503=DIRECTION ( 'NONE',  ( 1.000000000000000000, 0.000000000000000000, 0.000000000000000000 ) ) ;
#87513=CARTESIAN_POINT ( 'NONE',  ( -13.91025641025641235, -4.000000000000000000, 29.75000000000000355 ) ) ;
#87525=ORIENTED_EDGE ( 'NONE', *, *, #21707, .F. ) ;
#87533=DIRECTION ( 'NONE',  ( -1.000000000000000000, -0.000000000000000000, 0.000000000000000000 ) ) ;
#87551=ORIENTED_EDGE ( 'NONE', *, *, #36223, .F. ) ;
#87559=ADVANCED_FACE ( 'NONE', ( #58874 ), #80946, .T. ) ;
#87616=DIRECTION ( 'NONE',  ( -0.000000000000000000, 1.000000000000000000, -0.000000000000000000 ) ) ;
#87638=ORIENTED_EDGE ( 'NONE', *, *, #44492, .F. ) ;
#87649=EDGE_LOOP ( 'NONE', ( #44850, #79537, #41323, #24390 ) ) ;
#87656=CARTESIAN_POINT ( 'NONE',  ( -19.50000000000000000, -11.50000000000000000, 29.75000000000000355 ) ) ;
#87686=DIRECTION ( 'NONE',  ( -1.000000000000000000, -0.000000000000000000, 0.000000000000000000 ) ) ;
#87688=ORIENTED_EDGE ( 'NONE', *, *, #68229, .F. ) ;
#87691=VECTOR ( 'NONE', #45744, 1000.000000000000000 ) ;
#87692=DIRECTION ( 'NONE',  ( -1.000000000000000000, -0.000000000000000000, -0.000000000000000000 ) ) ;
#87706=VECTOR ( 'NONE', #74455, 1000.000000000000000 ) ;
#87714=EDGE_CURVE ( 'NONE', #30362, #6548, #54499, .T. ) ;
#87724=LINE ( 'NONE', #19246, #27008 ) ;
#87731=EDGE_CURVE ( 'NONE', #73366, #58603, #48457, .T. ) ;
#87739=ORIENTED_EDGE ( 'NONE', *, *, #75531, .F. ) ;
#87740=VECTOR ( 'NONE', #44114, 1000.000000000000000 ) ;
#87758=AXIS2_PLACEMENT_3D ( 'NONE', #49339, #76816, #15113 ) ;
#87760=EDGE_CURVE ( 'NONE', #4984, #87922, #6602, .T. ) ;
#87765=AXIS2_PLACEMENT_3D ( 'NONE', #67982, #26992, #66645 ) ;
#87766=ORIENTED_EDGE ( 'NONE', *, *, #40665, .F. ) ;
#87770=DIRECTION ( 'NONE',  ( -1.000000000000000000, -0.000000000000000000, -0.000000000000000000 ) ) ;
#87776=CARTESIAN_POINT ( 'NONE',  ( 19.50000000000000000, -4.000000000000000000, 29.75000000000000355 ) ) ;
#87789=EDGE_CURVE ( 'NONE', #1652, #11880, #55660, .T. ) ;
#87793=VERTEX_POINT ( 'NONE', #27752 ) ;
#87800=DIRECTION ( 'NONE',  ( -0.000000000000000000, 1.000000000000000000, -0.000000000000000000 ) ) ;
#87805=SURFACE_STYLE_USAGE ( .BOTH. , #80590 ) ;
#87814=DIRECTION ( 'NONE',  ( -0.000000000000000000, 1.000000000000000000, -0.000000000000000000 ) ) ;
#87824=LINE ( 'NONE', #39627, #49534 ) ;
#87828=CIRCLE ( 'NONE', #71971, 4.000000000000000000 ) ;
#87832=ADVANCED_FACE ( 'NONE', ( #83608 ), #77712, .F. ) ;
#87849=LINE ( 'NONE', #31986, #39975 ) ;
#87881=VERTEX_POINT ( 'NONE', #35397 ) ;
#87893=VECTOR ( 'NONE', #53641, 1000.000000000000000 ) ;
#87902=ORIENTED_EDGE ( 'NONE', *, *, #88083, .T. ) ;
#87915=DIRECTION ( 'NONE',  ( 1.000000000000000000, 0.000000000000000000, 0.000000000000000000 ) ) ;
#87922=VERTEX_POINT ( 'NONE', #56116 ) ;
#87924=EDGE_CURVE ( 'NONE', #32571, #73852, #76840, .T. ) ;
#87943=CIRCLE ( 'NONE', #18846, 4.000000000000000000 ) ;
#87951=ORIENTED_EDGE ( 'NONE', *, *, #68801, .T. ) ;
#87960=DIRECTION ( 'NONE',  ( 0.000000000000000000, 0.000000000000000000, -1.000000000000000000 ) ) ;
#87966=DIRECTION ( 'NONE',  ( -1.000000000000000000, -0.000000000000000000, -0.000000000000000000 ) ) ;
#87985=CARTESIAN_POINT ( 'NONE',  ( -3.262820512820514995, -11.50000000000000000, 29.75000000000000355 ) ) ;
#87986=FACE_OUTER_BOUND ( 'NONE', #16332, .T. ) ;
#88002=PLANE ( 'NONE',  #32194 ) ;
#88018=EDGE_LOOP ( 'NONE', ( #73325, #21735, #62162, #77604, #28946 ) ) ;
#88036=EDGE_CURVE ( 'NONE', #50542, #43102, #52456, .T. ) ;
#88065=CARTESIAN_POINT ( 'NONE',  ( -1.326923076923076872, -3.499999999999999556, 29.75000000000000355 ) ) ;
#88066=CARTESIAN_POINT ( 'NONE',  ( -14.87820512820512953, -7.500000000000000000, 29.75000000000000355 ) ) ;
#88073=ORIENTED_EDGE ( 'NONE', *, *, #30968, .T. ) ;
#88080=EDGE_CURVE ( 'NONE', #83231, #75643, #51707, .T. ) ;
#88083=EDGE_CURVE ( 'NONE', #30410, #64311, #6062, .T. ) ;
#88090=VECTOR ( 'NONE', #14782, 1000.000000000000000 ) ;
#88096=FACE_OUTER_BOUND ( 'NONE', #39247, .T. ) ;
#88097=VECTOR ( 'NONE', #50689, 1000.000000000000000 ) ;
#88098=ORIENTED_EDGE ( 'NONE', *, *, #34052, .F. ) ;
#88104=CARTESIAN_POINT ( 'NONE',  ( -19.50000000000000000, -3.499999999999999556, 29.75000000000000355 ) ) ;
#88119=LINE ( 'NONE', #61489, #67241 ) ;
#88123=LINE ( 'NONE', #6121, #4533 ) ;
#88147=LINE ( 'NONE', #40822, #83786 ) ;
#88166=VERTEX_POINT ( 'NONE', #6937 ) ;
#88197=ORIENTED_EDGE ( 'NONE', *, *, #49509, .T. ) ;
#88209=VERTEX_POINT ( 'NONE', #76275 ) ;
#88210=AXIS2_PLACEMENT_3D ( 'NONE', #28576, #55588, #49281 ) ;
#88216=CARTESIAN_POINT ( 'NONE',  ( -9.070512820512819374, -7.500000000000000000, 29.75000000000000355 ) ) ;
#88223=LINE ( 'NONE', #53960, #52818 ) ;
#88226=CARTESIAN_POINT ( 'NONE',  ( -16.09615384615384670, -3.499999999999999556, 29.75000000000000355 ) ) ;
#88265=CARTESIAN_POINT ( 'NONE',  ( 17.06410256410256565, -3.499999999999999556, 29.75000000000000355 ) ) ;
#88273=ORIENTED_EDGE ( 'NONE', *, *, #64633, .F. ) ;
#88277=AXIS2_PLACEMENT_3D ( 'NONE', #21122, #48591, #83734 ) ;
#88287=ORIENTED_EDGE ( 'NONE', *, *, #79661, .T. ) ;
#88293=DIRECTION ( 'NONE',  ( -1.000000000000000000, -0.000000000000000000, 0.000000000000000000 ) ) ;
#88297=EDGE_LOOP ( 'NONE', ( #64301, #40748, #33198, #77200, #24371 ) ) ;
#88299=ORIENTED_EDGE ( 'NONE', *, *, #18699, .T. ) ;
#88333=DIRECTION ( 'NONE',  ( -1.000000000000000000, -0.000000000000000000, -0.000000000000000000 ) ) ;
#88336=LINE ( 'NONE', #73475, #48910 ) ;
#88344=FACE_OUTER_BOUND ( 'NONE', #64551, .T. ) ;
#88353=ORIENTED_EDGE ( 'NONE', *, *, #1434, .T. ) ;
#88354=ORIENTED_EDGE ( 'NONE', *, *, #33972, .T. ) ;
#88358=CARTESIAN_POINT ( 'NONE',  ( 3.262820512820510999, -3.499999999999999556, 29.75000000000000355 ) ) ;
#88364=VECTOR ( 'NONE', #50433, 1000.000000000000000 ) ;
#88379=CARTESIAN_POINT ( 'NONE',  ( 7.384615384615385025, -3.499999999999999556, 29.75000000000000355 ) ) ;
#88396=EDGE_CURVE ( 'NONE', #87881, #19556, #52341, .T. ) ;
#88401=ORIENTED_EDGE ( 'NONE', *, *, #46037, .T. ) ;
#88437=ORIENTED_EDGE ( 'NONE', *, *, #79106, .T. ) ;
#88494=CARTESIAN_POINT ( 'NONE',  ( -4.230769230769230838, -3.499999999999999556, 29.75000000000000355 ) ) ;
#88501=CARTESIAN_POINT ( 'NONE',  ( 20.00000000000000000, -4.000000000000000000, 29.75000000000000355 ) ) ;
#88510=EDGE_CURVE ( 'NONE', #28699, #19429, #27549, .T. ) ;
#88518=ORIENTED_EDGE ( 'NONE', *, *, #41490, .T. ) ;
#88525=CIRCLE ( 'NONE', #10840, 4.000000000000000000 ) ;
#88531=ORIENTED_EDGE ( 'NONE', *, *, #35651, .T. ) ;
#88536=DIRECTION ( 'NONE',  ( 0.000000000000000000, 0.000000000000000000, -1.000000000000000000 ) ) ;
#88550=VERTEX_POINT ( 'NONE', #56350 ) ;
#88551=EDGE_CURVE ( 'NONE', #88209, #63997, #14927, .T. ) ;
#88561=CARTESIAN_POINT ( 'NONE',  ( -9.070512820512819374, -3.499999999999999556, 29.75000000000000355 ) ) ;
#88562=LINE ( 'NONE', #75032, #19135 ) ;
#88585=EDGE_CURVE ( 'NONE', #11346, #9623, #10268, .T. ) ;
#88587=DIRECTION ( 'NONE',  ( 1.000000000000000000, 0.000000000000000000, 0.000000000000000000 ) ) ;
#88608=EDGE_LOOP ( 'NONE', ( #59228, #46823, #81208, #15589, #34956 ) ) ;
#88616=DIRECTION ( 'NONE',  ( 1.000000000000000000, 0.000000000000000000, 0.000000000000000000 ) ) ;
#88621=VECTOR ( 'NONE', #54242, 1000.000000000000000 ) ;
#88628=ORIENTED_EDGE ( 'NONE', *, *, #15646, .F. ) ;
#88641=EDGE_LOOP ( 'NONE', ( #81769, #22402, #49387, #774 ) ) ;
#88645=LINE ( 'NONE', #48059, #27864 ) ;
#88647=EDGE_CURVE ( 'NONE', #5068, #58603, #18358, .T. ) ;
#88655=ORIENTED_EDGE ( 'NONE', *, *, #38780, .F. ) ;
#88667=DIRECTION ( 'NONE',  ( 1.000000000000000000, 0.000000000000000000, 0.000000000000000000 ) ) ;
#88668=DIRECTION ( 'NONE',  ( 0.000000000000000000, 0.000000000000000000, 1.000000000000000000 ) ) ;
#88673=( LENGTH_UNIT ( ) NAMED_UNIT ( * ) SI_UNIT ( .MILLI., .METRE. ) );
#88674=VERTEX_POINT ( 'NONE', #39084 ) ;
#88677=PRODUCT ( 'Dual Reciprocating Inner Cutter Blades', 'Dual Reciprocating Inner Cutter Blades', '', ( #52310 ) ) ;
#88700=LINE ( 'NONE', #73388, #74824 ) ;
#88707=VECTOR ( 'NONE', #24533, 1000.000000000000000 ) ;
#88712=FACE_OUTER_BOUND ( 'NONE', #80387, .T. ) ;
#88716=DIRECTION ( 'NONE',  ( 1.000000000000000000, 0.000000000000000000, 0.000000000000000000 ) ) ;
#88723=EDGE_LOOP ( 'NONE', ( #55653, #9854, #1428, #28765, #40693 ) ) ;
#88729=LINE ( 'NONE', #34201, #87297 ) ;
#88730=ORIENTED_EDGE ( 'NONE', *, *, #81621, .T. ) ;
#88737=CARTESIAN_POINT ( 'NONE',  ( 0.000000000000000000, -11.00000000000000000, 29.65000000000000213 ) ) ;
#88739=CARTESIAN_POINT ( 'NONE',  ( -16.81410256410256565, -11.50000000000000000, 29.75000000000000355 ) ) ;
#88741=EDGE_CURVE ( 'NONE', #76696, #20735, #72842, .T. ) ;
#88743=ADVANCED_FACE ( 'NONE', ( #26449 ), #52570, .F. ) ;
#88746=VECTOR ( 'NONE', #9262, 1000.000000000000000 ) ;
#88761=AXIS2_PLACEMENT_3D ( 'NONE', #62222, #27107, #26227 ) ;
#88766=VECTOR ( 'NONE', #13827, 1000.000000000000000 ) ;
#88774=VECTOR ( 'NONE', #8068, 1000.000000000000000 ) ;
#88784=DIRECTION ( 'NONE',  ( -1.000000000000000000, -0.000000000000000000, -0.000000000000000000 ) ) ;
#88786=VERTEX_POINT ( 'NONE', #66083 ) ;
#88791=EDGE_CURVE ( 'NONE', #60898, #18077, #80498, .T. ) ;
#88792=DIRECTION ( 'NONE',  ( 0.000000000000000000, 0.000000000000000000, -1.000000000000000000 ) ) ;
#88797=AXIS2_PLACEMENT_3D ( 'NONE', #73242, #25051, #79997 ) ;
#88803=LINE ( 'NONE', #34719, #23652 ) ;
#88829=CARTESIAN_POINT ( 'NONE',  ( 5.198717948717946236, -7.500000000000000000, 29.75000000000000355 ) ) ;
#88840=LINE ( 'NONE', #41970, #54375 ) ;
#88848=EDGE_CURVE ( 'NONE', #6322, #345, #47597, .T. ) ;
#88854=ORIENTED_EDGE ( 'NONE', *, *, #67995, .T. ) ;
#88866=AXIS2_PLACEMENT_3D ( 'NONE', #78932, #56886, #51429 ) ;
#88867=EDGE_CURVE ( 'NONE', #21562, #83716, #61109, .T. ) ;
#88872=EDGE_CURVE ( 'NONE', #72149, #40122, #45949, .T. ) ;
#88879=ORIENTED_EDGE ( 'NONE', *, *, #85614, .T. ) ;
#88890=DIRECTION ( 'NONE',  ( 0.000000000000000000, 0.000000000000000000, -1.000000000000000000 ) ) ;
#88913=CARTESIAN_POINT ( 'NONE',  ( 20.00000000000000000, -3.499999999999999556, 29.75000000000000355 ) ) ;
#88924=EDGE_CURVE ( 'NONE', #68522, #10355, #29117, .T. ) ;
#88926=ORIENTED_EDGE ( 'NONE', *, *, #22122, .F. ) ;
#88927=CARTESIAN_POINT ( 'NONE',  ( 10.28846153846153832, -7.500000000000000000, 29.75000000000000355 ) ) ;
#88928=ORIENTED_EDGE ( 'NONE', *, *, #39345, .F. ) ;
#88939=VECTOR ( 'NONE', #548, 1000.000000000000000 ) ;
#88947=VECTOR ( 'NONE', #50038, 1000.000000000000000 ) ;
#88950=ADVANCED_FACE ( 'NONE', ( #9708 ), #30428, .F. ) ;
#88973=EDGE_LOOP ( 'NONE', ( #61086, #45998, #36633, #54390 ) ) ;
#88980=LINE ( 'NONE', #27253, #69462 ) ;
#88985=AXIS2_PLACEMENT_3D ( 'NONE', #41316, #68784, #47628 ) ;
#89002=ADVANCED_FACE ( 'NONE', ( #19141 ), #11500, .F. ) ;
#89006=ORIENTED_EDGE ( 'NONE', *, *, #41100, .F. ) ;
#89019=EDGE_CURVE ( 'NONE', #51043, #84168, #3839, .T. ) ;
#89025=ORIENTED_EDGE ( 'NONE', *, *, #32979, .T. ) ;
#89037=DIRECTION ( 'NONE',  ( -0.000000000000000000, 0.000000000000000000, 1.000000000000000000 ) ) ;
#89063=AXIS2_PLACEMENT_3D ( 'NONE', #65043, #78126, #31279 ) ;
#89070=CARTESIAN_POINT ( 'NONE',  ( -8.352564102564102200, -3.499999999999999556, 29.75000000000000355 ) ) ;
#89074=EDGE_CURVE ( 'NONE', #46874, #80730, #34424, .T. ) ;
#89075=CARTESIAN_POINT ( 'NONE',  ( 18.03205128205128105, -3.499999999999999556, 29.75000000000000355 ) ) ;
#89094=DIRECTION ( 'NONE',  ( -0.000000000000000000, 1.000000000000000000, -0.000000000000000000 ) ) ;
#89107=CARTESIAN_POINT ( 'NONE',  ( 0.000000000000000000, -2.085786437626902856, 29.25000000000000000 ) ) ;
#89110=DIRECTION ( 'NONE',  ( -0.000000000000000000, 1.000000000000000000, -0.000000000000000000 ) ) ;
#89120=ORIENTED_EDGE ( 'NONE', *, *, #39345, .T. ) ;
#89132=ORIENTED_EDGE ( 'NONE', *, *, #30671, .T. ) ;
#89135=CARTESIAN_POINT ( 'NONE',  ( 15.84615384615384670, -3.499999999999999556, 29.75000000000000355 ) ) ;
#89157=PLANE ( 'NONE',  #37420 ) ;
#89164=ORIENTED_EDGE ( 'NONE', *, *, #88551, .T. ) ;
#89167=ORIENTED_EDGE ( 'NONE', *, *, #23479, .F. ) ;
#89171=VECTOR ( 'NONE', #88333, 1000.000000000000000 ) ;
ENDSEC;
END-ISO-10303-21;
